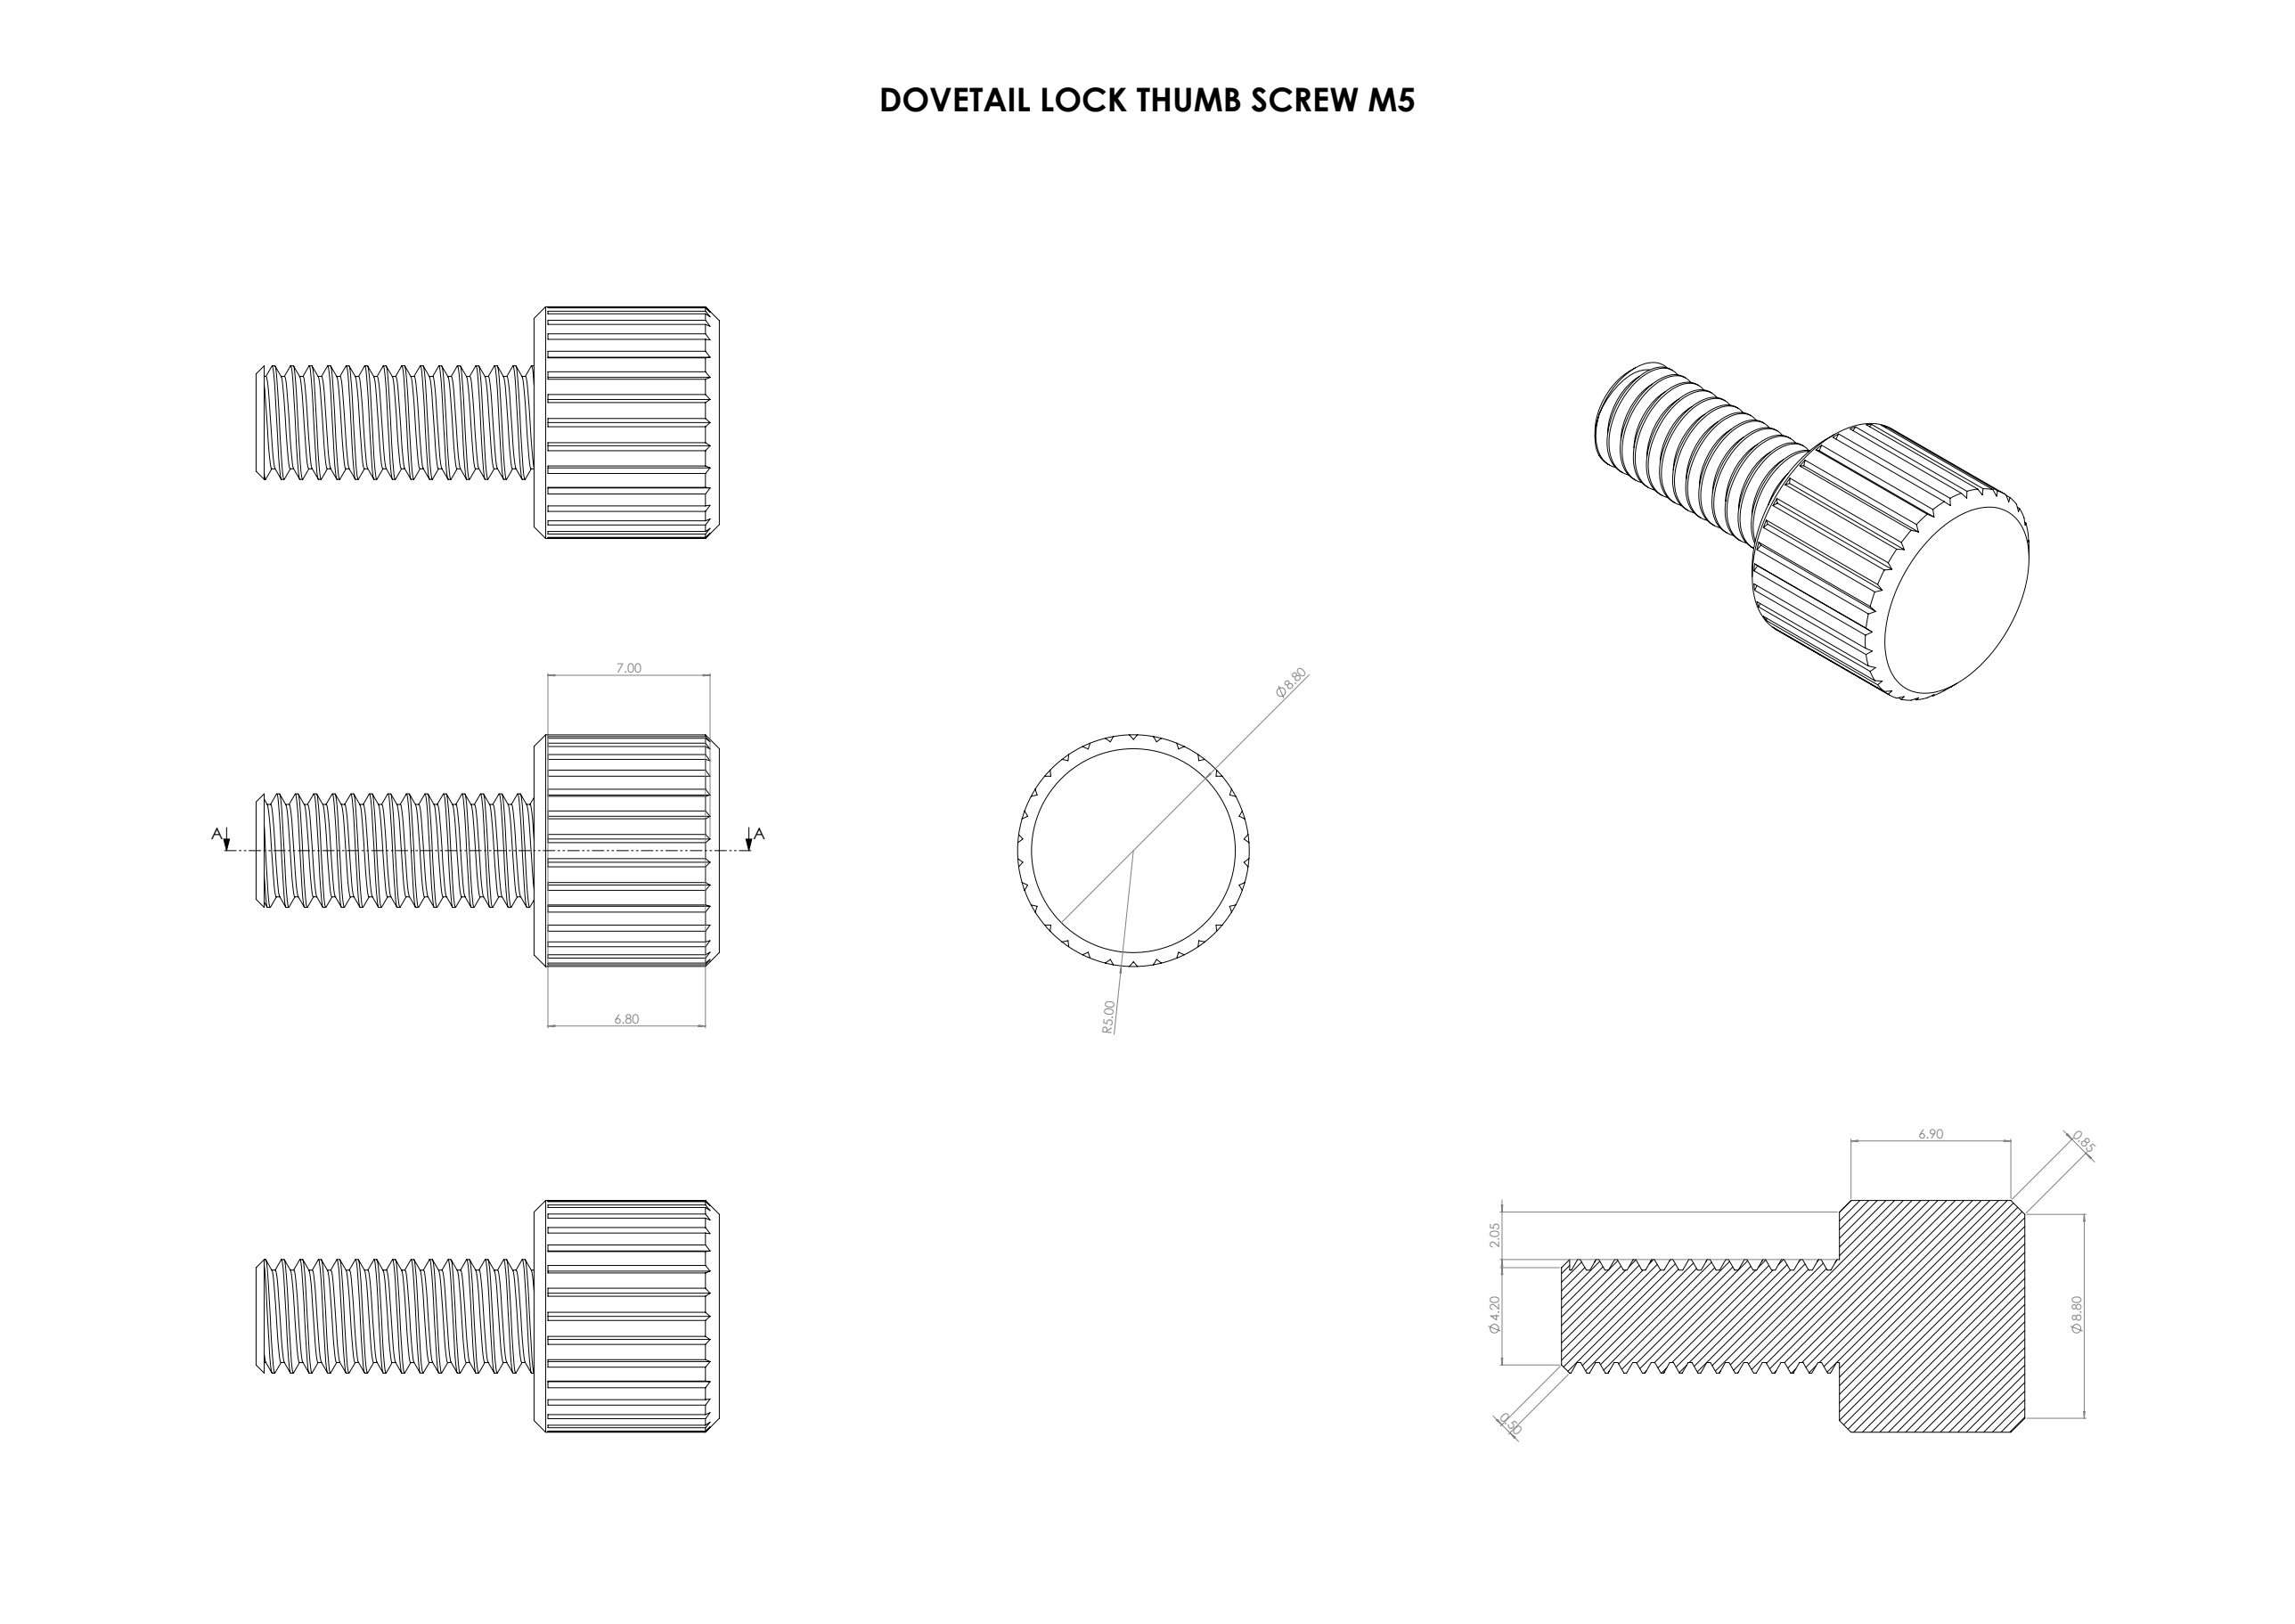
ISO-10303-21;
HEADER;
/* Generated by software containing ST-Developer
 * from STEP Tools, Inc. (www.steptools.com) 
 */

FILE_DESCRIPTION(
/* description */ (''),
/* implementation_level */ '2;1');

FILE_NAME(
/* name */ '12_Dovetail_Lock_Thumb_Screw_M5.step',
/* time_stamp */ '2026-10-21T02:03:06-07:00',
/* author */ (''),
/* organization */ (''),
/* preprocessor_version */ 'ST-DEVELOPER v20.2',
/* originating_system */ 'Autodesk Translation Framework v15.15.0.0',
/* authorisation */ '');

FILE_SCHEMA (('AUTOMOTIVE_DESIGN { 1 0 10303 214 3 1 1 }'));
ENDSEC;

DATA;
#10=MECHANICAL_DESIGN_GEOMETRIC_PRESENTATION_REPRESENTATION('',(#126),#38528);
#89=B_SPLINE_SURFACE_WITH_KNOTS('',3,3,((#36636,#36637,#36638,#36639,#36640,
#36641,#36642,#36643,#36644,#36645,#36646,#36647,#36648,#36649,#36650,#36651,
#36652,#36653,#36654,#36655,#36656,#36657,#36658,#36659,#36660,#36661,#36662,
#36663,#36664,#36665,#36666,#36667,#36668,#36669,#36670,#36671,#36672,#36673,
#36674,#36675,#36676,#36677,#36678,#36679,#36680,#36681,#36682,#36683,#36684,
#36685,#36686,#36687,#36688,#36689,#36690,#36691,#36692,#36693,#36694,#36695,
#36696,#36697,#36698,#36699,#36700,#36701,#36702,#36703,#36704,#36705,#36706,
#36707,#36708,#36709,#36710,#36711,#36712,#36713,#36714,#36715,#36716,#36717,
#36718,#36719,#36720,#36721,#36722,#36723,#36724,#36725,#36726,#36727,#36728,
#36729,#36730,#36731,#36732),(#36733,#36734,#36735,#36736,#36737,#36738,
#36739,#36740,#36741,#36742,#36743,#36744,#36745,#36746,#36747,#36748,#36749,
#36750,#36751,#36752,#36753,#36754,#36755,#36756,#36757,#36758,#36759,#36760,
#36761,#36762,#36763,#36764,#36765,#36766,#36767,#36768,#36769,#36770,#36771,
#36772,#36773,#36774,#36775,#36776,#36777,#36778,#36779,#36780,#36781,#36782,
#36783,#36784,#36785,#36786,#36787,#36788,#36789,#36790,#36791,#36792,#36793,
#36794,#36795,#36796,#36797,#36798,#36799,#36800,#36801,#36802,#36803,#36804,
#36805,#36806,#36807,#36808,#36809,#36810,#36811,#36812,#36813,#36814,#36815,
#36816,#36817,#36818,#36819,#36820,#36821,#36822,#36823,#36824,#36825,#36826,
#36827,#36828,#36829),(#36830,#36831,#36832,#36833,#36834,#36835,#36836,
#36837,#36838,#36839,#36840,#36841,#36842,#36843,#36844,#36845,#36846,#36847,
#36848,#36849,#36850,#36851,#36852,#36853,#36854,#36855,#36856,#36857,#36858,
#36859,#36860,#36861,#36862,#36863,#36864,#36865,#36866,#36867,#36868,#36869,
#36870,#36871,#36872,#36873,#36874,#36875,#36876,#36877,#36878,#36879,#36880,
#36881,#36882,#36883,#36884,#36885,#36886,#36887,#36888,#36889,#36890,#36891,
#36892,#36893,#36894,#36895,#36896,#36897,#36898,#36899,#36900,#36901,#36902,
#36903,#36904,#36905,#36906,#36907,#36908,#36909,#36910,#36911,#36912,#36913,
#36914,#36915,#36916,#36917,#36918,#36919,#36920,#36921,#36922,#36923,#36924,
#36925,#36926),(#36927,#36928,#36929,#36930,#36931,#36932,#36933,#36934,
#36935,#36936,#36937,#36938,#36939,#36940,#36941,#36942,#36943,#36944,#36945,
#36946,#36947,#36948,#36949,#36950,#36951,#36952,#36953,#36954,#36955,#36956,
#36957,#36958,#36959,#36960,#36961,#36962,#36963,#36964,#36965,#36966,#36967,
#36968,#36969,#36970,#36971,#36972,#36973,#36974,#36975,#36976,#36977,#36978,
#36979,#36980,#36981,#36982,#36983,#36984,#36985,#36986,#36987,#36988,#36989,
#36990,#36991,#36992,#36993,#36994,#36995,#36996,#36997,#36998,#36999,#37000,
#37001,#37002,#37003,#37004,#37005,#37006,#37007,#37008,#37009,#37010,#37011,
#37012,#37013,#37014,#37015,#37016,#37017,#37018,#37019,#37020,#37021,#37022,
#37023)),.UNSPECIFIED.,.F.,.F.,.F.,(4,4),(4,1,1,1,1,1,1,1,1,1,1,1,1,1,1,
1,1,1,1,1,1,1,1,1,1,1,1,1,1,1,1,1,1,1,1,1,1,1,1,1,1,1,1,1,1,1,1,1,1,1,1,
1,1,1,1,1,1,1,1,1,1,1,1,1,1,1,1,1,1,1,1,1,1,1,1,1,1,1,1,1,1,1,1,1,1,1,1,
1,1,1,1,1,1,1,4),(0.,0.0526254770366343),(8.30815772716261,9.30349343669038,
10.2988291462181,11.2941648557459,12.2895005652737,13.2848362748014,14.2801719843292,
15.275507693857,16.2708434033847,17.2661791129125,18.2615148224403,19.256850531968,
20.2521862414958,21.2475219510236,22.2428576605513,23.2381933700791,24.2335290796069,
25.2288647891346,26.2242004986624,27.2195362081902,28.2148719177179,29.2102076272457,
30.2055433367735,31.2008790463012,32.196214755829,33.1915504653568,34.1868861748845,
35.1822218844123,36.1775575939401,37.1728933034678,38.1682290129956,39.1635647225234,
40.1589004320511,41.1542361415789,42.1495718511067,43.1449075606344,44.1402432701622,
45.13557897969,46.1309146892177,47.1262503987455,48.1215861082733,49.116921817801,
50.1122575273288,51.1075932368566,52.1029289463843,53.0982646559121,54.0936003654399,
55.0889360749676,56.0842717844954,57.0796074940232,58.0749432035509,59.0702789130787,
60.0656146226065,61.0609503321342,62.056286041662,63.0516217511898,64.0469574607175,
65.0422931702453,66.0376288797731,67.0329645893008,68.0283002988286,69.0236360083564,
70.0189717178841,71.0143074274119,72.0096431369397,73.0049788464674,74.0003145559952,
74.995650265523,75.9909859750507,76.9863216845785,77.9816573941063,78.976993103634,
79.9723288131618,80.9676645226896,81.9630002322173,82.9583359417451,83.9536716512729,
84.9490073608006,85.9443430703284,86.9396787798562,87.9350144893839,88.9303501989117,
89.9256859084395,90.9210216179672,91.916357327495,92.9116930370228,93.9070287465505,
94.9023644560783,95.8977001656061,96.8930358751338,97.8883715846616,98.8837072941894,
99.8790430037171,100.874378713245,101.869714422773),.UNSPECIFIED.);
#90=B_SPLINE_SURFACE_WITH_KNOTS('',3,3,((#37321,#37322,#37323,#37324,#37325,
#37326,#37327,#37328,#37329,#37330,#37331,#37332,#37333,#37334,#37335,#37336,
#37337,#37338,#37339,#37340,#37341,#37342,#37343,#37344,#37345,#37346,#37347,
#37348,#37349,#37350,#37351,#37352,#37353,#37354,#37355,#37356,#37357,#37358,
#37359,#37360,#37361,#37362,#37363,#37364,#37365,#37366,#37367,#37368,#37369,
#37370,#37371,#37372,#37373,#37374,#37375,#37376,#37377,#37378,#37379,#37380,
#37381,#37382,#37383,#37384,#37385,#37386,#37387,#37388,#37389,#37390,#37391,
#37392,#37393,#37394,#37395,#37396,#37397,#37398,#37399,#37400,#37401,#37402,
#37403,#37404,#37405,#37406,#37407,#37408,#37409,#37410,#37411,#37412,#37413,
#37414,#37415,#37416,#37417),(#37418,#37419,#37420,#37421,#37422,#37423,
#37424,#37425,#37426,#37427,#37428,#37429,#37430,#37431,#37432,#37433,#37434,
#37435,#37436,#37437,#37438,#37439,#37440,#37441,#37442,#37443,#37444,#37445,
#37446,#37447,#37448,#37449,#37450,#37451,#37452,#37453,#37454,#37455,#37456,
#37457,#37458,#37459,#37460,#37461,#37462,#37463,#37464,#37465,#37466,#37467,
#37468,#37469,#37470,#37471,#37472,#37473,#37474,#37475,#37476,#37477,#37478,
#37479,#37480,#37481,#37482,#37483,#37484,#37485,#37486,#37487,#37488,#37489,
#37490,#37491,#37492,#37493,#37494,#37495,#37496,#37497,#37498,#37499,#37500,
#37501,#37502,#37503,#37504,#37505,#37506,#37507,#37508,#37509,#37510,#37511,
#37512,#37513,#37514),(#37515,#37516,#37517,#37518,#37519,#37520,#37521,
#37522,#37523,#37524,#37525,#37526,#37527,#37528,#37529,#37530,#37531,#37532,
#37533,#37534,#37535,#37536,#37537,#37538,#37539,#37540,#37541,#37542,#37543,
#37544,#37545,#37546,#37547,#37548,#37549,#37550,#37551,#37552,#37553,#37554,
#37555,#37556,#37557,#37558,#37559,#37560,#37561,#37562,#37563,#37564,#37565,
#37566,#37567,#37568,#37569,#37570,#37571,#37572,#37573,#37574,#37575,#37576,
#37577,#37578,#37579,#37580,#37581,#37582,#37583,#37584,#37585,#37586,#37587,
#37588,#37589,#37590,#37591,#37592,#37593,#37594,#37595,#37596,#37597,#37598,
#37599,#37600,#37601,#37602,#37603,#37604,#37605,#37606,#37607,#37608,#37609,
#37610,#37611),(#37612,#37613,#37614,#37615,#37616,#37617,#37618,#37619,
#37620,#37621,#37622,#37623,#37624,#37625,#37626,#37627,#37628,#37629,#37630,
#37631,#37632,#37633,#37634,#37635,#37636,#37637,#37638,#37639,#37640,#37641,
#37642,#37643,#37644,#37645,#37646,#37647,#37648,#37649,#37650,#37651,#37652,
#37653,#37654,#37655,#37656,#37657,#37658,#37659,#37660,#37661,#37662,#37663,
#37664,#37665,#37666,#37667,#37668,#37669,#37670,#37671,#37672,#37673,#37674,
#37675,#37676,#37677,#37678,#37679,#37680,#37681,#37682,#37683,#37684,#37685,
#37686,#37687,#37688,#37689,#37690,#37691,#37692,#37693,#37694,#37695,#37696,
#37697,#37698,#37699,#37700,#37701,#37702,#37703,#37704,#37705,#37706,#37707,
#37708)),.UNSPECIFIED.,.F.,.F.,.F.,(4,4),(4,1,1,1,1,1,1,1,1,1,1,1,1,1,1,
1,1,1,1,1,1,1,1,1,1,1,1,1,1,1,1,1,1,1,1,1,1,1,1,1,1,1,1,1,1,1,1,1,1,1,1,
1,1,1,1,1,1,1,1,1,1,1,1,1,1,1,1,1,1,1,1,1,1,1,1,1,1,1,1,1,1,1,1,1,1,1,1,
1,1,1,1,1,1,1,4),(0.,0.0526254770366343),(11.6163931973414,12.6117289068692,
13.6070646163969,14.6024003259247,15.5977360354525,16.5930717449802,17.588407454508,
18.5837431640358,19.5790788735635,20.5744145830913,21.5697502926191,22.5650860021468,
23.5604217116746,24.5557574212024,25.5510931307301,26.5464288402579,27.5417645497857,
28.5371002593134,29.5324359688412,30.527771678369,31.5231073878967,32.5184430974245,
33.5137788069523,34.50911451648,35.5044502260078,36.4997859355356,37.4951216450633,
38.4904573545911,39.4857930641189,40.4811287736466,41.4764644831744,42.4718001927022,
43.4671359022299,44.4624716117577,45.4578073212855,46.4531430308133,47.448478740341,
48.4438144498688,49.4391501593965,50.4344858689243,51.4298215784521,52.4251572879798,
53.4204929975076,54.4158287070354,55.4111644165631,56.4065001260909,57.4018358356187,
58.3971715451464,59.3925072546742,60.387842964202,61.3831786737297,62.3785143832575,
63.3738500927853,64.369185802313,65.3645215118408,66.3598572213686,67.3551929308963,
68.3505286404241,69.3458643499519,70.3412000594796,71.3365357690074,72.3318714785352,
73.3272071880629,74.3225428975907,75.3178786071185,76.3132143166462,77.308550026174,
78.3038857357018,79.2992214452295,80.2945571547573,81.2898928642851,82.2852285738128,
83.2805642833406,84.2758999928684,85.2712357023961,86.2665714119239,87.2619071214517,
88.2572428309794,89.2525785405072,90.247914250035,91.2432499595627,92.2385856690905,
93.2339213786183,94.229257088146,95.2245927976738,96.2199285072016,97.2152642167293,
98.2105999262571,99.2059356357849,100.201271345313,101.19660705484,102.191942764368,
103.187278473896,104.182614183424,105.177949892951),.UNSPECIFIED.);
#102=SHAPE_REPRESENTATION_RELATIONSHIP('SRR','None',#38587,#114);
#114=ADVANCED_BREP_SHAPE_REPRESENTATION('',(#138),#38527);
#126=STYLED_ITEM('',(#38713),#138);
#138=MANIFOLD_SOLID_BREP('Body1',#17083);
#396=CYLINDRICAL_SURFACE('',#18809,2.4505);
#397=CYLINDRICAL_SURFACE('',#18811,2.4505);
#398=CYLINDRICAL_SURFACE('',#18812,2.4505);
#399=CYLINDRICAL_SURFACE('',#18813,2.4505);
#400=CYLINDRICAL_SURFACE('',#18814,2.4505);
#401=CYLINDRICAL_SURFACE('',#18815,2.4505);
#402=CYLINDRICAL_SURFACE('',#18816,2.4505);
#403=CYLINDRICAL_SURFACE('',#18817,2.4505);
#404=CYLINDRICAL_SURFACE('',#18818,2.4505);
#405=CYLINDRICAL_SURFACE('',#18819,2.4505);
#406=CYLINDRICAL_SURFACE('',#18820,2.4505);
#407=CYLINDRICAL_SURFACE('',#18821,2.4505);
#408=CYLINDRICAL_SURFACE('',#18822,2.4505);
#409=CYLINDRICAL_SURFACE('',#18823,2.4505);
#410=CYLINDRICAL_SURFACE('',#18824,2.4505);
#411=CYLINDRICAL_SURFACE('',#18825,1.99475);
#412=CYLINDRICAL_SURFACE('',#18827,1.99475);
#413=CYLINDRICAL_SURFACE('',#18828,1.99475);
#414=CYLINDRICAL_SURFACE('',#18829,1.99475);
#415=CYLINDRICAL_SURFACE('',#18830,1.99475);
#416=CYLINDRICAL_SURFACE('',#18831,1.99475);
#417=CYLINDRICAL_SURFACE('',#18832,1.99475);
#418=CYLINDRICAL_SURFACE('',#18833,1.99475);
#419=CYLINDRICAL_SURFACE('',#18834,1.99475);
#420=CYLINDRICAL_SURFACE('',#18835,1.99475);
#421=CYLINDRICAL_SURFACE('',#18836,1.99475);
#422=CYLINDRICAL_SURFACE('',#18837,1.99475);
#423=CYLINDRICAL_SURFACE('',#18838,1.99475);
#424=CYLINDRICAL_SURFACE('',#18839,1.99475);
#425=CYLINDRICAL_SURFACE('',#18844,1.99475);
#426=CYLINDRICAL_SURFACE('',#18849,5.);
#427=CYLINDRICAL_SURFACE('',#19001,2.4505);
#781=B_SPLINE_CURVE_WITH_KNOTS('',3,(#35577,#35578,#35579,#35580,#35581,
#35582,#35583,#35584,#35585,#35586),.UNSPECIFIED.,.F.,.F.,(4,3,3,4),(-4.09157007060748,
-3.98134283811107,-2.9860071285833,-2.06659765062437),.UNSPECIFIED.);
#782=B_SPLINE_CURVE_WITH_KNOTS('',3,(#35589,#35590,#35591,#35592,#35593,
#35594,#35595),.UNSPECIFIED.,.F.,.F.,(4,3,4),(0.,0.995335709527768,1.1166202336066),
 .UNSPECIFIED.);
#783=B_SPLINE_CURVE_WITH_KNOTS('',3,(#35600,#35601,#35602,#35603,#35604,
#35605,#35606,#35607,#35608,#35609,#35610,#35611,#35612,#35613,#35614,#35615,
#35616,#35617,#35618,#35619,#35620,#35621),.UNSPECIFIED.,.F.,.F.,(4,3,3,
3,3,3,3,4),(-10.3747553777871,-9.95335709527767,-8.9580213857499,-7.96268567622213,
-6.96734996669437,-5.9720142571666,-4.97667854763883,-4.09157007060748),
 .UNSPECIFIED.);
#784=B_SPLINE_CURVE_WITH_KNOTS('',3,(#35622,#35623,#35624,#35625,#35626,
#35627,#35628,#35629,#35630,#35631,#35632,#35633,#35634,#35635,#35636,#35637,
#35638,#35639,#35640,#35641,#35642,#35643),.UNSPECIFIED.,.F.,.F.,(4,3,3,
3,3,3,3,4),(1.1166202336066,1.99067141905553,2.9860071285833,3.98134283811107,
4.97667854763883,5.9720142571666,6.96734996669436,7.39980554078619),
 .UNSPECIFIED.);
#785=B_SPLINE_CURVE_WITH_KNOTS('',3,(#35648,#35649,#35650,#35651,#35652,
#35653,#35654,#35655,#35656,#35657,#35658,#35659,#35660,#35661,#35662,#35663,
#35664,#35665,#35666,#35667,#35668,#35669),.UNSPECIFIED.,.F.,.F.,(4,3,3,
3,3,3,3,4),(-16.6579406849666,-15.9253713524443,-14.9300356429165,-13.9346999333887,
-12.939364223861,-11.9440285143332,-10.9486928048054,-10.3747553777871),
 .UNSPECIFIED.);
#786=B_SPLINE_CURVE_WITH_KNOTS('',3,(#35670,#35671,#35672,#35673,#35674,
#35675,#35676,#35677,#35678,#35679,#35680,#35681,#35682,#35683,#35684,#35685,
#35686,#35687,#35688,#35689,#35690,#35691),.UNSPECIFIED.,.F.,.F.,(4,3,3,
3,3,3,3,4),(7.39980554078619,7.96268567622213,8.9580213857499,9.95335709527766,
10.9486928048054,11.9440285143332,12.939364223861,13.6829908479658),
 .UNSPECIFIED.);
#787=B_SPLINE_CURVE_WITH_KNOTS('',3,(#35696,#35697,#35698,#35699,#35700,
#35701,#35702,#35703,#35704,#35705,#35706,#35707,#35708,#35709,#35710,#35711,
#35712,#35713,#35714,#35715,#35716,#35717,#35718,#35719,#35720),
 .UNSPECIFIED.,.F.,.F.,(4,3,3,3,3,3,3,3,4),(-22.9411259921462,-22.8927213191386,
-21.8973856096109,-20.9020499000831,-19.9067141905553,-18.9113784810276,
-17.9160427714998,-16.920707061972,-16.6579406849666),.UNSPECIFIED.);
#788=B_SPLINE_CURVE_WITH_KNOTS('',3,(#35721,#35722,#35723,#35724,#35725,
#35726,#35727,#35728,#35729,#35730,#35731,#35732,#35733,#35734,#35735,#35736,
#35737,#35738,#35739,#35740,#35741,#35742,#35743,#35744,#35745),
 .UNSPECIFIED.,.F.,.F.,(4,3,3,3,3,3,3,3,4),(13.6829908479658,13.9346999333887,
14.9300356429165,15.9253713524443,16.920707061972,17.9160427714998,18.9113784810276,
19.9067141905553,19.9661761551454),.UNSPECIFIED.);
#789=B_SPLINE_CURVE_WITH_KNOTS('',3,(#35750,#35751,#35752,#35753,#35754,
#35755,#35756,#35757,#35758,#35759,#35760,#35761,#35762,#35763,#35764,#35765,
#35766,#35767,#35768,#35769,#35770,#35771),.UNSPECIFIED.,.F.,.F.,(4,3,3,
3,3,3,3,4),(-29.2243112993258,-28.8647355763052,-27.8693998667775,-26.8740641572497,
-25.8787284477219,-24.8833927381942,-23.8880570286664,-22.9411259921462),
 .UNSPECIFIED.);
#790=B_SPLINE_CURVE_WITH_KNOTS('',3,(#35772,#35773,#35774,#35775,#35776,
#35777,#35778,#35779,#35780,#35781,#35782,#35783,#35784,#35785,#35786,#35787,
#35788,#35789,#35790,#35791,#35792,#35793),.UNSPECIFIED.,.F.,.F.,(4,3,3,
3,3,3,3,4),(19.9661761551454,20.9020499000831,21.8973856096109,22.8927213191386,
23.8880570286664,24.8833927381942,25.8787284477219,26.2493614623249),
 .UNSPECIFIED.);
#791=B_SPLINE_CURVE_WITH_KNOTS('',3,(#35798,#35799,#35800,#35801,#35802,
#35803,#35804,#35805,#35806,#35807,#35808,#35809,#35810,#35811,#35812,#35813,
#35814,#35815,#35816,#35817,#35818,#35819),.UNSPECIFIED.,.F.,.F.,(4,3,3,
3,3,3,3,4),(-35.5074966065054,-34.8367498334718,-33.8414141239441,-32.8460784144163,
-31.8507427048885,-30.8554069953608,-29.860071285833,-29.2243112993258),
 .UNSPECIFIED.);
#792=B_SPLINE_CURVE_WITH_KNOTS('',3,(#35820,#35821,#35822,#35823,#35824,
#35825,#35826,#35827,#35828,#35829,#35830,#35831,#35832,#35833,#35834,#35835,
#35836,#35837,#35838,#35839,#35840,#35841),.UNSPECIFIED.,.F.,.F.,(4,3,3,
3,3,3,3,4),(26.2493614623249,26.8740641572497,27.8693998667775,28.8647355763052,
29.860071285833,30.8554069953608,31.8507427048885,32.5325467695045),
 .UNSPECIFIED.);
#793=B_SPLINE_CURVE_WITH_KNOTS('',3,(#35846,#35847,#35848,#35849,#35850,
#35851,#35852,#35853,#35854,#35855,#35856,#35857,#35858,#35859,#35860,#35861,
#35862,#35863,#35864,#35865,#35866,#35867),.UNSPECIFIED.,.F.,.F.,(4,3,3,
3,3,3,3,4),(-41.790681913685,-40.8087640906384,-39.8134283811107,-38.8180926715829,
-37.8227569620551,-36.8274212525274,-35.8320855429996,-35.5074966065054),
 .UNSPECIFIED.);
#794=B_SPLINE_CURVE_WITH_KNOTS('',3,(#35868,#35869,#35870,#35871,#35872,
#35873,#35874,#35875,#35876,#35877,#35878,#35879,#35880,#35881,#35882,#35883,
#35884,#35885,#35886,#35887,#35888,#35889),.UNSPECIFIED.,.F.,.F.,(4,3,3,
3,3,3,3,4),(32.5325467695045,32.8460784144163,33.8414141239441,34.8367498334718,
35.8320855429996,36.8274212525274,37.8227569620551,38.8157320766841),
 .UNSPECIFIED.);
#795=B_SPLINE_CURVE_WITH_KNOTS('',3,(#35894,#35895,#35896,#35897,#35898,
#35899,#35900,#35901,#35902,#35903,#35904,#35905,#35906,#35907,#35908,#35909,
#35910,#35911,#35912,#35913,#35914,#35915,#35916,#35917,#35918),
 .UNSPECIFIED.,.F.,.F.,(4,3,3,3,3,3,3,3,4),(-48.0738672208646,-47.7761140573328,
-46.780778347805,-45.7854426382773,-44.7901069287495,-43.7947712192217,
-42.799435509694,-41.8040998001662,-41.790681913685),.UNSPECIFIED.);
#796=B_SPLINE_CURVE_WITH_KNOTS('',3,(#35919,#35920,#35921,#35922,#35923,
#35924,#35925,#35926,#35927,#35928,#35929,#35930,#35931,#35932,#35933,#35934,
#35935,#35936,#35937,#35938,#35939,#35940,#35941,#35942,#35943),
 .UNSPECIFIED.,.F.,.F.,(4,3,3,3,3,3,3,3,4),(38.8157320766841,38.8180926715829,
39.8134283811107,40.8087640906384,41.8040998001662,42.799435509694,43.7947712192217,
44.7901069287495,45.0989173838637),.UNSPECIFIED.);
#797=B_SPLINE_CURVE_WITH_KNOTS('',3,(#35948,#35949,#35950,#35951,#35952,
#35953,#35954,#35955,#35956,#35957,#35958,#35959,#35960,#35961,#35962,#35963,
#35964,#35965,#35966,#35967,#35968,#35969),.UNSPECIFIED.,.F.,.F.,(4,3,3,
3,3,3,3,4),(-54.3570525280442,-53.7481283144994,-52.7527926049716,-51.7574568954439,
-50.7621211859161,-49.7667854763883,-48.7714497668606,-48.0738672208646),
 .UNSPECIFIED.);
#798=B_SPLINE_CURVE_WITH_KNOTS('',3,(#35970,#35971,#35972,#35973,#35974,
#35975,#35976,#35977,#35978,#35979,#35980,#35981,#35982,#35983,#35984,#35985,
#35986,#35987,#35988,#35989,#35990,#35991),.UNSPECIFIED.,.F.,.F.,(4,3,3,
3,3,3,3,4),(45.0989173838637,45.7854426382773,46.780778347805,47.7761140573328,
48.7714497668606,49.7667854763883,50.7621211859161,51.3821026910433),
 .UNSPECIFIED.);
#799=B_SPLINE_CURVE_WITH_KNOTS('',3,(#35996,#35997,#35998,#35999,#36000,
#36001,#36002,#36003,#36004,#36005,#36006,#36007,#36008,#36009,#36010,#36011,
#36012,#36013,#36014,#36015,#36016,#36017),.UNSPECIFIED.,.F.,.F.,(4,3,3,
3,3,3,3,4),(-60.6402378352238,-59.720142571666,-58.7248068621382,-57.7294711526105,
-56.7341354430827,-55.7387997335549,-54.7434640240272,-54.3570525280442),
 .UNSPECIFIED.);
#800=B_SPLINE_CURVE_WITH_KNOTS('',3,(#36018,#36019,#36020,#36021,#36022,
#36023,#36024,#36025,#36026,#36027,#36028,#36029,#36030,#36031,#36032,#36033,
#36034,#36035,#36036,#36037,#36038,#36039),.UNSPECIFIED.,.F.,.F.,(4,3,3,
3,3,3,3,4),(51.3821026910433,51.7574568954439,52.7527926049716,53.7481283144994,
54.7434640240272,55.7387997335549,56.7341354430827,57.6652879982229),
 .UNSPECIFIED.);
#801=B_SPLINE_CURVE_WITH_KNOTS('',3,(#36044,#36045,#36046,#36047,#36048,
#36049,#36050,#36051,#36052,#36053,#36054,#36055,#36056,#36057,#36058,#36059,
#36060,#36061,#36062,#36063,#36064,#36065,#36066,#36067,#36068),
 .UNSPECIFIED.,.F.,.F.,(4,3,3,3,3,3,3,3,4),(-66.9234231424034,-66.6874925383604,
-65.6921568288326,-64.6968211193048,-63.7014854097771,-62.7061497002493,
-61.7108139907215,-60.7154782811938,-60.6402378352238),.UNSPECIFIED.);
#802=B_SPLINE_CURVE_WITH_KNOTS('',3,(#36069,#36070,#36071,#36072,#36073,
#36074,#36075,#36076,#36077,#36078,#36079,#36080,#36081,#36082,#36083,#36084,
#36085,#36086,#36087,#36088,#36089,#36090,#36091,#36092,#36093),
 .UNSPECIFIED.,.F.,.F.,(4,3,3,3,3,3,3,3,4),(57.6652879982229,57.7294711526105,
58.7248068621382,59.720142571666,60.7154782811938,61.7108139907215,62.7061497002493,
63.7014854097771,63.9484733054025),.UNSPECIFIED.);
#803=B_SPLINE_CURVE_WITH_KNOTS('',3,(#36098,#36099,#36100,#36101,#36102,
#36103,#36104,#36105,#36106,#36107,#36108,#36109,#36110,#36111,#36112,#36113,
#36114,#36115,#36116,#36117,#36118,#36119),.UNSPECIFIED.,.F.,.F.,(4,3,3,
3,3,3,3,4),(-73.206608449583,-72.659506795527,-71.6641710859992,-70.6688353764714,
-69.6734996669437,-68.6781639574159,-67.6828282478881,-66.9234231424034),
 .UNSPECIFIED.);
#804=B_SPLINE_CURVE_WITH_KNOTS('',3,(#36120,#36121,#36122,#36123,#36124,
#36125,#36126,#36127,#36128,#36129,#36130,#36131,#36132,#36133,#36134,#36135,
#36136,#36137,#36138,#36139,#36140,#36141),.UNSPECIFIED.,.F.,.F.,(4,3,3,
3,3,3,3,4),(63.9484733054025,64.6968211193048,65.6921568288326,66.6874925383604,
67.6828282478881,68.6781639574159,69.6734996669437,70.2316586125821),
 .UNSPECIFIED.);
#805=B_SPLINE_CURVE_WITH_KNOTS('',3,(#36146,#36147,#36148,#36149,#36150,
#36151,#36152,#36153,#36154,#36155,#36156,#36157,#36158,#36159,#36160,#36161,
#36162,#36163,#36164,#36165,#36166,#36167),.UNSPECIFIED.,.F.,.F.,(4,3,3,
3,3,3,3,4),(-79.4897937567626,-78.6315210526936,-77.6361853431658,-76.640849633638,
-75.6455139241102,-74.6501782145825,-73.6548425050547,-73.206608449583),
 .UNSPECIFIED.);
#806=B_SPLINE_CURVE_WITH_KNOTS('',3,(#36168,#36169,#36170,#36171,#36172,
#36173,#36174,#36175,#36176,#36177,#36178,#36179,#36180,#36181,#36182,#36183,
#36184,#36185,#36186,#36187,#36188,#36189),.UNSPECIFIED.,.F.,.F.,(4,3,3,
3,3,3,3,4),(70.2316586125821,70.6688353764714,71.6641710859992,72.659506795527,
73.6548425050547,74.6501782145825,75.6455139241103,76.5148439197617),
 .UNSPECIFIED.);
#807=B_SPLINE_CURVE_WITH_KNOTS('',3,(#36194,#36195,#36196,#36197,#36198,
#36199,#36200,#36201,#36202,#36203,#36204,#36205,#36206,#36207,#36208,#36209,
#36210,#36211,#36212,#36213,#36214,#36215,#36216,#36217,#36218),
 .UNSPECIFIED.,.F.,.F.,(4,3,3,3,3,3,3,3,4),(-85.7729790639422,-85.5988710193879,
-84.6035353098602,-83.6081996003324,-82.6128638908046,-81.6175281812769,
-80.6221924717491,-79.6268567622213,-79.4897937567626),.UNSPECIFIED.);
#808=B_SPLINE_CURVE_WITH_KNOTS('',3,(#36219,#36220,#36221,#36222,#36223,
#36224,#36225,#36226,#36227,#36228,#36229,#36230,#36231,#36232,#36233,#36234,
#36235,#36236,#36237,#36238,#36239,#36240,#36241,#36242,#36243),
 .UNSPECIFIED.,.F.,.F.,(4,3,3,3,3,3,3,3,4),(76.5148439197617,76.640849633638,
77.6361853431658,78.6315210526936,79.6268567622213,80.6221924717491,81.6175281812769,
82.6128638908046,82.7980292269413),.UNSPECIFIED.);
#809=B_SPLINE_CURVE_WITH_KNOTS('',3,(#36248,#36249,#36250,#36251,#36252,
#36253,#36254,#36255,#36256,#36257,#36258,#36259,#36260,#36261,#36262,#36263,
#36264,#36265,#36266,#36267,#36268,#36269),.UNSPECIFIED.,.F.,.F.,(4,3,3,
3,3,3,3,4),(-92.0561643711218,-91.5708852765545,-90.5755495670268,-89.580213857499,
-88.5848781479712,-87.5895424384435,-86.5942067289157,-85.7729790639422),
 .UNSPECIFIED.);
#810=B_SPLINE_CURVE_WITH_KNOTS('',3,(#36270,#36271,#36272,#36273,#36274,
#36275,#36276,#36277,#36278,#36279,#36280,#36281,#36282,#36283,#36284,#36285,
#36286,#36287,#36288,#36289,#36290,#36291),.UNSPECIFIED.,.F.,.F.,(4,3,3,
3,3,3,3,4),(82.7980292269413,83.6081996003324,84.6035353098601,85.5988710193879,
86.5942067289157,87.5895424384435,88.5848781479712,89.0812145341209),
 .UNSPECIFIED.);
#811=B_SPLINE_CURVE_WITH_KNOTS('',3,(#36297,#36298,#36299,#36300,#36301,
#36302,#36303,#36304,#36305),.UNSPECIFIED.,.F.,.F.,(4,1,1,1,1,1,4),(97.3893722612836,
98.2105999262571,99.2059356357849,100.201271345313,101.19660705484,102.191942764368,
103.111352242327),.UNSPECIFIED.);
#812=B_SPLINE_CURVE_WITH_KNOTS('',3,(#36308,#36309,#36310,#36311,#36312,
#36313,#36314,#36315),.UNSPECIFIED.,.F.,.F.,(4,1,1,1,1,4),(97.3893722612836,
97.8883715846616,98.8837072941894,99.8790430037171,100.874378713245,101.869714422773),
 .UNSPECIFIED.);
#813=B_SPLINE_CURVE_WITH_KNOTS('',3,(#36320,#36321,#36322,#36323,#36324,
#36325,#36326,#36327,#36328,#36329,#36330),.UNSPECIFIED.,.F.,.F.,(4,1,1,
1,1,1,1,1,4),(91.106186954104,91.2432499595627,92.2385856690905,93.2339213786183,
94.229257088146,95.2245927976738,96.2199285072016,97.2152642167293,97.3893722612836),
 .UNSPECIFIED.);
#814=B_SPLINE_CURVE_WITH_KNOTS('',3,(#36331,#36332,#36333,#36334,#36335,
#36336,#36337,#36338,#36339,#36340),.UNSPECIFIED.,.F.,.F.,(4,1,1,1,1,1,
1,4),(91.106186954104,91.916357327495,92.9116930370228,93.9070287465505,
94.9023644560783,95.8977001656061,96.8930358751338,97.3893722612836),
 .UNSPECIFIED.);
#815=B_SPLINE_CURVE_WITH_KNOTS('',3,(#36345,#36346,#36347,#36348,#36349,
#36350,#36351,#36352,#36353,#36354),.UNSPECIFIED.,.F.,.F.,(4,1,1,1,1,1,
1,4),(84.8230016469244,85.2712357023961,86.2665714119239,87.2619071214517,
88.2572428309794,89.2525785405072,90.247914250035,91.106186954104),
 .UNSPECIFIED.);
#816=B_SPLINE_CURVE_WITH_KNOTS('',3,(#36355,#36356,#36357,#36358,#36359,
#36360,#36361,#36362,#36363,#36364,#36365),.UNSPECIFIED.,.F.,.F.,(4,1,1,
1,1,1,1,1,4),(84.8230016469244,84.9490073608006,85.9443430703284,86.9396787798562,
87.9350144893839,88.9303501989117,89.9256859084395,90.9210216179672,91.106186954104),
 .UNSPECIFIED.);
#817=B_SPLINE_CURVE_WITH_KNOTS('',3,(#36370,#36371,#36372,#36373,#36374,
#36375,#36376,#36377,#36378,#36379),.UNSPECIFIED.,.F.,.F.,(4,1,1,1,1,1,
1,4),(78.5398163397448,79.2992214452295,80.2945571547573,81.2898928642851,
82.2852285738128,83.2805642833406,84.2758999928684,84.8230016469244),
 .UNSPECIFIED.);
#818=B_SPLINE_CURVE_WITH_KNOTS('',3,(#36380,#36381,#36382,#36383,#36384,
#36385,#36386,#36387,#36388,#36389),.UNSPECIFIED.,.F.,.F.,(4,1,1,1,1,1,
1,4),(78.5398163397448,78.976993103634,79.9723288131618,80.9676645226896,
81.9630002322173,82.9583359417451,83.9536716512729,84.8230016469244),
 .UNSPECIFIED.);
#819=B_SPLINE_CURVE_WITH_KNOTS('',3,(#36394,#36395,#36396,#36397,#36398,
#36399,#36400,#36401,#36402,#36403,#36404),.UNSPECIFIED.,.F.,.F.,(4,1,1,
1,1,1,1,1,4),(72.2566310325652,72.3318714785352,73.3272071880629,74.3225428975907,
75.3178786071185,76.3132143166462,77.308550026174,78.3038857357018,78.5398163397448),
 .UNSPECIFIED.);
#820=B_SPLINE_CURVE_WITH_KNOTS('',3,(#36405,#36406,#36407,#36408,#36409,
#36410,#36411,#36412,#36413,#36414),.UNSPECIFIED.,.F.,.F.,(4,1,1,1,1,1,
1,4),(72.2566310325652,73.0049788464674,74.0003145559952,74.995650265523,
75.9909859750507,76.9863216845785,77.9816573941063,78.5398163397448),
 .UNSPECIFIED.);
#821=B_SPLINE_CURVE_WITH_KNOTS('',3,(#36419,#36420,#36421,#36422,#36423,
#36424,#36425,#36426,#36427,#36428),.UNSPECIFIED.,.F.,.F.,(4,1,1,1,1,1,
1,4),(65.9734457253856,66.3598572213686,67.3551929308963,68.3505286404241,
69.3458643499519,70.3412000594796,71.3365357690074,72.2566310325652),
 .UNSPECIFIED.);
#822=B_SPLINE_CURVE_WITH_KNOTS('',3,(#36429,#36430,#36431,#36432,#36433,
#36434,#36435,#36436,#36437,#36438,#36439),.UNSPECIFIED.,.F.,.F.,(4,1,1,
1,1,1,1,1,4),(65.9734457253856,66.0376288797731,67.0329645893008,68.0283002988286,
69.0236360083564,70.0189717178841,71.0143074274119,72.0096431369397,72.2566310325652),
 .UNSPECIFIED.);
#823=B_SPLINE_CURVE_WITH_KNOTS('',3,(#36444,#36445,#36446,#36447,#36448,
#36449,#36450,#36451,#36452,#36453),.UNSPECIFIED.,.F.,.F.,(4,1,1,1,1,1,
1,4),(59.690260418206,60.387842964202,61.3831786737297,62.3785143832575,
63.3738500927853,64.369185802313,65.3645215118408,65.9734457253856),
 .UNSPECIFIED.);
#824=B_SPLINE_CURVE_WITH_KNOTS('',3,(#36454,#36455,#36456,#36457,#36458,
#36459,#36460,#36461,#36462,#36463),.UNSPECIFIED.,.F.,.F.,(4,1,1,1,1,1,
1,4),(59.690260418206,60.0656146226065,61.0609503321342,62.056286041662,
63.0516217511898,64.0469574607175,65.0422931702453,65.9734457253856),
 .UNSPECIFIED.);
#825=B_SPLINE_CURVE_WITH_KNOTS('',3,(#36468,#36469,#36470,#36471,#36472,
#36473,#36474,#36475,#36476,#36477,#36478),.UNSPECIFIED.,.F.,.F.,(4,1,1,
1,1,1,1,1,4),(53.4070751110264,53.4204929975076,54.4158287070354,55.4111644165631,
56.4065001260909,57.4018358356187,58.3971715451464,59.3925072546742,59.690260418206),
 .UNSPECIFIED.);
#826=B_SPLINE_CURVE_WITH_KNOTS('',3,(#36479,#36480,#36481,#36482,#36483,
#36484,#36485,#36486,#36487,#36488),.UNSPECIFIED.,.F.,.F.,(4,1,1,1,1,1,
1,4),(53.4070751110264,54.0936003654399,55.0889360749676,56.0842717844954,
57.0796074940232,58.0749432035509,59.0702789130787,59.690260418206),
 .UNSPECIFIED.);
#827=B_SPLINE_CURVE_WITH_KNOTS('',3,(#36493,#36494,#36495,#36496,#36497,
#36498,#36499,#36500,#36501,#36502),.UNSPECIFIED.,.F.,.F.,(4,1,1,1,1,1,
1,4),(47.1238898038469,47.448478740341,48.4438144498688,49.4391501593965,
50.4344858689243,51.4298215784521,52.4251572879798,53.4070751110264),
 .UNSPECIFIED.);
#828=B_SPLINE_CURVE_WITH_KNOTS('',3,(#36503,#36504,#36505,#36506,#36507,
#36508,#36509,#36510,#36511,#36512,#36513),.UNSPECIFIED.,.F.,.F.,(4,1,1,
1,1,1,1,1,4),(47.1238898038468,47.1262503987455,48.1215861082733,49.116921817801,
50.1122575273288,51.1075932368566,52.1029289463843,53.0982646559121,53.4070751110264),
 .UNSPECIFIED.);
#829=B_SPLINE_CURVE_WITH_KNOTS('',3,(#36518,#36519,#36520,#36521,#36522,
#36523,#36524,#36525,#36526,#36527),.UNSPECIFIED.,.F.,.F.,(4,1,1,1,1,1,
1,4),(40.8407044966673,41.4764644831744,42.4718001927022,43.4671359022299,
44.4624716117577,45.4578073212855,46.4531430308133,47.1238898038469),
 .UNSPECIFIED.);
#830=B_SPLINE_CURVE_WITH_KNOTS('',3,(#36528,#36529,#36530,#36531,#36532,
#36533,#36534,#36535,#36536,#36537),.UNSPECIFIED.,.F.,.F.,(4,1,1,1,1,1,
1,4),(40.8407044966672,41.1542361415789,42.1495718511067,43.1449075606344,
44.1402432701622,45.13557897969,46.1309146892177,47.1238898038468),
 .UNSPECIFIED.);
#831=B_SPLINE_CURVE_WITH_KNOTS('',3,(#36542,#36543,#36544,#36545,#36546,
#36547,#36548,#36549,#36550,#36551),.UNSPECIFIED.,.F.,.F.,(4,1,1,1,1,1,
1,4),(34.5575191894877,35.5044502260078,36.4997859355356,37.4951216450633,
38.4904573545911,39.4857930641189,40.4811287736466,40.8407044966673),
 .UNSPECIFIED.);
#832=B_SPLINE_CURVE_WITH_KNOTS('',3,(#36552,#36553,#36554,#36555,#36556,
#36557,#36558,#36559,#36560,#36561),.UNSPECIFIED.,.F.,.F.,(4,1,1,1,1,1,
1,4),(34.5575191894876,35.1822218844123,36.1775575939401,37.1728933034678,
38.1682290129956,39.1635647225234,40.1589004320511,40.8407044966672),
 .UNSPECIFIED.);
#833=B_SPLINE_CURVE_WITH_KNOTS('',3,(#36566,#36567,#36568,#36569,#36570,
#36571,#36572,#36573,#36574,#36575,#36576),.UNSPECIFIED.,.F.,.F.,(4,1,1,
1,1,1,1,1,4),(28.2743338823081,28.5371002593134,29.5324359688412,30.527771678369,
31.5231073878967,32.5184430974245,33.5137788069523,34.50911451648,34.5575191894877),
 .UNSPECIFIED.);
#834=B_SPLINE_CURVE_WITH_KNOTS('',3,(#36577,#36578,#36579,#36580,#36581,
#36582,#36583,#36584,#36585,#36586),.UNSPECIFIED.,.F.,.F.,(4,1,1,1,1,1,
1,4),(28.2743338823081,29.2102076272457,30.2055433367735,31.2008790463012,
32.196214755829,33.1915504653568,34.1868861748845,34.5575191894876),
 .UNSPECIFIED.);
#835=B_SPLINE_CURVE_WITH_KNOTS('',3,(#36591,#36592,#36593,#36594,#36595,
#36596,#36597,#36598,#36599,#36600),.UNSPECIFIED.,.F.,.F.,(4,1,1,1,1,1,
1,4),(21.9911485751285,22.5650860021468,23.5604217116746,24.5557574212024,
25.5510931307301,26.5464288402579,27.5417645497857,28.2743338823081),
 .UNSPECIFIED.);
#836=B_SPLINE_CURVE_WITH_KNOTS('',3,(#36601,#36602,#36603,#36604,#36605,
#36606,#36607,#36608,#36609,#36610,#36611),.UNSPECIFIED.,.F.,.F.,(4,1,1,
1,1,1,1,1,4),(21.9911485751285,22.2428576605513,23.2381933700791,24.2335290796069,
25.2288647891346,26.2242004986624,27.2195362081902,28.2148719177179,28.2743338823081),
 .UNSPECIFIED.);
#837=B_SPLINE_CURVE_WITH_KNOTS('',3,(#36616,#36617,#36618,#36619,#36620,
#36621,#36622,#36623,#36624,#36625),.UNSPECIFIED.,.F.,.F.,(4,1,1,1,1,1,
1,4),(15.7079632679489,16.5930717449802,17.588407454508,18.5837431640358,
19.5790788735635,20.5744145830913,21.5697502926191,21.9911485751285),
 .UNSPECIFIED.);
#838=B_SPLINE_CURVE_WITH_KNOTS('',3,(#36626,#36627,#36628,#36629,#36630,
#36631,#36632,#36633,#36634,#36635),.UNSPECIFIED.,.F.,.F.,(4,1,1,1,1,1,
1,4),(15.7079632679489,16.2708434033847,17.2661791129125,18.2615148224403,
19.256850531968,20.2521862414958,21.2475219510236,21.9911485751285),
 .UNSPECIFIED.);
#839=B_SPLINE_CURVE_WITH_KNOTS('',3,(#37025,#37026,#37027,#37028,#37029,
#37030,#37031,#37032,#37033,#37034,#37035,#37036,#37037,#37038,#37039,#37040,
#37041,#37042,#37043,#37044,#37045,#37046,#37047,#37048,#37049,#37050,#37051,
#37052,#37053,#37054,#37055,#37056,#37057,#37058,#37059,#37060,#37061,#37062,
#37063,#37064,#37065,#37066,#37067,#37068,#37069,#37070,#37071,#37072,#37073,
#37074,#37075,#37076,#37077,#37078,#37079,#37080,#37081,#37082,#37083,#37084,
#37085,#37086,#37087,#37088,#37089,#37090,#37091,#37092,#37093,#37094,#37095,
#37096,#37097,#37098,#37099,#37100,#37101,#37102,#37103,#37104,#37105,#37106,
#37107,#37108,#37109,#37110,#37111,#37112),.UNSPECIFIED.,.F.,.F.,(4,3,3,
3,3,3,3,3,3,3,3,3,3,3,3,3,3,3,3,3,3,3,3,3,3,3,3,3,3,4),(-0.461788964899778,
-0.4432234502138,-0.417585071690447,-0.404676823606039,-0.398380133623887,
-0.393259612278708,-0.367874849545492,-0.348272131144797,-0.338456418860554,
-0.332916476029383,-0.308151864898805,-0.283877174259086,-0.260161043087549,
-0.251332965374558,-0.246977223747103,-0.243306514944723,-0.219829616972232,
-0.211053102339927,-0.187088418858572,-0.163702366501251,-0.158787258719064,
-0.135433187942531,-0.112095172587591,-0.0891454130303583,-0.0803315821691377,
-0.0766175667602699,-0.0541537505784823,-0.0320531226257585,-0.0106595864360154,
0.),.UNSPECIFIED.);
#840=B_SPLINE_CURVE_WITH_KNOTS('',3,(#37113,#37114,#37115,#37116,#37117,
#37118,#37119,#37120,#37121,#37122),.UNSPECIFIED.,.F.,.F.,(4,3,3,4),(89.0812145341209,
89.580213857499,90.5755495670267,91.4949590449857),.UNSPECIFIED.);
#841=B_SPLINE_CURVE_WITH_KNOTS('',3,(#37124,#37125,#37126,#37127,#37128,
#37129,#37130,#37131,#37132,#37133,#37134,#37135,#37136,#37137,#37138,#37139,
#37140,#37141,#37142,#37143,#37144,#37145,#37146,#37147,#37148,#37149,#37150,
#37151,#37152,#37153,#37154,#37155,#37156,#37157,#37158,#37159,#37160,#37161,
#37162,#37163,#37164,#37165,#37166,#37167,#37168,#37169,#37170,#37171,#37172,
#37173,#37174,#37175,#37176,#37177,#37178,#37179,#37180,#37181,#37182,#37183,
#37184,#37185,#37186,#37187,#37188,#37189,#37190,#37191,#37192,#37193,#37194,
#37195,#37196,#37197,#37198,#37199,#37200,#37201,#37202,#37203,#37204,#37205,
#37206,#37207,#37208),.UNSPECIFIED.,.F.,.F.,(4,3,3,3,3,3,3,3,3,3,3,3,3,
3,3,3,3,3,3,3,3,3,3,3,3,3,3,3,4),(-0.463803050843711,-0.448429413206914,
-0.426704171981601,-0.414159993364273,-0.409718066359999,-0.387136470680841,
-0.368120384440548,-0.35895595361815,-0.354767190879561,-0.331504579574296,
-0.307380379870345,-0.289287230092382,-0.275717367758909,-0.271450226768227,
-0.267796738492813,-0.243369230116364,-0.235007780758492,-0.211413020390669,
-0.187330446081715,-0.181489281437917,-0.157060938111767,-0.132145865675509,
-0.107037279266715,-0.0963831544778031,-0.0910163492829886,-0.0652783368980751,
-0.0394980984327342,-0.0142604401573251,0.),.UNSPECIFIED.);
#842=B_SPLINE_CURVE_WITH_KNOTS('',3,(#37209,#37210,#37211,#37212,#37213,
#37214,#37215,#37216,#37217),.UNSPECIFIED.,.F.,.F.,(4,1,1,1,1,1,4),(10.374755377787,
11.2941648557459,12.2895005652737,13.2848362748014,14.2801719843292,15.275507693857,
15.7079632679489),.UNSPECIFIED.);
#843=B_SPLINE_CURVE_WITH_KNOTS('',3,(#37223,#37224,#37225,#37226,#37227,
#37228,#37229,#37230,#37231,#37232,#37233,#37234,#37235,#37236,#37237,#37238,
#37239,#37240,#37241,#37242,#37243,#37244,#37245,#37246,#37247,#37248,#37249,
#37250,#37251,#37252,#37253,#37254,#37255,#37256,#37257,#37258,#37259,#37260,
#37261,#37262,#37263,#37264,#37265,#37266,#37267,#37268,#37269,#37270,#37271,
#37272,#37273,#37274,#37275,#37276,#37277,#37278,#37279,#37280,#37281,#37282,
#37283,#37284,#37285,#37286,#37287,#37288,#37289,#37290,#37291,#37292,#37293,
#37294,#37295,#37296,#37297,#37298,#37299,#37300,#37301,#37302,#37303,#37304,
#37305,#37306,#37307,#37308,#37309,#37310),.UNSPECIFIED.,.F.,.F.,(4,3,3,
3,3,3,3,3,3,3,3,3,3,3,3,3,3,3,3,3,3,3,3,3,3,3,3,3,3,4),(-0.461788964899765,
-0.443223450213792,-0.417585071143145,-0.404676823092943,-0.398380110287486,
-0.393259604558869,-0.367874841639472,-0.348272124227028,-0.338456405730752,
-0.332916474245839,-0.308151862176156,-0.283877172217097,-0.260161025980822,
-0.251332920274659,-0.246977167765169,-0.243306502630573,-0.219829594194119,
-0.211053102339921,-0.187088411880509,-0.163702360395445,-0.158787259103022,
-0.135433184446935,-0.112095174888583,-0.0891454298609094,-0.0803315842997371,
-0.0766175679727495,-0.0541537625388748,-0.0320531510297545,-0.010659635642814,
0.),.UNSPECIFIED.);
#844=B_SPLINE_CURVE_WITH_KNOTS('',3,(#37313,#37314,#37315,#37316,#37317,
#37318,#37319,#37320),.UNSPECIFIED.,.F.,.F.,(4,1,1,1,1,4),(11.6163931973414,
12.6117289068692,13.6070646163969,14.6024003259247,15.5977360354525,15.7079632679489),
 .UNSPECIFIED.);
#845=B_SPLINE_CURVE_WITH_KNOTS('',3,(#37710,#37711,#37712,#37713,#37714,
#37715,#37716,#37717,#37718,#37719,#37720,#37721,#37722,#37723,#37724,#37725,
#37726,#37727,#37728,#37729,#37730,#37731,#37732,#37733,#37734,#37735,#37736,
#37737,#37738,#37739,#37740,#37741,#37742,#37743,#37744,#37745,#37746,#37747,
#37748,#37749,#37750,#37751,#37752,#37753,#37754,#37755,#37756,#37757,#37758,
#37759,#37760,#37761,#37762,#37763,#37764,#37765,#37766,#37767,#37768,#37769,
#37770,#37771,#37772,#37773,#37774,#37775,#37776,#37777,#37778,#37779,#37780,
#37781,#37782,#37783,#37784,#37785,#37786,#37787,#37788,#37789,#37790,#37791,
#37792,#37793,#37794),.UNSPECIFIED.,.F.,.F.,(4,3,3,3,3,3,3,3,3,3,3,3,3,
3,3,3,3,3,3,3,3,3,3,3,3,3,3,3,4),(-0.463803050843705,-0.448429413206907,
-0.42670415944794,-0.4141599708977,-0.409718048450771,-0.387136443589144,
-0.368120360735312,-0.358955917726794,-0.354767147726934,-0.331504528371831,
-0.307380341468495,-0.289287201290993,-0.275717346157866,-0.271450058108256,
-0.267796704376614,-0.243369196611869,-0.235007780758486,-0.211413015229316,
-0.187330434823406,-0.181489285380682,-0.157060936178603,-0.132145857977694,
-0.107037270590661,-0.0963831412843047,-0.0910163503959406,-0.0652783344338678,
-0.0394980989815758,-0.0142604566308707,0.),.UNSPECIFIED.);
#846=B_SPLINE_CURVE_WITH_KNOTS('',3,(#37795,#37796,#37797,#37798,#37799,
#37800,#37801),.UNSPECIFIED.,.F.,.F.,(4,3,4),(-93.5615566956101,-92.5662209860823,
-92.0561643711218),.UNSPECIFIED.);
#1048=CONICAL_SURFACE('',#19000,2.3,0.785398163397448);
#1049=CONICAL_SURFACE('',#19005,4.75,0.785398163397448);
#1050=CONICAL_SURFACE('',#19006,4.7,0.785398163397447);
#1364=(
BOUNDED_CURVE()
B_SPLINE_CURVE(2,(#37805,#37806,#37807),.UNSPECIFIED.,.F.,.F.)
B_SPLINE_CURVE_WITH_KNOTS((3,3),(0.,0.0331882448287731),.UNSPECIFIED.)
CURVE()
GEOMETRIC_REPRESENTATION_ITEM()
RATIONAL_B_SPLINE_CURVE((1.,1.00036538368932,1.))
REPRESENTATION_ITEM('')
);
#1365=(
BOUNDED_CURVE()
B_SPLINE_CURVE(2,(#37819,#37820,#37821),.UNSPECIFIED.,.F.,.F.)
B_SPLINE_CURVE_WITH_KNOTS((3,3),(0.,0.0331882448287731),.UNSPECIFIED.)
CURVE()
GEOMETRIC_REPRESENTATION_ITEM()
RATIONAL_B_SPLINE_CURVE((1.,1.00036538368669,1.))
REPRESENTATION_ITEM('')
);
#1366=(
BOUNDED_CURVE()
B_SPLINE_CURVE(2,(#38064,#38065,#38066),.UNSPECIFIED.,.F.,.F.)
B_SPLINE_CURVE_WITH_KNOTS((3,3),(0.,0.033188244828773),.UNSPECIFIED.)
CURVE()
GEOMETRIC_REPRESENTATION_ITEM()
RATIONAL_B_SPLINE_CURVE((1.,1.00036538369005,1.))
REPRESENTATION_ITEM('')
);
#1367=(
BOUNDED_CURVE()
B_SPLINE_CURVE(2,(#38073,#38074,#38075),.UNSPECIFIED.,.F.,.F.)
B_SPLINE_CURVE_WITH_KNOTS((3,3),(0.,0.0331882448287731),.UNSPECIFIED.)
CURVE()
GEOMETRIC_REPRESENTATION_ITEM()
RATIONAL_B_SPLINE_CURVE((1.,1.00036538368877,1.))
REPRESENTATION_ITEM('')
);
#1368=(
BOUNDED_CURVE()
B_SPLINE_CURVE(2,(#38078,#38079,#38080),.UNSPECIFIED.,.F.,.F.)
B_SPLINE_CURVE_WITH_KNOTS((3,3),(0.,0.0331882448287731),.UNSPECIFIED.)
CURVE()
GEOMETRIC_REPRESENTATION_ITEM()
RATIONAL_B_SPLINE_CURVE((1.,1.00036538368768,1.))
REPRESENTATION_ITEM('')
);
#1369=(
BOUNDED_CURVE()
B_SPLINE_CURVE(2,(#38087,#38088,#38089),.UNSPECIFIED.,.F.,.F.)
B_SPLINE_CURVE_WITH_KNOTS((3,3),(0.,0.0331882448287732),.UNSPECIFIED.)
CURVE()
GEOMETRIC_REPRESENTATION_ITEM()
RATIONAL_B_SPLINE_CURVE((1.,1.00036538368663,1.))
REPRESENTATION_ITEM('')
);
#1370=(
BOUNDED_CURVE()
B_SPLINE_CURVE(2,(#38092,#38093,#38094),.UNSPECIFIED.,.F.,.F.)
B_SPLINE_CURVE_WITH_KNOTS((3,3),(0.,0.033188244828773),.UNSPECIFIED.)
CURVE()
GEOMETRIC_REPRESENTATION_ITEM()
RATIONAL_B_SPLINE_CURVE((1.,1.0003653836895,1.))
REPRESENTATION_ITEM('')
);
#1371=(
BOUNDED_CURVE()
B_SPLINE_CURVE(2,(#38101,#38102,#38103),.UNSPECIFIED.,.F.,.F.)
B_SPLINE_CURVE_WITH_KNOTS((3,3),(0.,0.0331882448287732),.UNSPECIFIED.)
CURVE()
GEOMETRIC_REPRESENTATION_ITEM()
RATIONAL_B_SPLINE_CURVE((1.,1.0003653836875,1.))
REPRESENTATION_ITEM('')
);
#1372=(
BOUNDED_CURVE()
B_SPLINE_CURVE(2,(#38106,#38107,#38108),.UNSPECIFIED.,.F.,.F.)
B_SPLINE_CURVE_WITH_KNOTS((3,3),(0.,0.0331882448287729),.UNSPECIFIED.)
CURVE()
GEOMETRIC_REPRESENTATION_ITEM()
RATIONAL_B_SPLINE_CURVE((1.,1.00036538368829,1.))
REPRESENTATION_ITEM('')
);
#1373=(
BOUNDED_CURVE()
B_SPLINE_CURVE(2,(#38115,#38116,#38117),.UNSPECIFIED.,.F.,.F.)
B_SPLINE_CURVE_WITH_KNOTS((3,3),(0.,0.0331882448287728),.UNSPECIFIED.)
CURVE()
GEOMETRIC_REPRESENTATION_ITEM()
RATIONAL_B_SPLINE_CURVE((1.,1.00036538369157,1.))
REPRESENTATION_ITEM('')
);
#1374=(
BOUNDED_CURVE()
B_SPLINE_CURVE(2,(#38120,#38121,#38122),.UNSPECIFIED.,.F.,.F.)
B_SPLINE_CURVE_WITH_KNOTS((3,3),(0.,0.0331882448287729),.UNSPECIFIED.)
CURVE()
GEOMETRIC_REPRESENTATION_ITEM()
RATIONAL_B_SPLINE_CURVE((1.,1.00036538368829,1.))
REPRESENTATION_ITEM('')
);
#1375=(
BOUNDED_CURVE()
B_SPLINE_CURVE(2,(#38129,#38130,#38131),.UNSPECIFIED.,.F.,.F.)
B_SPLINE_CURVE_WITH_KNOTS((3,3),(0.,0.0331882448287729),.UNSPECIFIED.)
CURVE()
GEOMETRIC_REPRESENTATION_ITEM()
RATIONAL_B_SPLINE_CURVE((1.,1.00036538368924,1.))
REPRESENTATION_ITEM('')
);
#1376=(
BOUNDED_CURVE()
B_SPLINE_CURVE(2,(#38134,#38135,#38136),.UNSPECIFIED.,.F.,.F.)
B_SPLINE_CURVE_WITH_KNOTS((3,3),(0.,0.033188244828773),.UNSPECIFIED.)
CURVE()
GEOMETRIC_REPRESENTATION_ITEM()
RATIONAL_B_SPLINE_CURVE((1.,1.0003653836883,1.))
REPRESENTATION_ITEM('')
);
#1377=(
BOUNDED_CURVE()
B_SPLINE_CURVE(2,(#38143,#38144,#38145),.UNSPECIFIED.,.F.,.F.)
B_SPLINE_CURVE_WITH_KNOTS((3,3),(0.,0.033188244828773),.UNSPECIFIED.)
CURVE()
GEOMETRIC_REPRESENTATION_ITEM()
RATIONAL_B_SPLINE_CURVE((1.,1.00036538368856,1.))
REPRESENTATION_ITEM('')
);
#1378=(
BOUNDED_CURVE()
B_SPLINE_CURVE(2,(#38148,#38149,#38150),.UNSPECIFIED.,.F.,.F.)
B_SPLINE_CURVE_WITH_KNOTS((3,3),(0.,0.0331882448287729),.UNSPECIFIED.)
CURVE()
GEOMETRIC_REPRESENTATION_ITEM()
RATIONAL_B_SPLINE_CURVE((1.,1.000365383688,1.))
REPRESENTATION_ITEM('')
);
#1379=(
BOUNDED_CURVE()
B_SPLINE_CURVE(2,(#38157,#38158,#38159),.UNSPECIFIED.,.F.,.F.)
B_SPLINE_CURVE_WITH_KNOTS((3,3),(0.,0.0331882448287729),.UNSPECIFIED.)
CURVE()
GEOMETRIC_REPRESENTATION_ITEM()
RATIONAL_B_SPLINE_CURVE((1.,1.00036538369129,1.))
REPRESENTATION_ITEM('')
);
#1380=(
BOUNDED_CURVE()
B_SPLINE_CURVE(2,(#38162,#38163,#38164),.UNSPECIFIED.,.F.,.F.)
B_SPLINE_CURVE_WITH_KNOTS((3,3),(0.,0.033188244828773),.UNSPECIFIED.)
CURVE()
GEOMETRIC_REPRESENTATION_ITEM()
RATIONAL_B_SPLINE_CURVE((1.,1.00036538369007,1.))
REPRESENTATION_ITEM('')
);
#1381=(
BOUNDED_CURVE()
B_SPLINE_CURVE(2,(#38171,#38172,#38173),.UNSPECIFIED.,.F.,.F.)
B_SPLINE_CURVE_WITH_KNOTS((3,3),(0.,0.0331882448287728),.UNSPECIFIED.)
CURVE()
GEOMETRIC_REPRESENTATION_ITEM()
RATIONAL_B_SPLINE_CURVE((1.,1.00036538369054,1.))
REPRESENTATION_ITEM('')
);
#1382=(
BOUNDED_CURVE()
B_SPLINE_CURVE(2,(#38176,#38177,#38178),.UNSPECIFIED.,.F.,.F.)
B_SPLINE_CURVE_WITH_KNOTS((3,3),(0.,0.0331882448287728),.UNSPECIFIED.)
CURVE()
GEOMETRIC_REPRESENTATION_ITEM()
RATIONAL_B_SPLINE_CURVE((1.,1.00036538369027,1.))
REPRESENTATION_ITEM('')
);
#1383=(
BOUNDED_CURVE()
B_SPLINE_CURVE(2,(#38185,#38186,#38187),.UNSPECIFIED.,.F.,.F.)
B_SPLINE_CURVE_WITH_KNOTS((3,3),(0.,0.033188244828773),.UNSPECIFIED.)
CURVE()
GEOMETRIC_REPRESENTATION_ITEM()
RATIONAL_B_SPLINE_CURVE((1.,1.00036538369294,1.))
REPRESENTATION_ITEM('')
);
#1384=(
BOUNDED_CURVE()
B_SPLINE_CURVE(2,(#38190,#38191,#38192),.UNSPECIFIED.,.F.,.F.)
B_SPLINE_CURVE_WITH_KNOTS((3,3),(0.,0.0331882448287729),.UNSPECIFIED.)
CURVE()
GEOMETRIC_REPRESENTATION_ITEM()
RATIONAL_B_SPLINE_CURVE((1.,1.00036538369069,1.))
REPRESENTATION_ITEM('')
);
#1385=(
BOUNDED_CURVE()
B_SPLINE_CURVE(2,(#38199,#38200,#38201),.UNSPECIFIED.,.F.,.F.)
B_SPLINE_CURVE_WITH_KNOTS((3,3),(0.,0.0331882448287729),.UNSPECIFIED.)
CURVE()
GEOMETRIC_REPRESENTATION_ITEM()
RATIONAL_B_SPLINE_CURVE((1.,1.00036538369006,1.))
REPRESENTATION_ITEM('')
);
#1386=(
BOUNDED_CURVE()
B_SPLINE_CURVE(2,(#38204,#38205,#38206),.UNSPECIFIED.,.F.,.F.)
B_SPLINE_CURVE_WITH_KNOTS((3,3),(0.,0.0331882448287728),.UNSPECIFIED.)
CURVE()
GEOMETRIC_REPRESENTATION_ITEM()
RATIONAL_B_SPLINE_CURVE((1.,1.00036538369315,1.))
REPRESENTATION_ITEM('')
);
#1387=(
BOUNDED_CURVE()
B_SPLINE_CURVE(2,(#38213,#38214,#38215),.UNSPECIFIED.,.F.,.F.)
B_SPLINE_CURVE_WITH_KNOTS((3,3),(0.,0.0331882448287729),.UNSPECIFIED.)
CURVE()
GEOMETRIC_REPRESENTATION_ITEM()
RATIONAL_B_SPLINE_CURVE((1.,1.00036538368966,1.))
REPRESENTATION_ITEM('')
);
#1388=(
BOUNDED_CURVE()
B_SPLINE_CURVE(2,(#38218,#38219,#38220),.UNSPECIFIED.,.F.,.F.)
B_SPLINE_CURVE_WITH_KNOTS((3,3),(0.,0.0331882448287729),.UNSPECIFIED.)
CURVE()
GEOMETRIC_REPRESENTATION_ITEM()
RATIONAL_B_SPLINE_CURVE((1.,1.00036538369197,1.))
REPRESENTATION_ITEM('')
);
#1389=(
BOUNDED_CURVE()
B_SPLINE_CURVE(2,(#38227,#38228,#38229),.UNSPECIFIED.,.F.,.F.)
B_SPLINE_CURVE_WITH_KNOTS((3,3),(0.,0.0331882448287729),.UNSPECIFIED.)
CURVE()
GEOMETRIC_REPRESENTATION_ITEM()
RATIONAL_B_SPLINE_CURVE((1.,1.00036538368905,1.))
REPRESENTATION_ITEM('')
);
#1390=(
BOUNDED_CURVE()
B_SPLINE_CURVE(2,(#38232,#38233,#38234),.UNSPECIFIED.,.F.,.F.)
B_SPLINE_CURVE_WITH_KNOTS((3,3),(0.,0.033188244828773),.UNSPECIFIED.)
CURVE()
GEOMETRIC_REPRESENTATION_ITEM()
RATIONAL_B_SPLINE_CURVE((1.,1.0003653836867,1.))
REPRESENTATION_ITEM('')
);
#1391=(
BOUNDED_CURVE()
B_SPLINE_CURVE(2,(#38241,#38242,#38243),.UNSPECIFIED.,.F.,.F.)
B_SPLINE_CURVE_WITH_KNOTS((3,3),(0.,0.0331882448287729),.UNSPECIFIED.)
CURVE()
GEOMETRIC_REPRESENTATION_ITEM()
RATIONAL_B_SPLINE_CURVE((1.,1.00036538369137,1.))
REPRESENTATION_ITEM('')
);
#1392=(
BOUNDED_CURVE()
B_SPLINE_CURVE(2,(#38246,#38247,#38248),.UNSPECIFIED.,.F.,.F.)
B_SPLINE_CURVE_WITH_KNOTS((3,3),(0.,0.033188244828773),.UNSPECIFIED.)
CURVE()
GEOMETRIC_REPRESENTATION_ITEM()
RATIONAL_B_SPLINE_CURVE((1.,1.0003653836899,1.))
REPRESENTATION_ITEM('')
);
#1393=(
BOUNDED_CURVE()
B_SPLINE_CURVE(2,(#38255,#38256,#38257),.UNSPECIFIED.,.F.,.F.)
B_SPLINE_CURVE_WITH_KNOTS((3,3),(0.,0.033188244828773),.UNSPECIFIED.)
CURVE()
GEOMETRIC_REPRESENTATION_ITEM()
RATIONAL_B_SPLINE_CURVE((1.,1.00036538369,1.))
REPRESENTATION_ITEM('')
);
#1394=(
BOUNDED_CURVE()
B_SPLINE_CURVE(2,(#38260,#38261,#38262),.UNSPECIFIED.,.F.,.F.)
B_SPLINE_CURVE_WITH_KNOTS((3,3),(0.,0.0331882448287729),.UNSPECIFIED.)
CURVE()
GEOMETRIC_REPRESENTATION_ITEM()
RATIONAL_B_SPLINE_CURVE((1.,1.00036538369195,1.))
REPRESENTATION_ITEM('')
);
#1395=(
BOUNDED_CURVE()
B_SPLINE_CURVE(2,(#38269,#38270,#38271),.UNSPECIFIED.,.F.,.F.)
B_SPLINE_CURVE_WITH_KNOTS((3,3),(0.,0.033188244828773),.UNSPECIFIED.)
CURVE()
GEOMETRIC_REPRESENTATION_ITEM()
RATIONAL_B_SPLINE_CURVE((1.,1.00036538369028,1.))
REPRESENTATION_ITEM('')
);
#1396=(
BOUNDED_CURVE()
B_SPLINE_CURVE(2,(#38274,#38275,#38276),.UNSPECIFIED.,.F.,.F.)
B_SPLINE_CURVE_WITH_KNOTS((3,3),(0.,0.0331882448287728),.UNSPECIFIED.)
CURVE()
GEOMETRIC_REPRESENTATION_ITEM()
RATIONAL_B_SPLINE_CURVE((1.,1.00036538369196,1.))
REPRESENTATION_ITEM('')
);
#1397=(
BOUNDED_CURVE()
B_SPLINE_CURVE(2,(#38283,#38284,#38285),.UNSPECIFIED.,.F.,.F.)
B_SPLINE_CURVE_WITH_KNOTS((3,3),(0.,0.0331882448287729),.UNSPECIFIED.)
CURVE()
GEOMETRIC_REPRESENTATION_ITEM()
RATIONAL_B_SPLINE_CURVE((1.,1.00036538369028,1.))
REPRESENTATION_ITEM('')
);
#1398=(
BOUNDED_CURVE()
B_SPLINE_CURVE(2,(#38288,#38289,#38290),.UNSPECIFIED.,.F.,.F.)
B_SPLINE_CURVE_WITH_KNOTS((3,3),(0.,0.0331882448287729),.UNSPECIFIED.)
CURVE()
GEOMETRIC_REPRESENTATION_ITEM()
RATIONAL_B_SPLINE_CURVE((1.,1.00036538369004,1.))
REPRESENTATION_ITEM('')
);
#1399=(
BOUNDED_CURVE()
B_SPLINE_CURVE(2,(#38297,#38298,#38299),.UNSPECIFIED.,.F.,.F.)
B_SPLINE_CURVE_WITH_KNOTS((3,3),(0.,0.033188244828773),.UNSPECIFIED.)
CURVE()
GEOMETRIC_REPRESENTATION_ITEM()
RATIONAL_B_SPLINE_CURVE((1.,1.00036538368968,1.))
REPRESENTATION_ITEM('')
);
#1400=(
BOUNDED_CURVE()
B_SPLINE_CURVE(2,(#38302,#38303,#38304),.UNSPECIFIED.,.F.,.F.)
B_SPLINE_CURVE_WITH_KNOTS((3,3),(0.,0.0331882448287729),.UNSPECIFIED.)
CURVE()
GEOMETRIC_REPRESENTATION_ITEM()
RATIONAL_B_SPLINE_CURVE((1.,1.0003653836908,1.))
REPRESENTATION_ITEM('')
);
#1401=(
BOUNDED_CURVE()
B_SPLINE_CURVE(2,(#38311,#38312,#38313),.UNSPECIFIED.,.F.,.F.)
B_SPLINE_CURVE_WITH_KNOTS((3,3),(0.,0.0331882448287729),.UNSPECIFIED.)
CURVE()
GEOMETRIC_REPRESENTATION_ITEM()
RATIONAL_B_SPLINE_CURVE((1.,1.00036538369234,1.))
REPRESENTATION_ITEM('')
);
#1402=(
BOUNDED_CURVE()
B_SPLINE_CURVE(2,(#38316,#38317,#38318),.UNSPECIFIED.,.F.,.F.)
B_SPLINE_CURVE_WITH_KNOTS((3,3),(0.,0.033188244828773),.UNSPECIFIED.)
CURVE()
GEOMETRIC_REPRESENTATION_ITEM()
RATIONAL_B_SPLINE_CURVE((1.,1.00036538368982,1.))
REPRESENTATION_ITEM('')
);
#1403=(
BOUNDED_CURVE()
B_SPLINE_CURVE(2,(#38325,#38326,#38327),.UNSPECIFIED.,.F.,.F.)
B_SPLINE_CURVE_WITH_KNOTS((3,3),(0.,0.0331882448287727),.UNSPECIFIED.)
CURVE()
GEOMETRIC_REPRESENTATION_ITEM()
RATIONAL_B_SPLINE_CURVE((1.,1.00036538368872,1.))
REPRESENTATION_ITEM('')
);
#1404=(
BOUNDED_CURVE()
B_SPLINE_CURVE(2,(#38330,#38331,#38332),.UNSPECIFIED.,.F.,.F.)
B_SPLINE_CURVE_WITH_KNOTS((3,3),(0.,0.0331882448287729),.UNSPECIFIED.)
CURVE()
GEOMETRIC_REPRESENTATION_ITEM()
RATIONAL_B_SPLINE_CURVE((1.,1.00036538368741,1.))
REPRESENTATION_ITEM('')
);
#1405=(
BOUNDED_CURVE()
B_SPLINE_CURVE(2,(#38339,#38340,#38341),.UNSPECIFIED.,.F.,.F.)
B_SPLINE_CURVE_WITH_KNOTS((3,3),(0.,0.0331882448287729),.UNSPECIFIED.)
CURVE()
GEOMETRIC_REPRESENTATION_ITEM()
RATIONAL_B_SPLINE_CURVE((1.,1.00036538369134,1.))
REPRESENTATION_ITEM('')
);
#1406=(
BOUNDED_CURVE()
B_SPLINE_CURVE(2,(#38344,#38345,#38346),.UNSPECIFIED.,.F.,.F.)
B_SPLINE_CURVE_WITH_KNOTS((3,3),(0.,0.0331882448287729),.UNSPECIFIED.)
CURVE()
GEOMETRIC_REPRESENTATION_ITEM()
RATIONAL_B_SPLINE_CURVE((1.,1.00036538368855,1.))
REPRESENTATION_ITEM('')
);
#1407=(
BOUNDED_CURVE()
B_SPLINE_CURVE(2,(#38353,#38354,#38355),.UNSPECIFIED.,.F.,.F.)
B_SPLINE_CURVE_WITH_KNOTS((3,3),(0.,0.0331882448287729),.UNSPECIFIED.)
CURVE()
GEOMETRIC_REPRESENTATION_ITEM()
RATIONAL_B_SPLINE_CURVE((1.,1.00036538368991,1.))
REPRESENTATION_ITEM('')
);
#1408=(
BOUNDED_CURVE()
B_SPLINE_CURVE(2,(#38358,#38359,#38360),.UNSPECIFIED.,.F.,.F.)
B_SPLINE_CURVE_WITH_KNOTS((3,3),(0.,0.0331882448287729),.UNSPECIFIED.)
CURVE()
GEOMETRIC_REPRESENTATION_ITEM()
RATIONAL_B_SPLINE_CURVE((1.,1.00036538369097,1.))
REPRESENTATION_ITEM('')
);
#1409=(
BOUNDED_CURVE()
B_SPLINE_CURVE(2,(#38367,#38368,#38369),.UNSPECIFIED.,.F.,.F.)
B_SPLINE_CURVE_WITH_KNOTS((3,3),(0.,0.0331882448287729),.UNSPECIFIED.)
CURVE()
GEOMETRIC_REPRESENTATION_ITEM()
RATIONAL_B_SPLINE_CURVE((1.,1.00036538369135,1.))
REPRESENTATION_ITEM('')
);
#1410=(
BOUNDED_CURVE()
B_SPLINE_CURVE(2,(#38372,#38373,#38374),.UNSPECIFIED.,.F.,.F.)
B_SPLINE_CURVE_WITH_KNOTS((3,3),(0.,0.033188244828773),.UNSPECIFIED.)
CURVE()
GEOMETRIC_REPRESENTATION_ITEM()
RATIONAL_B_SPLINE_CURVE((1.,1.00036538369049,1.))
REPRESENTATION_ITEM('')
);
#1411=(
BOUNDED_CURVE()
B_SPLINE_CURVE(2,(#38381,#38382,#38383),.UNSPECIFIED.,.F.,.F.)
B_SPLINE_CURVE_WITH_KNOTS((3,3),(0.,0.033188244828773),.UNSPECIFIED.)
CURVE()
GEOMETRIC_REPRESENTATION_ITEM()
RATIONAL_B_SPLINE_CURVE((1.,1.00036538369154,1.))
REPRESENTATION_ITEM('')
);
#1412=(
BOUNDED_CURVE()
B_SPLINE_CURVE(2,(#38386,#38387,#38388),.UNSPECIFIED.,.F.,.F.)
B_SPLINE_CURVE_WITH_KNOTS((3,3),(0.,0.0331882448287728),.UNSPECIFIED.)
CURVE()
GEOMETRIC_REPRESENTATION_ITEM()
RATIONAL_B_SPLINE_CURVE((1.,1.00036538368967,1.))
REPRESENTATION_ITEM('')
);
#1413=(
BOUNDED_CURVE()
B_SPLINE_CURVE(2,(#38395,#38396,#38397),.UNSPECIFIED.,.F.,.F.)
B_SPLINE_CURVE_WITH_KNOTS((3,3),(0.,0.033188244828773),.UNSPECIFIED.)
CURVE()
GEOMETRIC_REPRESENTATION_ITEM()
RATIONAL_B_SPLINE_CURVE((1.,1.00036538369075,1.))
REPRESENTATION_ITEM('')
);
#1414=(
BOUNDED_CURVE()
B_SPLINE_CURVE(2,(#38400,#38401,#38402),.UNSPECIFIED.,.F.,.F.)
B_SPLINE_CURVE_WITH_KNOTS((3,3),(0.,0.0331882448287729),.UNSPECIFIED.)
CURVE()
GEOMETRIC_REPRESENTATION_ITEM()
RATIONAL_B_SPLINE_CURVE((1.,1.00036538369014,1.))
REPRESENTATION_ITEM('')
);
#1415=(
BOUNDED_CURVE()
B_SPLINE_CURVE(2,(#38409,#38410,#38411),.UNSPECIFIED.,.F.,.F.)
B_SPLINE_CURVE_WITH_KNOTS((3,3),(0.,0.0331882448287729),.UNSPECIFIED.)
CURVE()
GEOMETRIC_REPRESENTATION_ITEM()
RATIONAL_B_SPLINE_CURVE((1.,1.00036538368956,1.))
REPRESENTATION_ITEM('')
);
#1416=(
BOUNDED_CURVE()
B_SPLINE_CURVE(2,(#38414,#38415,#38416),.UNSPECIFIED.,.F.,.F.)
B_SPLINE_CURVE_WITH_KNOTS((3,3),(0.,0.0331882448287729),.UNSPECIFIED.)
CURVE()
GEOMETRIC_REPRESENTATION_ITEM()
RATIONAL_B_SPLINE_CURVE((1.,1.00036538369215,1.))
REPRESENTATION_ITEM('')
);
#1417=(
BOUNDED_CURVE()
B_SPLINE_CURVE(2,(#38423,#38424,#38425),.UNSPECIFIED.,.F.,.F.)
B_SPLINE_CURVE_WITH_KNOTS((3,3),(0.,0.0331882448287728),.UNSPECIFIED.)
CURVE()
GEOMETRIC_REPRESENTATION_ITEM()
RATIONAL_B_SPLINE_CURVE((1.,1.00036538368934,1.))
REPRESENTATION_ITEM('')
);
#1418=(
BOUNDED_CURVE()
B_SPLINE_CURVE(2,(#38428,#38429,#38430),.UNSPECIFIED.,.F.,.F.)
B_SPLINE_CURVE_WITH_KNOTS((3,3),(0.,0.0331882448287729),.UNSPECIFIED.)
CURVE()
GEOMETRIC_REPRESENTATION_ITEM()
RATIONAL_B_SPLINE_CURVE((1.,1.00036538368812,1.))
REPRESENTATION_ITEM('')
);
#1419=(
BOUNDED_CURVE()
B_SPLINE_CURVE(2,(#38437,#38438,#38439),.UNSPECIFIED.,.F.,.F.)
B_SPLINE_CURVE_WITH_KNOTS((3,3),(0.,0.033188244828773),.UNSPECIFIED.)
CURVE()
GEOMETRIC_REPRESENTATION_ITEM()
RATIONAL_B_SPLINE_CURVE((1.,1.00036538368966,1.))
REPRESENTATION_ITEM('')
);
#1420=(
BOUNDED_CURVE()
B_SPLINE_CURVE(2,(#38442,#38443,#38444),.UNSPECIFIED.,.F.,.F.)
B_SPLINE_CURVE_WITH_KNOTS((3,3),(0.,0.033188244828773),.UNSPECIFIED.)
CURVE()
GEOMETRIC_REPRESENTATION_ITEM()
RATIONAL_B_SPLINE_CURVE((1.,1.00036538368713,1.))
REPRESENTATION_ITEM('')
);
#1421=(
BOUNDED_CURVE()
B_SPLINE_CURVE(2,(#38451,#38452,#38453),.UNSPECIFIED.,.F.,.F.)
B_SPLINE_CURVE_WITH_KNOTS((3,3),(0.,0.0331882448287729),.UNSPECIFIED.)
CURVE()
GEOMETRIC_REPRESENTATION_ITEM()
RATIONAL_B_SPLINE_CURVE((1.,1.00036538369046,1.))
REPRESENTATION_ITEM('')
);
#1422=(
BOUNDED_CURVE()
B_SPLINE_CURVE(2,(#38456,#38457,#38458),.UNSPECIFIED.,.F.,.F.)
B_SPLINE_CURVE_WITH_KNOTS((3,3),(0.,0.033188244828773),.UNSPECIFIED.)
CURVE()
GEOMETRIC_REPRESENTATION_ITEM()
RATIONAL_B_SPLINE_CURVE((1.,1.00036538369035,1.))
REPRESENTATION_ITEM('')
);
#1423=(
BOUNDED_CURVE()
B_SPLINE_CURVE(2,(#38465,#38466,#38467),.UNSPECIFIED.,.F.,.F.)
B_SPLINE_CURVE_WITH_KNOTS((3,3),(0.,0.033188244828773),.UNSPECIFIED.)
CURVE()
GEOMETRIC_REPRESENTATION_ITEM()
RATIONAL_B_SPLINE_CURVE((1.,1.00036538369101,1.))
REPRESENTATION_ITEM('')
);
#1476=FACE_BOUND('',#4287,.T.);
#2209=CIRCLE('',#18810,2.4505);
#2210=CIRCLE('',#18826,1.99475);
#2211=CIRCLE('',#18841,2.4505);
#2212=CIRCLE('',#18842,2.4505);
#2213=CIRCLE('',#18843,1.99475);
#2214=CIRCLE('',#18847,5.);
#2215=CIRCLE('',#18850,5.);
#2216=CIRCLE('',#18851,5.);
#2217=CIRCLE('',#18852,5.);
#2218=CIRCLE('',#18853,5.);
#2219=CIRCLE('',#18854,5.);
#2220=CIRCLE('',#18855,5.);
#2221=CIRCLE('',#18856,5.);
#2222=CIRCLE('',#18857,5.);
#2223=CIRCLE('',#18858,5.);
#2224=CIRCLE('',#18859,5.);
#2225=CIRCLE('',#18860,5.);
#2226=CIRCLE('',#18861,5.);
#2227=CIRCLE('',#18862,5.);
#2228=CIRCLE('',#18863,5.);
#2229=CIRCLE('',#18864,5.);
#2230=CIRCLE('',#18865,5.);
#2231=CIRCLE('',#18866,5.);
#2232=CIRCLE('',#18867,5.);
#2233=CIRCLE('',#18868,5.);
#2234=CIRCLE('',#18869,5.);
#2235=CIRCLE('',#18870,5.);
#2236=CIRCLE('',#18871,5.);
#2237=CIRCLE('',#18872,5.);
#2238=CIRCLE('',#18873,5.);
#2239=CIRCLE('',#18874,5.);
#2240=CIRCLE('',#18875,5.);
#2241=CIRCLE('',#18876,5.);
#2242=CIRCLE('',#18877,5.);
#2243=CIRCLE('',#18878,5.);
#2244=CIRCLE('',#18879,5.);
#2245=CIRCLE('',#18880,5.);
#2246=CIRCLE('',#18881,5.);
#2247=CIRCLE('',#18882,5.);
#2248=CIRCLE('',#18883,5.);
#2249=CIRCLE('',#18884,5.);
#2250=CIRCLE('',#18885,5.);
#2251=CIRCLE('',#18886,5.);
#2252=CIRCLE('',#18887,5.);
#2253=CIRCLE('',#18888,5.);
#2254=CIRCLE('',#18889,5.);
#2255=CIRCLE('',#18890,5.);
#2256=CIRCLE('',#18891,5.);
#2257=CIRCLE('',#18892,5.);
#2258=CIRCLE('',#18893,5.);
#2259=CIRCLE('',#18894,5.);
#2260=CIRCLE('',#18895,5.);
#2261=CIRCLE('',#18896,5.);
#2262=CIRCLE('',#18897,5.);
#2263=CIRCLE('',#18898,5.);
#2264=CIRCLE('',#18899,5.);
#2265=CIRCLE('',#18900,5.);
#2266=CIRCLE('',#18901,5.);
#2267=CIRCLE('',#18902,5.);
#2268=CIRCLE('',#18903,5.);
#2269=CIRCLE('',#18904,5.);
#2270=CIRCLE('',#18905,5.);
#2271=CIRCLE('',#18906,5.);
#2272=CIRCLE('',#18907,5.);
#2273=CIRCLE('',#18908,5.);
#2274=CIRCLE('',#18909,5.);
#2275=CIRCLE('',#18910,5.);
#2276=CIRCLE('',#18999,2.1);
#2277=CIRCLE('',#19002,2.4505);
#2278=CIRCLE('',#19004,4.5);
#2279=CIRCLE('',#19007,4.4);
#3132=FACE_OUTER_BOUND('',#4159,.T.);
#3133=FACE_OUTER_BOUND('',#4160,.T.);
#3134=FACE_OUTER_BOUND('',#4161,.T.);
#3135=FACE_OUTER_BOUND('',#4162,.T.);
#3136=FACE_OUTER_BOUND('',#4163,.T.);
#3137=FACE_OUTER_BOUND('',#4164,.T.);
#3138=FACE_OUTER_BOUND('',#4165,.T.);
#3139=FACE_OUTER_BOUND('',#4166,.T.);
#3140=FACE_OUTER_BOUND('',#4167,.T.);
#3141=FACE_OUTER_BOUND('',#4168,.T.);
#3142=FACE_OUTER_BOUND('',#4169,.T.);
#3143=FACE_OUTER_BOUND('',#4170,.T.);
#3144=FACE_OUTER_BOUND('',#4171,.T.);
#3145=FACE_OUTER_BOUND('',#4172,.T.);
#3146=FACE_OUTER_BOUND('',#4173,.T.);
#3147=FACE_OUTER_BOUND('',#4174,.T.);
#3148=FACE_OUTER_BOUND('',#4175,.T.);
#3149=FACE_OUTER_BOUND('',#4176,.T.);
#3150=FACE_OUTER_BOUND('',#4177,.T.);
#3151=FACE_OUTER_BOUND('',#4178,.T.);
#3152=FACE_OUTER_BOUND('',#4179,.T.);
#3153=FACE_OUTER_BOUND('',#4180,.T.);
#3154=FACE_OUTER_BOUND('',#4181,.T.);
#3155=FACE_OUTER_BOUND('',#4182,.T.);
#3156=FACE_OUTER_BOUND('',#4183,.T.);
#3157=FACE_OUTER_BOUND('',#4184,.T.);
#3158=FACE_OUTER_BOUND('',#4185,.T.);
#3159=FACE_OUTER_BOUND('',#4186,.T.);
#3160=FACE_OUTER_BOUND('',#4187,.T.);
#3161=FACE_OUTER_BOUND('',#4188,.T.);
#3162=FACE_OUTER_BOUND('',#4189,.T.);
#3163=FACE_OUTER_BOUND('',#4190,.T.);
#3164=FACE_OUTER_BOUND('',#4191,.T.);
#3165=FACE_OUTER_BOUND('',#4192,.T.);
#3166=FACE_OUTER_BOUND('',#4193,.T.);
#3167=FACE_OUTER_BOUND('',#4194,.T.);
#3168=FACE_OUTER_BOUND('',#4195,.T.);
#3169=FACE_OUTER_BOUND('',#4196,.T.);
#3170=FACE_OUTER_BOUND('',#4197,.T.);
#3171=FACE_OUTER_BOUND('',#4198,.T.);
#3172=FACE_OUTER_BOUND('',#4199,.T.);
#3173=FACE_OUTER_BOUND('',#4200,.T.);
#3174=FACE_OUTER_BOUND('',#4201,.T.);
#3175=FACE_OUTER_BOUND('',#4202,.T.);
#3176=FACE_OUTER_BOUND('',#4203,.T.);
#3177=FACE_OUTER_BOUND('',#4204,.T.);
#3178=FACE_OUTER_BOUND('',#4205,.T.);
#3179=FACE_OUTER_BOUND('',#4206,.T.);
#3180=FACE_OUTER_BOUND('',#4207,.T.);
#3181=FACE_OUTER_BOUND('',#4208,.T.);
#3182=FACE_OUTER_BOUND('',#4209,.T.);
#3183=FACE_OUTER_BOUND('',#4210,.T.);
#3184=FACE_OUTER_BOUND('',#4211,.T.);
#3185=FACE_OUTER_BOUND('',#4212,.T.);
#3186=FACE_OUTER_BOUND('',#4213,.T.);
#3187=FACE_OUTER_BOUND('',#4214,.T.);
#3188=FACE_OUTER_BOUND('',#4215,.T.);
#3189=FACE_OUTER_BOUND('',#4216,.T.);
#3190=FACE_OUTER_BOUND('',#4217,.T.);
#3191=FACE_OUTER_BOUND('',#4218,.T.);
#3192=FACE_OUTER_BOUND('',#4219,.T.);
#3193=FACE_OUTER_BOUND('',#4220,.T.);
#3194=FACE_OUTER_BOUND('',#4221,.T.);
#3195=FACE_OUTER_BOUND('',#4222,.T.);
#3196=FACE_OUTER_BOUND('',#4223,.T.);
#3197=FACE_OUTER_BOUND('',#4224,.T.);
#3198=FACE_OUTER_BOUND('',#4225,.T.);
#3199=FACE_OUTER_BOUND('',#4226,.T.);
#3200=FACE_OUTER_BOUND('',#4227,.T.);
#3201=FACE_OUTER_BOUND('',#4228,.T.);
#3202=FACE_OUTER_BOUND('',#4229,.T.);
#3203=FACE_OUTER_BOUND('',#4230,.T.);
#3204=FACE_OUTER_BOUND('',#4231,.T.);
#3205=FACE_OUTER_BOUND('',#4232,.T.);
#3206=FACE_OUTER_BOUND('',#4233,.T.);
#3207=FACE_OUTER_BOUND('',#4234,.T.);
#3208=FACE_OUTER_BOUND('',#4235,.T.);
#3209=FACE_OUTER_BOUND('',#4236,.T.);
#3210=FACE_OUTER_BOUND('',#4237,.T.);
#3211=FACE_OUTER_BOUND('',#4238,.T.);
#3212=FACE_OUTER_BOUND('',#4239,.T.);
#3213=FACE_OUTER_BOUND('',#4240,.T.);
#3214=FACE_OUTER_BOUND('',#4241,.T.);
#3215=FACE_OUTER_BOUND('',#4242,.T.);
#3216=FACE_OUTER_BOUND('',#4243,.T.);
#3217=FACE_OUTER_BOUND('',#4244,.T.);
#3218=FACE_OUTER_BOUND('',#4245,.T.);
#3219=FACE_OUTER_BOUND('',#4246,.T.);
#3220=FACE_OUTER_BOUND('',#4247,.T.);
#3221=FACE_OUTER_BOUND('',#4248,.T.);
#3222=FACE_OUTER_BOUND('',#4249,.T.);
#3223=FACE_OUTER_BOUND('',#4250,.T.);
#3224=FACE_OUTER_BOUND('',#4251,.T.);
#3225=FACE_OUTER_BOUND('',#4252,.T.);
#3226=FACE_OUTER_BOUND('',#4253,.T.);
#3227=FACE_OUTER_BOUND('',#4254,.T.);
#3228=FACE_OUTER_BOUND('',#4255,.T.);
#3229=FACE_OUTER_BOUND('',#4256,.T.);
#3230=FACE_OUTER_BOUND('',#4257,.T.);
#3231=FACE_OUTER_BOUND('',#4258,.T.);
#3232=FACE_OUTER_BOUND('',#4259,.T.);
#3233=FACE_OUTER_BOUND('',#4260,.T.);
#3234=FACE_OUTER_BOUND('',#4261,.T.);
#3235=FACE_OUTER_BOUND('',#4262,.T.);
#3236=FACE_OUTER_BOUND('',#4263,.T.);
#3237=FACE_OUTER_BOUND('',#4264,.T.);
#3238=FACE_OUTER_BOUND('',#4265,.T.);
#3239=FACE_OUTER_BOUND('',#4266,.T.);
#3240=FACE_OUTER_BOUND('',#4267,.T.);
#3241=FACE_OUTER_BOUND('',#4268,.T.);
#3242=FACE_OUTER_BOUND('',#4269,.T.);
#3243=FACE_OUTER_BOUND('',#4270,.T.);
#3244=FACE_OUTER_BOUND('',#4271,.T.);
#3245=FACE_OUTER_BOUND('',#4272,.T.);
#3246=FACE_OUTER_BOUND('',#4273,.T.);
#3247=FACE_OUTER_BOUND('',#4274,.T.);
#3248=FACE_OUTER_BOUND('',#4275,.T.);
#3249=FACE_OUTER_BOUND('',#4276,.T.);
#3250=FACE_OUTER_BOUND('',#4277,.T.);
#3251=FACE_OUTER_BOUND('',#4278,.T.);
#3252=FACE_OUTER_BOUND('',#4279,.T.);
#3253=FACE_OUTER_BOUND('',#4280,.T.);
#3254=FACE_OUTER_BOUND('',#4281,.T.);
#3255=FACE_OUTER_BOUND('',#4282,.T.);
#3256=FACE_OUTER_BOUND('',#4283,.T.);
#3257=FACE_OUTER_BOUND('',#4284,.T.);
#3258=FACE_OUTER_BOUND('',#4285,.T.);
#3259=FACE_OUTER_BOUND('',#4286,.T.);
#3260=FACE_OUTER_BOUND('',#4288,.T.);
#3261=FACE_OUTER_BOUND('',#4289,.T.);
#3262=FACE_OUTER_BOUND('',#4290,.T.);
#4159=EDGE_LOOP('',(#14855,#14856,#14857,#14858));
#4160=EDGE_LOOP('',(#14859,#14860,#14861,#14862));
#4161=EDGE_LOOP('',(#14863,#14864,#14865,#14866));
#4162=EDGE_LOOP('',(#14867,#14868,#14869,#14870));
#4163=EDGE_LOOP('',(#14871,#14872,#14873,#14874));
#4164=EDGE_LOOP('',(#14875,#14876,#14877,#14878));
#4165=EDGE_LOOP('',(#14879,#14880,#14881,#14882));
#4166=EDGE_LOOP('',(#14883,#14884,#14885,#14886));
#4167=EDGE_LOOP('',(#14887,#14888,#14889,#14890));
#4168=EDGE_LOOP('',(#14891,#14892,#14893,#14894));
#4169=EDGE_LOOP('',(#14895,#14896,#14897,#14898));
#4170=EDGE_LOOP('',(#14899,#14900,#14901,#14902));
#4171=EDGE_LOOP('',(#14903,#14904,#14905,#14906));
#4172=EDGE_LOOP('',(#14907,#14908,#14909,#14910));
#4173=EDGE_LOOP('',(#14911,#14912,#14913,#14914));
#4174=EDGE_LOOP('',(#14915,#14916,#14917,#14918));
#4175=EDGE_LOOP('',(#14919,#14920,#14921,#14922));
#4176=EDGE_LOOP('',(#14923,#14924,#14925,#14926));
#4177=EDGE_LOOP('',(#14927,#14928,#14929,#14930));
#4178=EDGE_LOOP('',(#14931,#14932,#14933,#14934));
#4179=EDGE_LOOP('',(#14935,#14936,#14937,#14938));
#4180=EDGE_LOOP('',(#14939,#14940,#14941,#14942));
#4181=EDGE_LOOP('',(#14943,#14944,#14945,#14946));
#4182=EDGE_LOOP('',(#14947,#14948,#14949,#14950));
#4183=EDGE_LOOP('',(#14951,#14952,#14953,#14954));
#4184=EDGE_LOOP('',(#14955,#14956,#14957,#14958));
#4185=EDGE_LOOP('',(#14959,#14960,#14961,#14962));
#4186=EDGE_LOOP('',(#14963,#14964,#14965,#14966));
#4187=EDGE_LOOP('',(#14967,#14968,#14969,#14970));
#4188=EDGE_LOOP('',(#14971,#14972,#14973,#14974,#14975,#14976,#14977,#14978,
#14979,#14980,#14981,#14982,#14983,#14984,#14985,#14986,#14987,#14988,#14989,
#14990,#14991,#14992,#14993,#14994,#14995,#14996,#14997,#14998,#14999,#15000,
#15001,#15002,#15003));
#4189=EDGE_LOOP('',(#15004,#15005,#15006,#15007,#15008));
#4190=EDGE_LOOP('',(#15009,#15010,#15011,#15012));
#4191=EDGE_LOOP('',(#15013,#15014,#15015,#15016,#15017,#15018,#15019,#15020,
#15021,#15022,#15023,#15024,#15025,#15026,#15027,#15028,#15029,#15030,#15031,
#15032,#15033,#15034,#15035,#15036,#15037,#15038,#15039,#15040,#15041,#15042,
#15043,#15044,#15045));
#4192=EDGE_LOOP('',(#15046,#15047,#15048,#15049));
#4193=EDGE_LOOP('',(#15050,#15051,#15052));
#4194=EDGE_LOOP('',(#15053,#15054,#15055,#15056));
#4195=EDGE_LOOP('',(#15057,#15058,#15059,#15060,#15061,#15062,#15063,#15064,
#15065,#15066,#15067,#15068,#15069,#15070,#15071,#15072,#15073,#15074,#15075,
#15076,#15077,#15078,#15079,#15080,#15081,#15082,#15083,#15084,#15085,#15086,
#15087,#15088,#15089,#15090,#15091,#15092,#15093,#15094,#15095,#15096,#15097,
#15098,#15099,#15100,#15101,#15102,#15103,#15104,#15105,#15106,#15107,#15108,
#15109,#15110,#15111,#15112,#15113,#15114,#15115,#15116,#15117,#15118,#15119,
#15120,#15121,#15122,#15123,#15124,#15125,#15126,#15127,#15128,#15129,#15130,
#15131,#15132,#15133,#15134,#15135,#15136,#15137,#15138,#15139,#15140,#15141,
#15142,#15143,#15144,#15145,#15146,#15147,#15148,#15149,#15150,#15151,#15152,
#15153,#15154,#15155,#15156,#15157,#15158,#15159,#15160,#15161,#15162,#15163,
#15164,#15165,#15166,#15167,#15168,#15169,#15170,#15171,#15172,#15173,#15174,
#15175,#15176,#15177,#15178,#15179,#15180));
#4196=EDGE_LOOP('',(#15181,#15182,#15183,#15184));
#4197=EDGE_LOOP('',(#15185,#15186,#15187));
#4198=EDGE_LOOP('',(#15188,#15189,#15190,#15191));
#4199=EDGE_LOOP('',(#15192,#15193,#15194,#15195));
#4200=EDGE_LOOP('',(#15196,#15197,#15198));
#4201=EDGE_LOOP('',(#15199,#15200,#15201,#15202));
#4202=EDGE_LOOP('',(#15203,#15204,#15205,#15206));
#4203=EDGE_LOOP('',(#15207,#15208,#15209));
#4204=EDGE_LOOP('',(#15210,#15211,#15212,#15213));
#4205=EDGE_LOOP('',(#15214,#15215,#15216,#15217));
#4206=EDGE_LOOP('',(#15218,#15219,#15220));
#4207=EDGE_LOOP('',(#15221,#15222,#15223,#15224));
#4208=EDGE_LOOP('',(#15225,#15226,#15227,#15228));
#4209=EDGE_LOOP('',(#15229,#15230,#15231));
#4210=EDGE_LOOP('',(#15232,#15233,#15234,#15235));
#4211=EDGE_LOOP('',(#15236,#15237,#15238,#15239));
#4212=EDGE_LOOP('',(#15240,#15241,#15242));
#4213=EDGE_LOOP('',(#15243,#15244,#15245,#15246));
#4214=EDGE_LOOP('',(#15247,#15248,#15249,#15250));
#4215=EDGE_LOOP('',(#15251,#15252,#15253));
#4216=EDGE_LOOP('',(#15254,#15255,#15256,#15257));
#4217=EDGE_LOOP('',(#15258,#15259,#15260,#15261));
#4218=EDGE_LOOP('',(#15262,#15263,#15264));
#4219=EDGE_LOOP('',(#15265,#15266,#15267,#15268));
#4220=EDGE_LOOP('',(#15269,#15270,#15271,#15272));
#4221=EDGE_LOOP('',(#15273,#15274,#15275));
#4222=EDGE_LOOP('',(#15276,#15277,#15278,#15279));
#4223=EDGE_LOOP('',(#15280,#15281,#15282,#15283));
#4224=EDGE_LOOP('',(#15284,#15285,#15286));
#4225=EDGE_LOOP('',(#15287,#15288,#15289,#15290));
#4226=EDGE_LOOP('',(#15291,#15292,#15293,#15294));
#4227=EDGE_LOOP('',(#15295,#15296,#15297));
#4228=EDGE_LOOP('',(#15298,#15299,#15300,#15301));
#4229=EDGE_LOOP('',(#15302,#15303,#15304,#15305));
#4230=EDGE_LOOP('',(#15306,#15307,#15308));
#4231=EDGE_LOOP('',(#15309,#15310,#15311,#15312));
#4232=EDGE_LOOP('',(#15313,#15314,#15315,#15316));
#4233=EDGE_LOOP('',(#15317,#15318,#15319));
#4234=EDGE_LOOP('',(#15320,#15321,#15322,#15323));
#4235=EDGE_LOOP('',(#15324,#15325,#15326,#15327));
#4236=EDGE_LOOP('',(#15328,#15329,#15330,#15331));
#4237=EDGE_LOOP('',(#15332,#15333,#15334,#15335));
#4238=EDGE_LOOP('',(#15336,#15337,#15338,#15339));
#4239=EDGE_LOOP('',(#15340,#15341,#15342));
#4240=EDGE_LOOP('',(#15343,#15344,#15345,#15346));
#4241=EDGE_LOOP('',(#15347,#15348,#15349,#15350));
#4242=EDGE_LOOP('',(#15351,#15352,#15353));
#4243=EDGE_LOOP('',(#15354,#15355,#15356,#15357));
#4244=EDGE_LOOP('',(#15358,#15359,#15360,#15361));
#4245=EDGE_LOOP('',(#15362,#15363,#15364));
#4246=EDGE_LOOP('',(#15365,#15366,#15367,#15368));
#4247=EDGE_LOOP('',(#15369,#15370,#15371,#15372));
#4248=EDGE_LOOP('',(#15373,#15374,#15375));
#4249=EDGE_LOOP('',(#15376,#15377,#15378,#15379));
#4250=EDGE_LOOP('',(#15380,#15381,#15382,#15383));
#4251=EDGE_LOOP('',(#15384,#15385,#15386));
#4252=EDGE_LOOP('',(#15387,#15388,#15389,#15390));
#4253=EDGE_LOOP('',(#15391,#15392,#15393,#15394));
#4254=EDGE_LOOP('',(#15395,#15396,#15397));
#4255=EDGE_LOOP('',(#15398,#15399,#15400,#15401));
#4256=EDGE_LOOP('',(#15402,#15403,#15404,#15405));
#4257=EDGE_LOOP('',(#15406,#15407,#15408));
#4258=EDGE_LOOP('',(#15409,#15410,#15411,#15412));
#4259=EDGE_LOOP('',(#15413,#15414,#15415,#15416));
#4260=EDGE_LOOP('',(#15417,#15418,#15419));
#4261=EDGE_LOOP('',(#15420,#15421,#15422,#15423));
#4262=EDGE_LOOP('',(#15424,#15425,#15426,#15427));
#4263=EDGE_LOOP('',(#15428,#15429,#15430));
#4264=EDGE_LOOP('',(#15431,#15432,#15433,#15434));
#4265=EDGE_LOOP('',(#15435,#15436,#15437,#15438));
#4266=EDGE_LOOP('',(#15439,#15440,#15441));
#4267=EDGE_LOOP('',(#15442,#15443,#15444,#15445));
#4268=EDGE_LOOP('',(#15446,#15447,#15448,#15449));
#4269=EDGE_LOOP('',(#15450,#15451,#15452));
#4270=EDGE_LOOP('',(#15453,#15454,#15455,#15456));
#4271=EDGE_LOOP('',(#15457,#15458,#15459,#15460));
#4272=EDGE_LOOP('',(#15461,#15462,#15463));
#4273=EDGE_LOOP('',(#15464,#15465,#15466,#15467));
#4274=EDGE_LOOP('',(#15468,#15469,#15470,#15471));
#4275=EDGE_LOOP('',(#15472,#15473,#15474));
#4276=EDGE_LOOP('',(#15475,#15476,#15477,#15478));
#4277=EDGE_LOOP('',(#15479,#15480,#15481,#15482));
#4278=EDGE_LOOP('',(#15483,#15484,#15485));
#4279=EDGE_LOOP('',(#15486,#15487,#15488,#15489));
#4280=EDGE_LOOP('',(#15490,#15491,#15492,#15493));
#4281=EDGE_LOOP('',(#15494,#15495,#15496));
#4282=EDGE_LOOP('',(#15497,#15498,#15499,#15500));
#4283=EDGE_LOOP('',(#15501));
#4284=EDGE_LOOP('',(#15502,#15503,#15504,#15505,#15506,#15507));
#4285=EDGE_LOOP('',(#15508,#15509,#15510,#15511));
#4286=EDGE_LOOP('',(#15512));
#4287=EDGE_LOOP('',(#15513,#15514,#15515,#15516));
#4288=EDGE_LOOP('',(#15517,#15518,#15519,#15520));
#4289=EDGE_LOOP('',(#15521,#15522,#15523,#15524,#15525,#15526,#15527,#15528,
#15529,#15530,#15531,#15532,#15533,#15534,#15535,#15536,#15537,#15538,#15539,
#15540,#15541,#15542,#15543,#15544,#15545,#15546,#15547,#15548,#15549,#15550,
#15551,#15552,#15553,#15554,#15555,#15556,#15557,#15558,#15559,#15560,#15561,
#15562,#15563,#15564,#15565,#15566,#15567,#15568,#15569,#15570,#15571,#15572,
#15573,#15574,#15575,#15576,#15577,#15578,#15579,#15580,#15581,#15582,#15583,
#15584,#15585,#15586,#15587,#15588,#15589,#15590,#15591,#15592,#15593,#15594,
#15595,#15596,#15597,#15598,#15599,#15600,#15601,#15602,#15603,#15604,#15605,
#15606,#15607,#15608,#15609,#15610,#15611,#15612,#15613));
#4290=EDGE_LOOP('',(#15614));
#5083=LINE('',#35575,#6058);
#5084=LINE('',#35599,#6059);
#5085=LINE('',#35647,#6060);
#5086=LINE('',#35695,#6061);
#5087=LINE('',#35749,#6062);
#5088=LINE('',#35797,#6063);
#5089=LINE('',#35845,#6064);
#5090=LINE('',#35893,#6065);
#5091=LINE('',#35947,#6066);
#5092=LINE('',#35995,#6067);
#5093=LINE('',#36043,#6068);
#5094=LINE('',#36097,#6069);
#5095=LINE('',#36145,#6070);
#5096=LINE('',#36193,#6071);
#5097=LINE('',#36247,#6072);
#5098=LINE('',#36295,#6073);
#5099=LINE('',#36319,#6074);
#5100=LINE('',#36344,#6075);
#5101=LINE('',#36369,#6076);
#5102=LINE('',#36393,#6077);
#5103=LINE('',#36418,#6078);
#5104=LINE('',#36443,#6079);
#5105=LINE('',#36467,#6080);
#5106=LINE('',#36492,#6081);
#5107=LINE('',#36517,#6082);
#5108=LINE('',#36541,#6083);
#5109=LINE('',#36565,#6084);
#5110=LINE('',#36590,#6085);
#5111=LINE('',#36615,#6086);
#5112=LINE('',#37809,#6087);
#5113=LINE('',#37811,#6088);
#5114=LINE('',#37812,#6089);
#5115=LINE('',#37816,#6090);
#5116=LINE('',#37822,#6091);
#5117=LINE('',#37827,#6092);
#5118=LINE('',#37831,#6093);
#5119=LINE('',#37835,#6094);
#5120=LINE('',#37839,#6095);
#5121=LINE('',#37843,#6096);
#5122=LINE('',#37847,#6097);
#5123=LINE('',#37851,#6098);
#5124=LINE('',#37855,#6099);
#5125=LINE('',#37859,#6100);
#5126=LINE('',#37863,#6101);
#5127=LINE('',#37867,#6102);
#5128=LINE('',#37871,#6103);
#5129=LINE('',#37875,#6104);
#5130=LINE('',#37879,#6105);
#5131=LINE('',#37883,#6106);
#5132=LINE('',#37887,#6107);
#5133=LINE('',#37891,#6108);
#5134=LINE('',#37895,#6109);
#5135=LINE('',#37899,#6110);
#5136=LINE('',#37903,#6111);
#5137=LINE('',#37907,#6112);
#5138=LINE('',#37911,#6113);
#5139=LINE('',#37915,#6114);
#5140=LINE('',#37919,#6115);
#5141=LINE('',#37923,#6116);
#5142=LINE('',#37927,#6117);
#5143=LINE('',#37931,#6118);
#5144=LINE('',#37935,#6119);
#5145=LINE('',#37940,#6120);
#5146=LINE('',#37944,#6121);
#5147=LINE('',#37948,#6122);
#5148=LINE('',#37952,#6123);
#5149=LINE('',#37956,#6124);
#5150=LINE('',#37960,#6125);
#5151=LINE('',#37964,#6126);
#5152=LINE('',#37968,#6127);
#5153=LINE('',#37972,#6128);
#5154=LINE('',#37976,#6129);
#5155=LINE('',#37980,#6130);
#5156=LINE('',#37984,#6131);
#5157=LINE('',#37988,#6132);
#5158=LINE('',#37992,#6133);
#5159=LINE('',#37996,#6134);
#5160=LINE('',#38000,#6135);
#5161=LINE('',#38004,#6136);
#5162=LINE('',#38008,#6137);
#5163=LINE('',#38012,#6138);
#5164=LINE('',#38016,#6139);
#5165=LINE('',#38020,#6140);
#5166=LINE('',#38024,#6141);
#5167=LINE('',#38028,#6142);
#5168=LINE('',#38032,#6143);
#5169=LINE('',#38036,#6144);
#5170=LINE('',#38040,#6145);
#5171=LINE('',#38044,#6146);
#5172=LINE('',#38048,#6147);
#5173=LINE('',#38052,#6148);
#5174=LINE('',#38056,#6149);
#5175=LINE('',#38060,#6150);
#5176=LINE('',#38068,#6151);
#5177=LINE('',#38069,#6152);
#5178=LINE('',#38071,#6153);
#5179=LINE('',#38082,#6154);
#5180=LINE('',#38083,#6155);
#5181=LINE('',#38085,#6156);
#5182=LINE('',#38096,#6157);
#5183=LINE('',#38097,#6158);
#5184=LINE('',#38099,#6159);
#5185=LINE('',#38110,#6160);
#5186=LINE('',#38111,#6161);
#5187=LINE('',#38113,#6162);
#5188=LINE('',#38124,#6163);
#5189=LINE('',#38125,#6164);
#5190=LINE('',#38127,#6165);
#5191=LINE('',#38138,#6166);
#5192=LINE('',#38139,#6167);
#5193=LINE('',#38141,#6168);
#5194=LINE('',#38152,#6169);
#5195=LINE('',#38153,#6170);
#5196=LINE('',#38155,#6171);
#5197=LINE('',#38166,#6172);
#5198=LINE('',#38167,#6173);
#5199=LINE('',#38169,#6174);
#5200=LINE('',#38180,#6175);
#5201=LINE('',#38181,#6176);
#5202=LINE('',#38183,#6177);
#5203=LINE('',#38194,#6178);
#5204=LINE('',#38195,#6179);
#5205=LINE('',#38197,#6180);
#5206=LINE('',#38208,#6181);
#5207=LINE('',#38209,#6182);
#5208=LINE('',#38211,#6183);
#5209=LINE('',#38222,#6184);
#5210=LINE('',#38223,#6185);
#5211=LINE('',#38225,#6186);
#5212=LINE('',#38236,#6187);
#5213=LINE('',#38237,#6188);
#5214=LINE('',#38239,#6189);
#5215=LINE('',#38250,#6190);
#5216=LINE('',#38251,#6191);
#5217=LINE('',#38253,#6192);
#5218=LINE('',#38264,#6193);
#5219=LINE('',#38265,#6194);
#5220=LINE('',#38267,#6195);
#5221=LINE('',#38278,#6196);
#5222=LINE('',#38279,#6197);
#5223=LINE('',#38281,#6198);
#5224=LINE('',#38292,#6199);
#5225=LINE('',#38293,#6200);
#5226=LINE('',#38295,#6201);
#5227=LINE('',#38306,#6202);
#5228=LINE('',#38307,#6203);
#5229=LINE('',#38309,#6204);
#5230=LINE('',#38320,#6205);
#5231=LINE('',#38321,#6206);
#5232=LINE('',#38323,#6207);
#5233=LINE('',#38334,#6208);
#5234=LINE('',#38335,#6209);
#5235=LINE('',#38337,#6210);
#5236=LINE('',#38348,#6211);
#5237=LINE('',#38349,#6212);
#5238=LINE('',#38351,#6213);
#5239=LINE('',#38362,#6214);
#5240=LINE('',#38363,#6215);
#5241=LINE('',#38365,#6216);
#5242=LINE('',#38376,#6217);
#5243=LINE('',#38377,#6218);
#5244=LINE('',#38379,#6219);
#5245=LINE('',#38390,#6220);
#5246=LINE('',#38391,#6221);
#5247=LINE('',#38393,#6222);
#5248=LINE('',#38404,#6223);
#5249=LINE('',#38405,#6224);
#5250=LINE('',#38407,#6225);
#5251=LINE('',#38418,#6226);
#5252=LINE('',#38419,#6227);
#5253=LINE('',#38421,#6228);
#5254=LINE('',#38432,#6229);
#5255=LINE('',#38433,#6230);
#5256=LINE('',#38435,#6231);
#5257=LINE('',#38446,#6232);
#5258=LINE('',#38447,#6233);
#5259=LINE('',#38449,#6234);
#5260=LINE('',#38460,#6235);
#5261=LINE('',#38461,#6236);
#5262=LINE('',#38463,#6237);
#5263=LINE('',#38472,#6238);
#5264=LINE('',#38479,#6239);
#5265=LINE('',#38483,#6240);
#6058=VECTOR('',#23003,2.5);
#6059=VECTOR('',#23008,2.5);
#6060=VECTOR('',#23011,2.5);
#6061=VECTOR('',#23014,2.5);
#6062=VECTOR('',#23017,2.5);
#6063=VECTOR('',#23020,2.5);
#6064=VECTOR('',#23023,2.5);
#6065=VECTOR('',#23026,2.5);
#6066=VECTOR('',#23029,2.5);
#6067=VECTOR('',#23032,2.5);
#6068=VECTOR('',#23035,2.5);
#6069=VECTOR('',#23038,2.5);
#6070=VECTOR('',#23041,2.5);
#6071=VECTOR('',#23044,2.5);
#6072=VECTOR('',#23047,2.5);
#6073=VECTOR('',#23050,1.99475);
#6074=VECTOR('',#23055,1.99475);
#6075=VECTOR('',#23058,1.99475);
#6076=VECTOR('',#23061,1.99475);
#6077=VECTOR('',#23064,1.99475);
#6078=VECTOR('',#23067,1.99475);
#6079=VECTOR('',#23070,1.99475);
#6080=VECTOR('',#23073,1.99475);
#6081=VECTOR('',#23076,1.99475);
#6082=VECTOR('',#23079,1.99475);
#6083=VECTOR('',#23082,1.99475);
#6084=VECTOR('',#23085,1.99475);
#6085=VECTOR('',#23088,1.99475);
#6086=VECTOR('',#23091,1.99475);
#6087=VECTOR('',#23104,10.);
#6088=VECTOR('',#23105,10.);
#6089=VECTOR('',#23106,10.);
#6090=VECTOR('',#23111,10.);
#6091=VECTOR('',#23114,10.);
#6092=VECTOR('',#23119,10.);
#6093=VECTOR('',#23122,10.);
#6094=VECTOR('',#23125,10.);
#6095=VECTOR('',#23128,10.);
#6096=VECTOR('',#23131,10.);
#6097=VECTOR('',#23134,10.);
#6098=VECTOR('',#23137,10.);
#6099=VECTOR('',#23140,10.);
#6100=VECTOR('',#23143,10.);
#6101=VECTOR('',#23146,10.);
#6102=VECTOR('',#23149,10.);
#6103=VECTOR('',#23152,10.);
#6104=VECTOR('',#23155,10.);
#6105=VECTOR('',#23158,10.);
#6106=VECTOR('',#23161,10.);
#6107=VECTOR('',#23164,10.);
#6108=VECTOR('',#23167,10.);
#6109=VECTOR('',#23170,10.);
#6110=VECTOR('',#23173,10.);
#6111=VECTOR('',#23176,10.);
#6112=VECTOR('',#23179,10.);
#6113=VECTOR('',#23182,10.);
#6114=VECTOR('',#23185,10.);
#6115=VECTOR('',#23188,10.);
#6116=VECTOR('',#23191,10.);
#6117=VECTOR('',#23194,10.);
#6118=VECTOR('',#23197,10.);
#6119=VECTOR('',#23200,5.);
#6120=VECTOR('',#23205,10.);
#6121=VECTOR('',#23208,10.);
#6122=VECTOR('',#23211,10.);
#6123=VECTOR('',#23214,10.);
#6124=VECTOR('',#23217,10.);
#6125=VECTOR('',#23220,10.);
#6126=VECTOR('',#23223,10.);
#6127=VECTOR('',#23226,10.);
#6128=VECTOR('',#23229,10.);
#6129=VECTOR('',#23232,10.);
#6130=VECTOR('',#23235,10.);
#6131=VECTOR('',#23238,10.);
#6132=VECTOR('',#23241,10.);
#6133=VECTOR('',#23244,10.);
#6134=VECTOR('',#23247,10.);
#6135=VECTOR('',#23250,10.);
#6136=VECTOR('',#23253,10.);
#6137=VECTOR('',#23256,10.);
#6138=VECTOR('',#23259,10.);
#6139=VECTOR('',#23262,10.);
#6140=VECTOR('',#23265,10.);
#6141=VECTOR('',#23268,10.);
#6142=VECTOR('',#23271,10.);
#6143=VECTOR('',#23274,10.);
#6144=VECTOR('',#23277,10.);
#6145=VECTOR('',#23280,10.);
#6146=VECTOR('',#23283,10.);
#6147=VECTOR('',#23286,10.);
#6148=VECTOR('',#23289,10.);
#6149=VECTOR('',#23292,10.);
#6150=VECTOR('',#23295,10.);
#6151=VECTOR('',#23300,10.);
#6152=VECTOR('',#23301,10.);
#6153=VECTOR('',#23304,10.);
#6154=VECTOR('',#23309,10.);
#6155=VECTOR('',#23310,10.);
#6156=VECTOR('',#23313,10.);
#6157=VECTOR('',#23318,10.);
#6158=VECTOR('',#23319,10.);
#6159=VECTOR('',#23322,10.);
#6160=VECTOR('',#23327,10.);
#6161=VECTOR('',#23328,10.);
#6162=VECTOR('',#23331,10.);
#6163=VECTOR('',#23336,10.);
#6164=VECTOR('',#23337,10.);
#6165=VECTOR('',#23340,10.);
#6166=VECTOR('',#23345,10.);
#6167=VECTOR('',#23346,10.);
#6168=VECTOR('',#23349,10.);
#6169=VECTOR('',#23354,10.);
#6170=VECTOR('',#23355,10.);
#6171=VECTOR('',#23358,10.);
#6172=VECTOR('',#23363,10.);
#6173=VECTOR('',#23364,10.);
#6174=VECTOR('',#23367,10.);
#6175=VECTOR('',#23372,10.);
#6176=VECTOR('',#23373,10.);
#6177=VECTOR('',#23376,10.);
#6178=VECTOR('',#23381,10.);
#6179=VECTOR('',#23382,10.);
#6180=VECTOR('',#23385,10.);
#6181=VECTOR('',#23390,10.);
#6182=VECTOR('',#23391,10.);
#6183=VECTOR('',#23394,10.);
#6184=VECTOR('',#23399,10.);
#6185=VECTOR('',#23400,10.);
#6186=VECTOR('',#23403,10.);
#6187=VECTOR('',#23408,10.);
#6188=VECTOR('',#23409,10.);
#6189=VECTOR('',#23412,10.);
#6190=VECTOR('',#23417,10.);
#6191=VECTOR('',#23418,10.);
#6192=VECTOR('',#23421,10.);
#6193=VECTOR('',#23426,10.);
#6194=VECTOR('',#23427,10.);
#6195=VECTOR('',#23430,10.);
#6196=VECTOR('',#23435,10.);
#6197=VECTOR('',#23436,10.);
#6198=VECTOR('',#23439,10.);
#6199=VECTOR('',#23444,10.);
#6200=VECTOR('',#23445,10.);
#6201=VECTOR('',#23448,10.);
#6202=VECTOR('',#23453,10.);
#6203=VECTOR('',#23454,10.);
#6204=VECTOR('',#23457,10.);
#6205=VECTOR('',#23462,10.);
#6206=VECTOR('',#23463,10.);
#6207=VECTOR('',#23466,10.);
#6208=VECTOR('',#23471,10.);
#6209=VECTOR('',#23472,10.);
#6210=VECTOR('',#23475,10.);
#6211=VECTOR('',#23480,10.);
#6212=VECTOR('',#23481,10.);
#6213=VECTOR('',#23484,10.);
#6214=VECTOR('',#23489,10.);
#6215=VECTOR('',#23490,10.);
#6216=VECTOR('',#23493,10.);
#6217=VECTOR('',#23498,10.);
#6218=VECTOR('',#23499,10.);
#6219=VECTOR('',#23502,10.);
#6220=VECTOR('',#23507,10.);
#6221=VECTOR('',#23508,10.);
#6222=VECTOR('',#23511,10.);
#6223=VECTOR('',#23516,10.);
#6224=VECTOR('',#23517,10.);
#6225=VECTOR('',#23520,10.);
#6226=VECTOR('',#23525,10.);
#6227=VECTOR('',#23526,10.);
#6228=VECTOR('',#23529,10.);
#6229=VECTOR('',#23534,10.);
#6230=VECTOR('',#23535,10.);
#6231=VECTOR('',#23538,10.);
#6232=VECTOR('',#23543,10.);
#6233=VECTOR('',#23544,10.);
#6234=VECTOR('',#23547,10.);
#6235=VECTOR('',#23552,10.);
#6236=VECTOR('',#23553,10.);
#6237=VECTOR('',#23556,10.);
#6238=VECTOR('',#23565,2.3);
#6239=VECTOR('',#23576,4.75);
#6240=VECTOR('',#23581,4.7);
#7629=VERTEX_POINT('',#35573);
#7630=VERTEX_POINT('',#35574);
#7631=VERTEX_POINT('',#35576);
#7632=VERTEX_POINT('',#35587);
#7633=VERTEX_POINT('',#35597);
#7634=VERTEX_POINT('',#35598);
#7635=VERTEX_POINT('',#35645);
#7636=VERTEX_POINT('',#35646);
#7637=VERTEX_POINT('',#35693);
#7638=VERTEX_POINT('',#35694);
#7639=VERTEX_POINT('',#35747);
#7640=VERTEX_POINT('',#35748);
#7641=VERTEX_POINT('',#35795);
#7642=VERTEX_POINT('',#35796);
#7643=VERTEX_POINT('',#35843);
#7644=VERTEX_POINT('',#35844);
#7645=VERTEX_POINT('',#35891);
#7646=VERTEX_POINT('',#35892);
#7647=VERTEX_POINT('',#35945);
#7648=VERTEX_POINT('',#35946);
#7649=VERTEX_POINT('',#35993);
#7650=VERTEX_POINT('',#35994);
#7651=VERTEX_POINT('',#36041);
#7652=VERTEX_POINT('',#36042);
#7653=VERTEX_POINT('',#36095);
#7654=VERTEX_POINT('',#36096);
#7655=VERTEX_POINT('',#36143);
#7656=VERTEX_POINT('',#36144);
#7657=VERTEX_POINT('',#36191);
#7658=VERTEX_POINT('',#36192);
#7659=VERTEX_POINT('',#36245);
#7660=VERTEX_POINT('',#36246);
#7661=VERTEX_POINT('',#36293);
#7662=VERTEX_POINT('',#36294);
#7663=VERTEX_POINT('',#36296);
#7664=VERTEX_POINT('',#36306);
#7665=VERTEX_POINT('',#36317);
#7666=VERTEX_POINT('',#36318);
#7667=VERTEX_POINT('',#36342);
#7668=VERTEX_POINT('',#36343);
#7669=VERTEX_POINT('',#36367);
#7670=VERTEX_POINT('',#36368);
#7671=VERTEX_POINT('',#36391);
#7672=VERTEX_POINT('',#36392);
#7673=VERTEX_POINT('',#36416);
#7674=VERTEX_POINT('',#36417);
#7675=VERTEX_POINT('',#36441);
#7676=VERTEX_POINT('',#36442);
#7677=VERTEX_POINT('',#36465);
#7678=VERTEX_POINT('',#36466);
#7679=VERTEX_POINT('',#36490);
#7680=VERTEX_POINT('',#36491);
#7681=VERTEX_POINT('',#36515);
#7682=VERTEX_POINT('',#36516);
#7683=VERTEX_POINT('',#36539);
#7684=VERTEX_POINT('',#36540);
#7685=VERTEX_POINT('',#36563);
#7686=VERTEX_POINT('',#36564);
#7687=VERTEX_POINT('',#36588);
#7688=VERTEX_POINT('',#36589);
#7689=VERTEX_POINT('',#36613);
#7690=VERTEX_POINT('',#36614);
#7691=VERTEX_POINT('',#37024);
#7692=VERTEX_POINT('',#37123);
#7693=VERTEX_POINT('',#37219);
#7694=VERTEX_POINT('',#37222);
#7695=VERTEX_POINT('',#37709);
#7696=VERTEX_POINT('',#37803);
#7697=VERTEX_POINT('',#37804);
#7698=VERTEX_POINT('',#37808);
#7699=VERTEX_POINT('',#37810);
#7700=VERTEX_POINT('',#37814);
#7701=VERTEX_POINT('',#37818);
#7702=VERTEX_POINT('',#37824);
#7703=VERTEX_POINT('',#37826);
#7704=VERTEX_POINT('',#37828);
#7705=VERTEX_POINT('',#37830);
#7706=VERTEX_POINT('',#37832);
#7707=VERTEX_POINT('',#37834);
#7708=VERTEX_POINT('',#37836);
#7709=VERTEX_POINT('',#37838);
#7710=VERTEX_POINT('',#37840);
#7711=VERTEX_POINT('',#37842);
#7712=VERTEX_POINT('',#37844);
#7713=VERTEX_POINT('',#37846);
#7714=VERTEX_POINT('',#37848);
#7715=VERTEX_POINT('',#37850);
#7716=VERTEX_POINT('',#37852);
#7717=VERTEX_POINT('',#37854);
#7718=VERTEX_POINT('',#37856);
#7719=VERTEX_POINT('',#37858);
#7720=VERTEX_POINT('',#37860);
#7721=VERTEX_POINT('',#37862);
#7722=VERTEX_POINT('',#37864);
#7723=VERTEX_POINT('',#37866);
#7724=VERTEX_POINT('',#37868);
#7725=VERTEX_POINT('',#37870);
#7726=VERTEX_POINT('',#37872);
#7727=VERTEX_POINT('',#37874);
#7728=VERTEX_POINT('',#37876);
#7729=VERTEX_POINT('',#37878);
#7730=VERTEX_POINT('',#37880);
#7731=VERTEX_POINT('',#37882);
#7732=VERTEX_POINT('',#37884);
#7733=VERTEX_POINT('',#37886);
#7734=VERTEX_POINT('',#37888);
#7735=VERTEX_POINT('',#37890);
#7736=VERTEX_POINT('',#37892);
#7737=VERTEX_POINT('',#37894);
#7738=VERTEX_POINT('',#37896);
#7739=VERTEX_POINT('',#37898);
#7740=VERTEX_POINT('',#37900);
#7741=VERTEX_POINT('',#37902);
#7742=VERTEX_POINT('',#37904);
#7743=VERTEX_POINT('',#37906);
#7744=VERTEX_POINT('',#37908);
#7745=VERTEX_POINT('',#37910);
#7746=VERTEX_POINT('',#37912);
#7747=VERTEX_POINT('',#37914);
#7748=VERTEX_POINT('',#37916);
#7749=VERTEX_POINT('',#37918);
#7750=VERTEX_POINT('',#37920);
#7751=VERTEX_POINT('',#37922);
#7752=VERTEX_POINT('',#37924);
#7753=VERTEX_POINT('',#37926);
#7754=VERTEX_POINT('',#37928);
#7755=VERTEX_POINT('',#37930);
#7756=VERTEX_POINT('',#37932);
#7757=VERTEX_POINT('',#37934);
#7758=VERTEX_POINT('',#37937);
#7759=VERTEX_POINT('',#37939);
#7760=VERTEX_POINT('',#37941);
#7761=VERTEX_POINT('',#37943);
#7762=VERTEX_POINT('',#37945);
#7763=VERTEX_POINT('',#37947);
#7764=VERTEX_POINT('',#37949);
#7765=VERTEX_POINT('',#37951);
#7766=VERTEX_POINT('',#37953);
#7767=VERTEX_POINT('',#37955);
#7768=VERTEX_POINT('',#37957);
#7769=VERTEX_POINT('',#37959);
#7770=VERTEX_POINT('',#37961);
#7771=VERTEX_POINT('',#37963);
#7772=VERTEX_POINT('',#37965);
#7773=VERTEX_POINT('',#37967);
#7774=VERTEX_POINT('',#37969);
#7775=VERTEX_POINT('',#37971);
#7776=VERTEX_POINT('',#37973);
#7777=VERTEX_POINT('',#37975);
#7778=VERTEX_POINT('',#37977);
#7779=VERTEX_POINT('',#37979);
#7780=VERTEX_POINT('',#37981);
#7781=VERTEX_POINT('',#37983);
#7782=VERTEX_POINT('',#37985);
#7783=VERTEX_POINT('',#37987);
#7784=VERTEX_POINT('',#37989);
#7785=VERTEX_POINT('',#37991);
#7786=VERTEX_POINT('',#37993);
#7787=VERTEX_POINT('',#37995);
#7788=VERTEX_POINT('',#37997);
#7789=VERTEX_POINT('',#37999);
#7790=VERTEX_POINT('',#38001);
#7791=VERTEX_POINT('',#38003);
#7792=VERTEX_POINT('',#38005);
#7793=VERTEX_POINT('',#38007);
#7794=VERTEX_POINT('',#38009);
#7795=VERTEX_POINT('',#38011);
#7796=VERTEX_POINT('',#38013);
#7797=VERTEX_POINT('',#38015);
#7798=VERTEX_POINT('',#38017);
#7799=VERTEX_POINT('',#38019);
#7800=VERTEX_POINT('',#38021);
#7801=VERTEX_POINT('',#38023);
#7802=VERTEX_POINT('',#38025);
#7803=VERTEX_POINT('',#38027);
#7804=VERTEX_POINT('',#38029);
#7805=VERTEX_POINT('',#38031);
#7806=VERTEX_POINT('',#38033);
#7807=VERTEX_POINT('',#38035);
#7808=VERTEX_POINT('',#38037);
#7809=VERTEX_POINT('',#38039);
#7810=VERTEX_POINT('',#38041);
#7811=VERTEX_POINT('',#38043);
#7812=VERTEX_POINT('',#38045);
#7813=VERTEX_POINT('',#38047);
#7814=VERTEX_POINT('',#38049);
#7815=VERTEX_POINT('',#38051);
#7816=VERTEX_POINT('',#38053);
#7817=VERTEX_POINT('',#38055);
#7818=VERTEX_POINT('',#38057);
#7819=VERTEX_POINT('',#38059);
#7820=VERTEX_POINT('',#38063);
#7821=VERTEX_POINT('',#38067);
#7822=VERTEX_POINT('',#38077);
#7823=VERTEX_POINT('',#38081);
#7824=VERTEX_POINT('',#38091);
#7825=VERTEX_POINT('',#38095);
#7826=VERTEX_POINT('',#38105);
#7827=VERTEX_POINT('',#38109);
#7828=VERTEX_POINT('',#38119);
#7829=VERTEX_POINT('',#38123);
#7830=VERTEX_POINT('',#38133);
#7831=VERTEX_POINT('',#38137);
#7832=VERTEX_POINT('',#38147);
#7833=VERTEX_POINT('',#38151);
#7834=VERTEX_POINT('',#38161);
#7835=VERTEX_POINT('',#38165);
#7836=VERTEX_POINT('',#38175);
#7837=VERTEX_POINT('',#38179);
#7838=VERTEX_POINT('',#38189);
#7839=VERTEX_POINT('',#38193);
#7840=VERTEX_POINT('',#38203);
#7841=VERTEX_POINT('',#38207);
#7842=VERTEX_POINT('',#38217);
#7843=VERTEX_POINT('',#38221);
#7844=VERTEX_POINT('',#38231);
#7845=VERTEX_POINT('',#38235);
#7846=VERTEX_POINT('',#38245);
#7847=VERTEX_POINT('',#38249);
#7848=VERTEX_POINT('',#38259);
#7849=VERTEX_POINT('',#38263);
#7850=VERTEX_POINT('',#38273);
#7851=VERTEX_POINT('',#38277);
#7852=VERTEX_POINT('',#38287);
#7853=VERTEX_POINT('',#38291);
#7854=VERTEX_POINT('',#38301);
#7855=VERTEX_POINT('',#38305);
#7856=VERTEX_POINT('',#38315);
#7857=VERTEX_POINT('',#38319);
#7858=VERTEX_POINT('',#38329);
#7859=VERTEX_POINT('',#38333);
#7860=VERTEX_POINT('',#38343);
#7861=VERTEX_POINT('',#38347);
#7862=VERTEX_POINT('',#38357);
#7863=VERTEX_POINT('',#38361);
#7864=VERTEX_POINT('',#38371);
#7865=VERTEX_POINT('',#38375);
#7866=VERTEX_POINT('',#38385);
#7867=VERTEX_POINT('',#38389);
#7868=VERTEX_POINT('',#38399);
#7869=VERTEX_POINT('',#38403);
#7870=VERTEX_POINT('',#38413);
#7871=VERTEX_POINT('',#38417);
#7872=VERTEX_POINT('',#38427);
#7873=VERTEX_POINT('',#38431);
#7874=VERTEX_POINT('',#38441);
#7875=VERTEX_POINT('',#38445);
#7876=VERTEX_POINT('',#38455);
#7877=VERTEX_POINT('',#38459);
#7878=VERTEX_POINT('',#38469);
#7879=VERTEX_POINT('',#38476);
#7880=VERTEX_POINT('',#38481);
#10079=EDGE_CURVE('',#7629,#7630,#5083,.T.);
#10080=EDGE_CURVE('',#7629,#7631,#781,.T.);
#10081=EDGE_CURVE('',#7631,#7632,#2209,.T.);
#10082=EDGE_CURVE('',#7632,#7630,#782,.T.);
#10083=EDGE_CURVE('',#7633,#7634,#5084,.T.);
#10084=EDGE_CURVE('',#7633,#7629,#783,.T.);
#10085=EDGE_CURVE('',#7630,#7634,#784,.T.);
#10086=EDGE_CURVE('',#7635,#7636,#5085,.T.);
#10087=EDGE_CURVE('',#7635,#7633,#785,.T.);
#10088=EDGE_CURVE('',#7634,#7636,#786,.T.);
#10089=EDGE_CURVE('',#7637,#7638,#5086,.T.);
#10090=EDGE_CURVE('',#7637,#7635,#787,.T.);
#10091=EDGE_CURVE('',#7636,#7638,#788,.T.);
#10092=EDGE_CURVE('',#7639,#7640,#5087,.T.);
#10093=EDGE_CURVE('',#7639,#7637,#789,.T.);
#10094=EDGE_CURVE('',#7638,#7640,#790,.T.);
#10095=EDGE_CURVE('',#7641,#7642,#5088,.T.);
#10096=EDGE_CURVE('',#7641,#7639,#791,.T.);
#10097=EDGE_CURVE('',#7640,#7642,#792,.T.);
#10098=EDGE_CURVE('',#7643,#7644,#5089,.T.);
#10099=EDGE_CURVE('',#7643,#7641,#793,.T.);
#10100=EDGE_CURVE('',#7642,#7644,#794,.T.);
#10101=EDGE_CURVE('',#7645,#7646,#5090,.T.);
#10102=EDGE_CURVE('',#7645,#7643,#795,.T.);
#10103=EDGE_CURVE('',#7644,#7646,#796,.T.);
#10104=EDGE_CURVE('',#7647,#7648,#5091,.T.);
#10105=EDGE_CURVE('',#7647,#7645,#797,.T.);
#10106=EDGE_CURVE('',#7646,#7648,#798,.T.);
#10107=EDGE_CURVE('',#7649,#7650,#5092,.T.);
#10108=EDGE_CURVE('',#7649,#7647,#799,.T.);
#10109=EDGE_CURVE('',#7648,#7650,#800,.T.);
#10110=EDGE_CURVE('',#7651,#7652,#5093,.T.);
#10111=EDGE_CURVE('',#7651,#7649,#801,.T.);
#10112=EDGE_CURVE('',#7650,#7652,#802,.T.);
#10113=EDGE_CURVE('',#7653,#7654,#5094,.T.);
#10114=EDGE_CURVE('',#7653,#7651,#803,.T.);
#10115=EDGE_CURVE('',#7652,#7654,#804,.T.);
#10116=EDGE_CURVE('',#7655,#7656,#5095,.T.);
#10117=EDGE_CURVE('',#7655,#7653,#805,.T.);
#10118=EDGE_CURVE('',#7654,#7656,#806,.T.);
#10119=EDGE_CURVE('',#7657,#7658,#5096,.T.);
#10120=EDGE_CURVE('',#7657,#7655,#807,.T.);
#10121=EDGE_CURVE('',#7656,#7658,#808,.T.);
#10122=EDGE_CURVE('',#7659,#7660,#5097,.T.);
#10123=EDGE_CURVE('',#7659,#7657,#809,.T.);
#10124=EDGE_CURVE('',#7658,#7660,#810,.T.);
#10125=EDGE_CURVE('',#7661,#7662,#5098,.T.);
#10126=EDGE_CURVE('',#7661,#7663,#811,.T.);
#10127=EDGE_CURVE('',#7664,#7663,#2210,.T.);
#10128=EDGE_CURVE('',#7662,#7664,#812,.T.);
#10129=EDGE_CURVE('',#7665,#7666,#5099,.T.);
#10130=EDGE_CURVE('',#7665,#7661,#813,.T.);
#10131=EDGE_CURVE('',#7666,#7662,#814,.T.);
#10132=EDGE_CURVE('',#7667,#7668,#5100,.T.);
#10133=EDGE_CURVE('',#7667,#7665,#815,.T.);
#10134=EDGE_CURVE('',#7668,#7666,#816,.T.);
#10135=EDGE_CURVE('',#7669,#7670,#5101,.T.);
#10136=EDGE_CURVE('',#7669,#7667,#817,.T.);
#10137=EDGE_CURVE('',#7670,#7668,#818,.T.);
#10138=EDGE_CURVE('',#7671,#7672,#5102,.T.);
#10139=EDGE_CURVE('',#7671,#7669,#819,.T.);
#10140=EDGE_CURVE('',#7672,#7670,#820,.T.);
#10141=EDGE_CURVE('',#7673,#7674,#5103,.T.);
#10142=EDGE_CURVE('',#7673,#7671,#821,.T.);
#10143=EDGE_CURVE('',#7674,#7672,#822,.T.);
#10144=EDGE_CURVE('',#7675,#7676,#5104,.T.);
#10145=EDGE_CURVE('',#7675,#7673,#823,.T.);
#10146=EDGE_CURVE('',#7676,#7674,#824,.T.);
#10147=EDGE_CURVE('',#7677,#7678,#5105,.T.);
#10148=EDGE_CURVE('',#7677,#7675,#825,.T.);
#10149=EDGE_CURVE('',#7678,#7676,#826,.T.);
#10150=EDGE_CURVE('',#7679,#7680,#5106,.T.);
#10151=EDGE_CURVE('',#7679,#7677,#827,.T.);
#10152=EDGE_CURVE('',#7680,#7678,#828,.T.);
#10153=EDGE_CURVE('',#7681,#7682,#5107,.T.);
#10154=EDGE_CURVE('',#7681,#7679,#829,.T.);
#10155=EDGE_CURVE('',#7682,#7680,#830,.T.);
#10156=EDGE_CURVE('',#7683,#7684,#5108,.T.);
#10157=EDGE_CURVE('',#7683,#7681,#831,.T.);
#10158=EDGE_CURVE('',#7684,#7682,#832,.T.);
#10159=EDGE_CURVE('',#7685,#7686,#5109,.T.);
#10160=EDGE_CURVE('',#7685,#7683,#833,.T.);
#10161=EDGE_CURVE('',#7686,#7684,#834,.T.);
#10162=EDGE_CURVE('',#7687,#7688,#5110,.T.);
#10163=EDGE_CURVE('',#7687,#7685,#835,.T.);
#10164=EDGE_CURVE('',#7688,#7686,#836,.T.);
#10165=EDGE_CURVE('',#7689,#7690,#5111,.T.);
#10166=EDGE_CURVE('',#7689,#7687,#837,.T.);
#10167=EDGE_CURVE('',#7690,#7688,#838,.T.);
#10168=EDGE_CURVE('',#7691,#7664,#839,.T.);
#10169=EDGE_CURVE('',#7660,#7691,#840,.T.);
#10170=EDGE_CURVE('',#7692,#7632,#841,.T.);
#10171=EDGE_CURVE('',#7692,#7690,#842,.T.);
#10172=EDGE_CURVE('',#7632,#7693,#2211,.T.);
#10173=EDGE_CURVE('',#7693,#7631,#2212,.T.);
#10174=EDGE_CURVE('',#7631,#7694,#843,.T.);
#10175=EDGE_CURVE('',#7694,#7692,#2213,.T.);
#10176=EDGE_CURVE('',#7694,#7689,#844,.T.);
#10177=EDGE_CURVE('',#7663,#7695,#845,.T.);
#10178=EDGE_CURVE('',#7695,#7659,#846,.T.);
#10179=EDGE_CURVE('',#7696,#7697,#1364,.T.);
#10180=EDGE_CURVE('',#7698,#7696,#5112,.T.);
#10181=EDGE_CURVE('',#7699,#7698,#5113,.T.);
#10182=EDGE_CURVE('',#7697,#7699,#5114,.T.);
#10183=EDGE_CURVE('',#7699,#7700,#2214,.T.);
#10184=EDGE_CURVE('',#7698,#7700,#5115,.T.);
#10185=EDGE_CURVE('',#7701,#7696,#1365,.T.);
#10186=EDGE_CURVE('',#7700,#7701,#5116,.T.);
#10187=EDGE_CURVE('',#7702,#7701,#2215,.T.);
#10188=EDGE_CURVE('',#7702,#7703,#5117,.T.);
#10189=EDGE_CURVE('',#7703,#7704,#2216,.T.);
#10190=EDGE_CURVE('',#7704,#7705,#5118,.T.);
#10191=EDGE_CURVE('',#7706,#7705,#2217,.T.);
#10192=EDGE_CURVE('',#7706,#7707,#5119,.T.);
#10193=EDGE_CURVE('',#7707,#7708,#2218,.T.);
#10194=EDGE_CURVE('',#7708,#7709,#5120,.T.);
#10195=EDGE_CURVE('',#7710,#7709,#2219,.T.);
#10196=EDGE_CURVE('',#7710,#7711,#5121,.T.);
#10197=EDGE_CURVE('',#7711,#7712,#2220,.T.);
#10198=EDGE_CURVE('',#7712,#7713,#5122,.T.);
#10199=EDGE_CURVE('',#7714,#7713,#2221,.T.);
#10200=EDGE_CURVE('',#7714,#7715,#5123,.T.);
#10201=EDGE_CURVE('',#7715,#7716,#2222,.T.);
#10202=EDGE_CURVE('',#7716,#7717,#5124,.T.);
#10203=EDGE_CURVE('',#7718,#7717,#2223,.T.);
#10204=EDGE_CURVE('',#7718,#7719,#5125,.T.);
#10205=EDGE_CURVE('',#7719,#7720,#2224,.T.);
#10206=EDGE_CURVE('',#7720,#7721,#5126,.T.);
#10207=EDGE_CURVE('',#7722,#7721,#2225,.T.);
#10208=EDGE_CURVE('',#7722,#7723,#5127,.T.);
#10209=EDGE_CURVE('',#7723,#7724,#2226,.T.);
#10210=EDGE_CURVE('',#7724,#7725,#5128,.T.);
#10211=EDGE_CURVE('',#7726,#7725,#2227,.T.);
#10212=EDGE_CURVE('',#7726,#7727,#5129,.T.);
#10213=EDGE_CURVE('',#7727,#7728,#2228,.T.);
#10214=EDGE_CURVE('',#7728,#7729,#5130,.T.);
#10215=EDGE_CURVE('',#7730,#7729,#2229,.T.);
#10216=EDGE_CURVE('',#7730,#7731,#5131,.T.);
#10217=EDGE_CURVE('',#7731,#7732,#2230,.T.);
#10218=EDGE_CURVE('',#7732,#7733,#5132,.T.);
#10219=EDGE_CURVE('',#7734,#7733,#2231,.T.);
#10220=EDGE_CURVE('',#7734,#7735,#5133,.T.);
#10221=EDGE_CURVE('',#7735,#7736,#2232,.T.);
#10222=EDGE_CURVE('',#7736,#7737,#5134,.T.);
#10223=EDGE_CURVE('',#7738,#7737,#2233,.T.);
#10224=EDGE_CURVE('',#7738,#7739,#5135,.T.);
#10225=EDGE_CURVE('',#7739,#7740,#2234,.T.);
#10226=EDGE_CURVE('',#7740,#7741,#5136,.T.);
#10227=EDGE_CURVE('',#7742,#7741,#2235,.T.);
#10228=EDGE_CURVE('',#7742,#7743,#5137,.T.);
#10229=EDGE_CURVE('',#7743,#7744,#2236,.T.);
#10230=EDGE_CURVE('',#7744,#7745,#5138,.T.);
#10231=EDGE_CURVE('',#7746,#7745,#2237,.T.);
#10232=EDGE_CURVE('',#7746,#7747,#5139,.T.);
#10233=EDGE_CURVE('',#7747,#7748,#2238,.T.);
#10234=EDGE_CURVE('',#7748,#7749,#5140,.T.);
#10235=EDGE_CURVE('',#7750,#7749,#2239,.T.);
#10236=EDGE_CURVE('',#7750,#7751,#5141,.T.);
#10237=EDGE_CURVE('',#7751,#7752,#2240,.T.);
#10238=EDGE_CURVE('',#7752,#7753,#5142,.T.);
#10239=EDGE_CURVE('',#7754,#7753,#2241,.T.);
#10240=EDGE_CURVE('',#7754,#7755,#5143,.T.);
#10241=EDGE_CURVE('',#7755,#7756,#2242,.T.);
#10242=EDGE_CURVE('',#7756,#7757,#5144,.T.);
#10243=EDGE_CURVE('',#7757,#7757,#2243,.T.);
#10244=EDGE_CURVE('',#7756,#7758,#2244,.T.);
#10245=EDGE_CURVE('',#7758,#7759,#5145,.T.);
#10246=EDGE_CURVE('',#7760,#7759,#2245,.T.);
#10247=EDGE_CURVE('',#7760,#7761,#5146,.T.);
#10248=EDGE_CURVE('',#7761,#7762,#2246,.T.);
#10249=EDGE_CURVE('',#7762,#7763,#5147,.T.);
#10250=EDGE_CURVE('',#7764,#7763,#2247,.T.);
#10251=EDGE_CURVE('',#7764,#7765,#5148,.T.);
#10252=EDGE_CURVE('',#7765,#7766,#2248,.T.);
#10253=EDGE_CURVE('',#7766,#7767,#5149,.T.);
#10254=EDGE_CURVE('',#7768,#7767,#2249,.T.);
#10255=EDGE_CURVE('',#7768,#7769,#5150,.T.);
#10256=EDGE_CURVE('',#7769,#7770,#2250,.T.);
#10257=EDGE_CURVE('',#7770,#7771,#5151,.T.);
#10258=EDGE_CURVE('',#7772,#7771,#2251,.T.);
#10259=EDGE_CURVE('',#7772,#7773,#5152,.T.);
#10260=EDGE_CURVE('',#7773,#7774,#2252,.T.);
#10261=EDGE_CURVE('',#7774,#7775,#5153,.T.);
#10262=EDGE_CURVE('',#7776,#7775,#2253,.T.);
#10263=EDGE_CURVE('',#7776,#7777,#5154,.T.);
#10264=EDGE_CURVE('',#7777,#7778,#2254,.T.);
#10265=EDGE_CURVE('',#7778,#7779,#5155,.T.);
#10266=EDGE_CURVE('',#7780,#7779,#2255,.T.);
#10267=EDGE_CURVE('',#7780,#7781,#5156,.T.);
#10268=EDGE_CURVE('',#7781,#7782,#2256,.T.);
#10269=EDGE_CURVE('',#7782,#7783,#5157,.T.);
#10270=EDGE_CURVE('',#7784,#7783,#2257,.T.);
#10271=EDGE_CURVE('',#7784,#7785,#5158,.T.);
#10272=EDGE_CURVE('',#7785,#7786,#2258,.T.);
#10273=EDGE_CURVE('',#7786,#7787,#5159,.T.);
#10274=EDGE_CURVE('',#7788,#7787,#2259,.T.);
#10275=EDGE_CURVE('',#7788,#7789,#5160,.T.);
#10276=EDGE_CURVE('',#7789,#7790,#2260,.T.);
#10277=EDGE_CURVE('',#7790,#7791,#5161,.T.);
#10278=EDGE_CURVE('',#7792,#7791,#2261,.T.);
#10279=EDGE_CURVE('',#7792,#7793,#5162,.T.);
#10280=EDGE_CURVE('',#7793,#7794,#2262,.T.);
#10281=EDGE_CURVE('',#7794,#7795,#5163,.T.);
#10282=EDGE_CURVE('',#7796,#7795,#2263,.T.);
#10283=EDGE_CURVE('',#7796,#7797,#5164,.T.);
#10284=EDGE_CURVE('',#7797,#7798,#2264,.T.);
#10285=EDGE_CURVE('',#7798,#7799,#5165,.T.);
#10286=EDGE_CURVE('',#7800,#7799,#2265,.T.);
#10287=EDGE_CURVE('',#7800,#7801,#5166,.T.);
#10288=EDGE_CURVE('',#7801,#7802,#2266,.T.);
#10289=EDGE_CURVE('',#7802,#7803,#5167,.T.);
#10290=EDGE_CURVE('',#7804,#7803,#2267,.T.);
#10291=EDGE_CURVE('',#7804,#7805,#5168,.T.);
#10292=EDGE_CURVE('',#7805,#7806,#2268,.T.);
#10293=EDGE_CURVE('',#7806,#7807,#5169,.T.);
#10294=EDGE_CURVE('',#7808,#7807,#2269,.T.);
#10295=EDGE_CURVE('',#7808,#7809,#5170,.T.);
#10296=EDGE_CURVE('',#7809,#7810,#2270,.T.);
#10297=EDGE_CURVE('',#7810,#7811,#5171,.T.);
#10298=EDGE_CURVE('',#7812,#7811,#2271,.T.);
#10299=EDGE_CURVE('',#7812,#7813,#5172,.T.);
#10300=EDGE_CURVE('',#7813,#7814,#2272,.T.);
#10301=EDGE_CURVE('',#7814,#7815,#5173,.T.);
#10302=EDGE_CURVE('',#7816,#7815,#2273,.T.);
#10303=EDGE_CURVE('',#7816,#7817,#5174,.T.);
#10304=EDGE_CURVE('',#7817,#7818,#2274,.T.);
#10305=EDGE_CURVE('',#7818,#7819,#5175,.T.);
#10306=EDGE_CURVE('',#7697,#7819,#2275,.T.);
#10307=EDGE_CURVE('',#7820,#7702,#1366,.T.);
#10308=EDGE_CURVE('',#7821,#7820,#5176,.T.);
#10309=EDGE_CURVE('',#7703,#7821,#5177,.T.);
#10310=EDGE_CURVE('',#7821,#7704,#5178,.T.);
#10311=EDGE_CURVE('',#7705,#7820,#1367,.T.);
#10312=EDGE_CURVE('',#7822,#7706,#1368,.T.);
#10313=EDGE_CURVE('',#7823,#7822,#5179,.T.);
#10314=EDGE_CURVE('',#7707,#7823,#5180,.T.);
#10315=EDGE_CURVE('',#7823,#7708,#5181,.T.);
#10316=EDGE_CURVE('',#7709,#7822,#1369,.T.);
#10317=EDGE_CURVE('',#7824,#7710,#1370,.T.);
#10318=EDGE_CURVE('',#7825,#7824,#5182,.T.);
#10319=EDGE_CURVE('',#7711,#7825,#5183,.T.);
#10320=EDGE_CURVE('',#7825,#7712,#5184,.T.);
#10321=EDGE_CURVE('',#7713,#7824,#1371,.T.);
#10322=EDGE_CURVE('',#7826,#7714,#1372,.T.);
#10323=EDGE_CURVE('',#7827,#7826,#5185,.T.);
#10324=EDGE_CURVE('',#7715,#7827,#5186,.T.);
#10325=EDGE_CURVE('',#7827,#7716,#5187,.T.);
#10326=EDGE_CURVE('',#7717,#7826,#1373,.T.);
#10327=EDGE_CURVE('',#7828,#7718,#1374,.T.);
#10328=EDGE_CURVE('',#7829,#7828,#5188,.T.);
#10329=EDGE_CURVE('',#7719,#7829,#5189,.T.);
#10330=EDGE_CURVE('',#7829,#7720,#5190,.T.);
#10331=EDGE_CURVE('',#7721,#7828,#1375,.T.);
#10332=EDGE_CURVE('',#7830,#7722,#1376,.T.);
#10333=EDGE_CURVE('',#7831,#7830,#5191,.T.);
#10334=EDGE_CURVE('',#7723,#7831,#5192,.T.);
#10335=EDGE_CURVE('',#7831,#7724,#5193,.T.);
#10336=EDGE_CURVE('',#7725,#7830,#1377,.T.);
#10337=EDGE_CURVE('',#7832,#7726,#1378,.T.);
#10338=EDGE_CURVE('',#7833,#7832,#5194,.T.);
#10339=EDGE_CURVE('',#7727,#7833,#5195,.T.);
#10340=EDGE_CURVE('',#7833,#7728,#5196,.T.);
#10341=EDGE_CURVE('',#7729,#7832,#1379,.T.);
#10342=EDGE_CURVE('',#7834,#7730,#1380,.T.);
#10343=EDGE_CURVE('',#7835,#7834,#5197,.T.);
#10344=EDGE_CURVE('',#7731,#7835,#5198,.T.);
#10345=EDGE_CURVE('',#7835,#7732,#5199,.T.);
#10346=EDGE_CURVE('',#7733,#7834,#1381,.T.);
#10347=EDGE_CURVE('',#7836,#7734,#1382,.T.);
#10348=EDGE_CURVE('',#7837,#7836,#5200,.T.);
#10349=EDGE_CURVE('',#7735,#7837,#5201,.T.);
#10350=EDGE_CURVE('',#7837,#7736,#5202,.T.);
#10351=EDGE_CURVE('',#7737,#7836,#1383,.T.);
#10352=EDGE_CURVE('',#7838,#7738,#1384,.T.);
#10353=EDGE_CURVE('',#7839,#7838,#5203,.T.);
#10354=EDGE_CURVE('',#7739,#7839,#5204,.T.);
#10355=EDGE_CURVE('',#7839,#7740,#5205,.T.);
#10356=EDGE_CURVE('',#7741,#7838,#1385,.T.);
#10357=EDGE_CURVE('',#7840,#7742,#1386,.T.);
#10358=EDGE_CURVE('',#7841,#7840,#5206,.T.);
#10359=EDGE_CURVE('',#7743,#7841,#5207,.T.);
#10360=EDGE_CURVE('',#7841,#7744,#5208,.T.);
#10361=EDGE_CURVE('',#7745,#7840,#1387,.T.);
#10362=EDGE_CURVE('',#7842,#7746,#1388,.T.);
#10363=EDGE_CURVE('',#7843,#7842,#5209,.T.);
#10364=EDGE_CURVE('',#7747,#7843,#5210,.T.);
#10365=EDGE_CURVE('',#7843,#7748,#5211,.T.);
#10366=EDGE_CURVE('',#7749,#7842,#1389,.T.);
#10367=EDGE_CURVE('',#7844,#7750,#1390,.T.);
#10368=EDGE_CURVE('',#7845,#7844,#5212,.T.);
#10369=EDGE_CURVE('',#7751,#7845,#5213,.T.);
#10370=EDGE_CURVE('',#7845,#7752,#5214,.T.);
#10371=EDGE_CURVE('',#7753,#7844,#1391,.T.);
#10372=EDGE_CURVE('',#7846,#7754,#1392,.T.);
#10373=EDGE_CURVE('',#7847,#7846,#5215,.T.);
#10374=EDGE_CURVE('',#7755,#7847,#5216,.T.);
#10375=EDGE_CURVE('',#7847,#7758,#5217,.T.);
#10376=EDGE_CURVE('',#7759,#7846,#1393,.T.);
#10377=EDGE_CURVE('',#7848,#7760,#1394,.T.);
#10378=EDGE_CURVE('',#7849,#7848,#5218,.T.);
#10379=EDGE_CURVE('',#7761,#7849,#5219,.T.);
#10380=EDGE_CURVE('',#7849,#7762,#5220,.T.);
#10381=EDGE_CURVE('',#7763,#7848,#1395,.T.);
#10382=EDGE_CURVE('',#7850,#7764,#1396,.T.);
#10383=EDGE_CURVE('',#7851,#7850,#5221,.T.);
#10384=EDGE_CURVE('',#7765,#7851,#5222,.T.);
#10385=EDGE_CURVE('',#7851,#7766,#5223,.T.);
#10386=EDGE_CURVE('',#7767,#7850,#1397,.T.);
#10387=EDGE_CURVE('',#7852,#7768,#1398,.T.);
#10388=EDGE_CURVE('',#7853,#7852,#5224,.T.);
#10389=EDGE_CURVE('',#7769,#7853,#5225,.T.);
#10390=EDGE_CURVE('',#7853,#7770,#5226,.T.);
#10391=EDGE_CURVE('',#7771,#7852,#1399,.T.);
#10392=EDGE_CURVE('',#7854,#7772,#1400,.T.);
#10393=EDGE_CURVE('',#7855,#7854,#5227,.T.);
#10394=EDGE_CURVE('',#7773,#7855,#5228,.T.);
#10395=EDGE_CURVE('',#7855,#7774,#5229,.T.);
#10396=EDGE_CURVE('',#7775,#7854,#1401,.T.);
#10397=EDGE_CURVE('',#7856,#7776,#1402,.T.);
#10398=EDGE_CURVE('',#7857,#7856,#5230,.T.);
#10399=EDGE_CURVE('',#7777,#7857,#5231,.T.);
#10400=EDGE_CURVE('',#7857,#7778,#5232,.T.);
#10401=EDGE_CURVE('',#7779,#7856,#1403,.T.);
#10402=EDGE_CURVE('',#7858,#7780,#1404,.T.);
#10403=EDGE_CURVE('',#7859,#7858,#5233,.T.);
#10404=EDGE_CURVE('',#7781,#7859,#5234,.T.);
#10405=EDGE_CURVE('',#7859,#7782,#5235,.T.);
#10406=EDGE_CURVE('',#7783,#7858,#1405,.T.);
#10407=EDGE_CURVE('',#7860,#7784,#1406,.T.);
#10408=EDGE_CURVE('',#7861,#7860,#5236,.T.);
#10409=EDGE_CURVE('',#7785,#7861,#5237,.T.);
#10410=EDGE_CURVE('',#7861,#7786,#5238,.T.);
#10411=EDGE_CURVE('',#7787,#7860,#1407,.T.);
#10412=EDGE_CURVE('',#7862,#7788,#1408,.T.);
#10413=EDGE_CURVE('',#7863,#7862,#5239,.T.);
#10414=EDGE_CURVE('',#7789,#7863,#5240,.T.);
#10415=EDGE_CURVE('',#7863,#7790,#5241,.T.);
#10416=EDGE_CURVE('',#7791,#7862,#1409,.T.);
#10417=EDGE_CURVE('',#7864,#7792,#1410,.T.);
#10418=EDGE_CURVE('',#7865,#7864,#5242,.T.);
#10419=EDGE_CURVE('',#7793,#7865,#5243,.T.);
#10420=EDGE_CURVE('',#7865,#7794,#5244,.T.);
#10421=EDGE_CURVE('',#7795,#7864,#1411,.T.);
#10422=EDGE_CURVE('',#7866,#7796,#1412,.T.);
#10423=EDGE_CURVE('',#7867,#7866,#5245,.T.);
#10424=EDGE_CURVE('',#7797,#7867,#5246,.T.);
#10425=EDGE_CURVE('',#7867,#7798,#5247,.T.);
#10426=EDGE_CURVE('',#7799,#7866,#1413,.T.);
#10427=EDGE_CURVE('',#7868,#7800,#1414,.T.);
#10428=EDGE_CURVE('',#7869,#7868,#5248,.T.);
#10429=EDGE_CURVE('',#7801,#7869,#5249,.T.);
#10430=EDGE_CURVE('',#7869,#7802,#5250,.T.);
#10431=EDGE_CURVE('',#7803,#7868,#1415,.T.);
#10432=EDGE_CURVE('',#7870,#7804,#1416,.T.);
#10433=EDGE_CURVE('',#7871,#7870,#5251,.T.);
#10434=EDGE_CURVE('',#7805,#7871,#5252,.T.);
#10435=EDGE_CURVE('',#7871,#7806,#5253,.T.);
#10436=EDGE_CURVE('',#7807,#7870,#1417,.T.);
#10437=EDGE_CURVE('',#7872,#7808,#1418,.T.);
#10438=EDGE_CURVE('',#7873,#7872,#5254,.T.);
#10439=EDGE_CURVE('',#7809,#7873,#5255,.T.);
#10440=EDGE_CURVE('',#7873,#7810,#5256,.T.);
#10441=EDGE_CURVE('',#7811,#7872,#1419,.T.);
#10442=EDGE_CURVE('',#7874,#7812,#1420,.T.);
#10443=EDGE_CURVE('',#7875,#7874,#5257,.T.);
#10444=EDGE_CURVE('',#7813,#7875,#5258,.T.);
#10445=EDGE_CURVE('',#7875,#7814,#5259,.T.);
#10446=EDGE_CURVE('',#7815,#7874,#1421,.T.);
#10447=EDGE_CURVE('',#7876,#7816,#1422,.T.);
#10448=EDGE_CURVE('',#7877,#7876,#5260,.T.);
#10449=EDGE_CURVE('',#7817,#7877,#5261,.T.);
#10450=EDGE_CURVE('',#7877,#7818,#5262,.T.);
#10451=EDGE_CURVE('',#7819,#7876,#1423,.T.);
#10452=EDGE_CURVE('',#7878,#7878,#2276,.T.);
#10453=EDGE_CURVE('',#7693,#7878,#5263,.T.);
#10454=EDGE_CURVE('',#7695,#7691,#2277,.T.);
#10455=EDGE_CURVE('',#7879,#7879,#2278,.T.);
#10456=EDGE_CURVE('',#7757,#7879,#5264,.T.);
#10457=EDGE_CURVE('',#7880,#7880,#2279,.T.);
#10458=EDGE_CURVE('',#7880,#7846,#5265,.T.);
#14855=ORIENTED_EDGE('',*,*,#10079,.F.);
#14856=ORIENTED_EDGE('',*,*,#10080,.T.);
#14857=ORIENTED_EDGE('',*,*,#10081,.T.);
#14858=ORIENTED_EDGE('',*,*,#10082,.T.);
#14859=ORIENTED_EDGE('',*,*,#10083,.F.);
#14860=ORIENTED_EDGE('',*,*,#10084,.T.);
#14861=ORIENTED_EDGE('',*,*,#10079,.T.);
#14862=ORIENTED_EDGE('',*,*,#10085,.T.);
#14863=ORIENTED_EDGE('',*,*,#10086,.F.);
#14864=ORIENTED_EDGE('',*,*,#10087,.T.);
#14865=ORIENTED_EDGE('',*,*,#10083,.T.);
#14866=ORIENTED_EDGE('',*,*,#10088,.T.);
#14867=ORIENTED_EDGE('',*,*,#10089,.F.);
#14868=ORIENTED_EDGE('',*,*,#10090,.T.);
#14869=ORIENTED_EDGE('',*,*,#10086,.T.);
#14870=ORIENTED_EDGE('',*,*,#10091,.T.);
#14871=ORIENTED_EDGE('',*,*,#10092,.F.);
#14872=ORIENTED_EDGE('',*,*,#10093,.T.);
#14873=ORIENTED_EDGE('',*,*,#10089,.T.);
#14874=ORIENTED_EDGE('',*,*,#10094,.T.);
#14875=ORIENTED_EDGE('',*,*,#10095,.F.);
#14876=ORIENTED_EDGE('',*,*,#10096,.T.);
#14877=ORIENTED_EDGE('',*,*,#10092,.T.);
#14878=ORIENTED_EDGE('',*,*,#10097,.T.);
#14879=ORIENTED_EDGE('',*,*,#10098,.F.);
#14880=ORIENTED_EDGE('',*,*,#10099,.T.);
#14881=ORIENTED_EDGE('',*,*,#10095,.T.);
#14882=ORIENTED_EDGE('',*,*,#10100,.T.);
#14883=ORIENTED_EDGE('',*,*,#10101,.F.);
#14884=ORIENTED_EDGE('',*,*,#10102,.T.);
#14885=ORIENTED_EDGE('',*,*,#10098,.T.);
#14886=ORIENTED_EDGE('',*,*,#10103,.T.);
#14887=ORIENTED_EDGE('',*,*,#10104,.F.);
#14888=ORIENTED_EDGE('',*,*,#10105,.T.);
#14889=ORIENTED_EDGE('',*,*,#10101,.T.);
#14890=ORIENTED_EDGE('',*,*,#10106,.T.);
#14891=ORIENTED_EDGE('',*,*,#10107,.F.);
#14892=ORIENTED_EDGE('',*,*,#10108,.T.);
#14893=ORIENTED_EDGE('',*,*,#10104,.T.);
#14894=ORIENTED_EDGE('',*,*,#10109,.T.);
#14895=ORIENTED_EDGE('',*,*,#10110,.F.);
#14896=ORIENTED_EDGE('',*,*,#10111,.T.);
#14897=ORIENTED_EDGE('',*,*,#10107,.T.);
#14898=ORIENTED_EDGE('',*,*,#10112,.T.);
#14899=ORIENTED_EDGE('',*,*,#10113,.F.);
#14900=ORIENTED_EDGE('',*,*,#10114,.T.);
#14901=ORIENTED_EDGE('',*,*,#10110,.T.);
#14902=ORIENTED_EDGE('',*,*,#10115,.T.);
#14903=ORIENTED_EDGE('',*,*,#10116,.F.);
#14904=ORIENTED_EDGE('',*,*,#10117,.T.);
#14905=ORIENTED_EDGE('',*,*,#10113,.T.);
#14906=ORIENTED_EDGE('',*,*,#10118,.T.);
#14907=ORIENTED_EDGE('',*,*,#10119,.F.);
#14908=ORIENTED_EDGE('',*,*,#10120,.T.);
#14909=ORIENTED_EDGE('',*,*,#10116,.T.);
#14910=ORIENTED_EDGE('',*,*,#10121,.T.);
#14911=ORIENTED_EDGE('',*,*,#10122,.F.);
#14912=ORIENTED_EDGE('',*,*,#10123,.T.);
#14913=ORIENTED_EDGE('',*,*,#10119,.T.);
#14914=ORIENTED_EDGE('',*,*,#10124,.T.);
#14915=ORIENTED_EDGE('',*,*,#10125,.F.);
#14916=ORIENTED_EDGE('',*,*,#10126,.T.);
#14917=ORIENTED_EDGE('',*,*,#10127,.F.);
#14918=ORIENTED_EDGE('',*,*,#10128,.F.);
#14919=ORIENTED_EDGE('',*,*,#10129,.F.);
#14920=ORIENTED_EDGE('',*,*,#10130,.T.);
#14921=ORIENTED_EDGE('',*,*,#10125,.T.);
#14922=ORIENTED_EDGE('',*,*,#10131,.F.);
#14923=ORIENTED_EDGE('',*,*,#10132,.F.);
#14924=ORIENTED_EDGE('',*,*,#10133,.T.);
#14925=ORIENTED_EDGE('',*,*,#10129,.T.);
#14926=ORIENTED_EDGE('',*,*,#10134,.F.);
#14927=ORIENTED_EDGE('',*,*,#10135,.F.);
#14928=ORIENTED_EDGE('',*,*,#10136,.T.);
#14929=ORIENTED_EDGE('',*,*,#10132,.T.);
#14930=ORIENTED_EDGE('',*,*,#10137,.F.);
#14931=ORIENTED_EDGE('',*,*,#10138,.F.);
#14932=ORIENTED_EDGE('',*,*,#10139,.T.);
#14933=ORIENTED_EDGE('',*,*,#10135,.T.);
#14934=ORIENTED_EDGE('',*,*,#10140,.F.);
#14935=ORIENTED_EDGE('',*,*,#10141,.F.);
#14936=ORIENTED_EDGE('',*,*,#10142,.T.);
#14937=ORIENTED_EDGE('',*,*,#10138,.T.);
#14938=ORIENTED_EDGE('',*,*,#10143,.F.);
#14939=ORIENTED_EDGE('',*,*,#10144,.F.);
#14940=ORIENTED_EDGE('',*,*,#10145,.T.);
#14941=ORIENTED_EDGE('',*,*,#10141,.T.);
#14942=ORIENTED_EDGE('',*,*,#10146,.F.);
#14943=ORIENTED_EDGE('',*,*,#10147,.F.);
#14944=ORIENTED_EDGE('',*,*,#10148,.T.);
#14945=ORIENTED_EDGE('',*,*,#10144,.T.);
#14946=ORIENTED_EDGE('',*,*,#10149,.F.);
#14947=ORIENTED_EDGE('',*,*,#10150,.F.);
#14948=ORIENTED_EDGE('',*,*,#10151,.T.);
#14949=ORIENTED_EDGE('',*,*,#10147,.T.);
#14950=ORIENTED_EDGE('',*,*,#10152,.F.);
#14951=ORIENTED_EDGE('',*,*,#10153,.F.);
#14952=ORIENTED_EDGE('',*,*,#10154,.T.);
#14953=ORIENTED_EDGE('',*,*,#10150,.T.);
#14954=ORIENTED_EDGE('',*,*,#10155,.F.);
#14955=ORIENTED_EDGE('',*,*,#10156,.F.);
#14956=ORIENTED_EDGE('',*,*,#10157,.T.);
#14957=ORIENTED_EDGE('',*,*,#10153,.T.);
#14958=ORIENTED_EDGE('',*,*,#10158,.F.);
#14959=ORIENTED_EDGE('',*,*,#10159,.F.);
#14960=ORIENTED_EDGE('',*,*,#10160,.T.);
#14961=ORIENTED_EDGE('',*,*,#10156,.T.);
#14962=ORIENTED_EDGE('',*,*,#10161,.F.);
#14963=ORIENTED_EDGE('',*,*,#10162,.F.);
#14964=ORIENTED_EDGE('',*,*,#10163,.T.);
#14965=ORIENTED_EDGE('',*,*,#10159,.T.);
#14966=ORIENTED_EDGE('',*,*,#10164,.F.);
#14967=ORIENTED_EDGE('',*,*,#10165,.F.);
#14968=ORIENTED_EDGE('',*,*,#10166,.T.);
#14969=ORIENTED_EDGE('',*,*,#10162,.T.);
#14970=ORIENTED_EDGE('',*,*,#10167,.F.);
#14971=ORIENTED_EDGE('',*,*,#10168,.F.);
#14972=ORIENTED_EDGE('',*,*,#10169,.F.);
#14973=ORIENTED_EDGE('',*,*,#10124,.F.);
#14974=ORIENTED_EDGE('',*,*,#10121,.F.);
#14975=ORIENTED_EDGE('',*,*,#10118,.F.);
#14976=ORIENTED_EDGE('',*,*,#10115,.F.);
#14977=ORIENTED_EDGE('',*,*,#10112,.F.);
#14978=ORIENTED_EDGE('',*,*,#10109,.F.);
#14979=ORIENTED_EDGE('',*,*,#10106,.F.);
#14980=ORIENTED_EDGE('',*,*,#10103,.F.);
#14981=ORIENTED_EDGE('',*,*,#10100,.F.);
#14982=ORIENTED_EDGE('',*,*,#10097,.F.);
#14983=ORIENTED_EDGE('',*,*,#10094,.F.);
#14984=ORIENTED_EDGE('',*,*,#10091,.F.);
#14985=ORIENTED_EDGE('',*,*,#10088,.F.);
#14986=ORIENTED_EDGE('',*,*,#10085,.F.);
#14987=ORIENTED_EDGE('',*,*,#10082,.F.);
#14988=ORIENTED_EDGE('',*,*,#10170,.F.);
#14989=ORIENTED_EDGE('',*,*,#10171,.T.);
#14990=ORIENTED_EDGE('',*,*,#10167,.T.);
#14991=ORIENTED_EDGE('',*,*,#10164,.T.);
#14992=ORIENTED_EDGE('',*,*,#10161,.T.);
#14993=ORIENTED_EDGE('',*,*,#10158,.T.);
#14994=ORIENTED_EDGE('',*,*,#10155,.T.);
#14995=ORIENTED_EDGE('',*,*,#10152,.T.);
#14996=ORIENTED_EDGE('',*,*,#10149,.T.);
#14997=ORIENTED_EDGE('',*,*,#10146,.T.);
#14998=ORIENTED_EDGE('',*,*,#10143,.T.);
#14999=ORIENTED_EDGE('',*,*,#10140,.T.);
#15000=ORIENTED_EDGE('',*,*,#10137,.T.);
#15001=ORIENTED_EDGE('',*,*,#10134,.T.);
#15002=ORIENTED_EDGE('',*,*,#10131,.T.);
#15003=ORIENTED_EDGE('',*,*,#10128,.T.);
#15004=ORIENTED_EDGE('',*,*,#10172,.T.);
#15005=ORIENTED_EDGE('',*,*,#10173,.T.);
#15006=ORIENTED_EDGE('',*,*,#10174,.T.);
#15007=ORIENTED_EDGE('',*,*,#10175,.T.);
#15008=ORIENTED_EDGE('',*,*,#10170,.T.);
#15009=ORIENTED_EDGE('',*,*,#10165,.T.);
#15010=ORIENTED_EDGE('',*,*,#10171,.F.);
#15011=ORIENTED_EDGE('',*,*,#10175,.F.);
#15012=ORIENTED_EDGE('',*,*,#10176,.T.);
#15013=ORIENTED_EDGE('',*,*,#10177,.F.);
#15014=ORIENTED_EDGE('',*,*,#10126,.F.);
#15015=ORIENTED_EDGE('',*,*,#10130,.F.);
#15016=ORIENTED_EDGE('',*,*,#10133,.F.);
#15017=ORIENTED_EDGE('',*,*,#10136,.F.);
#15018=ORIENTED_EDGE('',*,*,#10139,.F.);
#15019=ORIENTED_EDGE('',*,*,#10142,.F.);
#15020=ORIENTED_EDGE('',*,*,#10145,.F.);
#15021=ORIENTED_EDGE('',*,*,#10148,.F.);
#15022=ORIENTED_EDGE('',*,*,#10151,.F.);
#15023=ORIENTED_EDGE('',*,*,#10154,.F.);
#15024=ORIENTED_EDGE('',*,*,#10157,.F.);
#15025=ORIENTED_EDGE('',*,*,#10160,.F.);
#15026=ORIENTED_EDGE('',*,*,#10163,.F.);
#15027=ORIENTED_EDGE('',*,*,#10166,.F.);
#15028=ORIENTED_EDGE('',*,*,#10176,.F.);
#15029=ORIENTED_EDGE('',*,*,#10174,.F.);
#15030=ORIENTED_EDGE('',*,*,#10080,.F.);
#15031=ORIENTED_EDGE('',*,*,#10084,.F.);
#15032=ORIENTED_EDGE('',*,*,#10087,.F.);
#15033=ORIENTED_EDGE('',*,*,#10090,.F.);
#15034=ORIENTED_EDGE('',*,*,#10093,.F.);
#15035=ORIENTED_EDGE('',*,*,#10096,.F.);
#15036=ORIENTED_EDGE('',*,*,#10099,.F.);
#15037=ORIENTED_EDGE('',*,*,#10102,.F.);
#15038=ORIENTED_EDGE('',*,*,#10105,.F.);
#15039=ORIENTED_EDGE('',*,*,#10108,.F.);
#15040=ORIENTED_EDGE('',*,*,#10111,.F.);
#15041=ORIENTED_EDGE('',*,*,#10114,.F.);
#15042=ORIENTED_EDGE('',*,*,#10117,.F.);
#15043=ORIENTED_EDGE('',*,*,#10120,.F.);
#15044=ORIENTED_EDGE('',*,*,#10123,.F.);
#15045=ORIENTED_EDGE('',*,*,#10178,.F.);
#15046=ORIENTED_EDGE('',*,*,#10179,.F.);
#15047=ORIENTED_EDGE('',*,*,#10180,.F.);
#15048=ORIENTED_EDGE('',*,*,#10181,.F.);
#15049=ORIENTED_EDGE('',*,*,#10182,.F.);
#15050=ORIENTED_EDGE('',*,*,#10183,.F.);
#15051=ORIENTED_EDGE('',*,*,#10181,.T.);
#15052=ORIENTED_EDGE('',*,*,#10184,.T.);
#15053=ORIENTED_EDGE('',*,*,#10185,.F.);
#15054=ORIENTED_EDGE('',*,*,#10186,.F.);
#15055=ORIENTED_EDGE('',*,*,#10184,.F.);
#15056=ORIENTED_EDGE('',*,*,#10180,.T.);
#15057=ORIENTED_EDGE('',*,*,#10182,.T.);
#15058=ORIENTED_EDGE('',*,*,#10183,.T.);
#15059=ORIENTED_EDGE('',*,*,#10186,.T.);
#15060=ORIENTED_EDGE('',*,*,#10187,.F.);
#15061=ORIENTED_EDGE('',*,*,#10188,.T.);
#15062=ORIENTED_EDGE('',*,*,#10189,.T.);
#15063=ORIENTED_EDGE('',*,*,#10190,.T.);
#15064=ORIENTED_EDGE('',*,*,#10191,.F.);
#15065=ORIENTED_EDGE('',*,*,#10192,.T.);
#15066=ORIENTED_EDGE('',*,*,#10193,.T.);
#15067=ORIENTED_EDGE('',*,*,#10194,.T.);
#15068=ORIENTED_EDGE('',*,*,#10195,.F.);
#15069=ORIENTED_EDGE('',*,*,#10196,.T.);
#15070=ORIENTED_EDGE('',*,*,#10197,.T.);
#15071=ORIENTED_EDGE('',*,*,#10198,.T.);
#15072=ORIENTED_EDGE('',*,*,#10199,.F.);
#15073=ORIENTED_EDGE('',*,*,#10200,.T.);
#15074=ORIENTED_EDGE('',*,*,#10201,.T.);
#15075=ORIENTED_EDGE('',*,*,#10202,.T.);
#15076=ORIENTED_EDGE('',*,*,#10203,.F.);
#15077=ORIENTED_EDGE('',*,*,#10204,.T.);
#15078=ORIENTED_EDGE('',*,*,#10205,.T.);
#15079=ORIENTED_EDGE('',*,*,#10206,.T.);
#15080=ORIENTED_EDGE('',*,*,#10207,.F.);
#15081=ORIENTED_EDGE('',*,*,#10208,.T.);
#15082=ORIENTED_EDGE('',*,*,#10209,.T.);
#15083=ORIENTED_EDGE('',*,*,#10210,.T.);
#15084=ORIENTED_EDGE('',*,*,#10211,.F.);
#15085=ORIENTED_EDGE('',*,*,#10212,.T.);
#15086=ORIENTED_EDGE('',*,*,#10213,.T.);
#15087=ORIENTED_EDGE('',*,*,#10214,.T.);
#15088=ORIENTED_EDGE('',*,*,#10215,.F.);
#15089=ORIENTED_EDGE('',*,*,#10216,.T.);
#15090=ORIENTED_EDGE('',*,*,#10217,.T.);
#15091=ORIENTED_EDGE('',*,*,#10218,.T.);
#15092=ORIENTED_EDGE('',*,*,#10219,.F.);
#15093=ORIENTED_EDGE('',*,*,#10220,.T.);
#15094=ORIENTED_EDGE('',*,*,#10221,.T.);
#15095=ORIENTED_EDGE('',*,*,#10222,.T.);
#15096=ORIENTED_EDGE('',*,*,#10223,.F.);
#15097=ORIENTED_EDGE('',*,*,#10224,.T.);
#15098=ORIENTED_EDGE('',*,*,#10225,.T.);
#15099=ORIENTED_EDGE('',*,*,#10226,.T.);
#15100=ORIENTED_EDGE('',*,*,#10227,.F.);
#15101=ORIENTED_EDGE('',*,*,#10228,.T.);
#15102=ORIENTED_EDGE('',*,*,#10229,.T.);
#15103=ORIENTED_EDGE('',*,*,#10230,.T.);
#15104=ORIENTED_EDGE('',*,*,#10231,.F.);
#15105=ORIENTED_EDGE('',*,*,#10232,.T.);
#15106=ORIENTED_EDGE('',*,*,#10233,.T.);
#15107=ORIENTED_EDGE('',*,*,#10234,.T.);
#15108=ORIENTED_EDGE('',*,*,#10235,.F.);
#15109=ORIENTED_EDGE('',*,*,#10236,.T.);
#15110=ORIENTED_EDGE('',*,*,#10237,.T.);
#15111=ORIENTED_EDGE('',*,*,#10238,.T.);
#15112=ORIENTED_EDGE('',*,*,#10239,.F.);
#15113=ORIENTED_EDGE('',*,*,#10240,.T.);
#15114=ORIENTED_EDGE('',*,*,#10241,.T.);
#15115=ORIENTED_EDGE('',*,*,#10242,.T.);
#15116=ORIENTED_EDGE('',*,*,#10243,.T.);
#15117=ORIENTED_EDGE('',*,*,#10242,.F.);
#15118=ORIENTED_EDGE('',*,*,#10244,.T.);
#15119=ORIENTED_EDGE('',*,*,#10245,.T.);
#15120=ORIENTED_EDGE('',*,*,#10246,.F.);
#15121=ORIENTED_EDGE('',*,*,#10247,.T.);
#15122=ORIENTED_EDGE('',*,*,#10248,.T.);
#15123=ORIENTED_EDGE('',*,*,#10249,.T.);
#15124=ORIENTED_EDGE('',*,*,#10250,.F.);
#15125=ORIENTED_EDGE('',*,*,#10251,.T.);
#15126=ORIENTED_EDGE('',*,*,#10252,.T.);
#15127=ORIENTED_EDGE('',*,*,#10253,.T.);
#15128=ORIENTED_EDGE('',*,*,#10254,.F.);
#15129=ORIENTED_EDGE('',*,*,#10255,.T.);
#15130=ORIENTED_EDGE('',*,*,#10256,.T.);
#15131=ORIENTED_EDGE('',*,*,#10257,.T.);
#15132=ORIENTED_EDGE('',*,*,#10258,.F.);
#15133=ORIENTED_EDGE('',*,*,#10259,.T.);
#15134=ORIENTED_EDGE('',*,*,#10260,.T.);
#15135=ORIENTED_EDGE('',*,*,#10261,.T.);
#15136=ORIENTED_EDGE('',*,*,#10262,.F.);
#15137=ORIENTED_EDGE('',*,*,#10263,.T.);
#15138=ORIENTED_EDGE('',*,*,#10264,.T.);
#15139=ORIENTED_EDGE('',*,*,#10265,.T.);
#15140=ORIENTED_EDGE('',*,*,#10266,.F.);
#15141=ORIENTED_EDGE('',*,*,#10267,.T.);
#15142=ORIENTED_EDGE('',*,*,#10268,.T.);
#15143=ORIENTED_EDGE('',*,*,#10269,.T.);
#15144=ORIENTED_EDGE('',*,*,#10270,.F.);
#15145=ORIENTED_EDGE('',*,*,#10271,.T.);
#15146=ORIENTED_EDGE('',*,*,#10272,.T.);
#15147=ORIENTED_EDGE('',*,*,#10273,.T.);
#15148=ORIENTED_EDGE('',*,*,#10274,.F.);
#15149=ORIENTED_EDGE('',*,*,#10275,.T.);
#15150=ORIENTED_EDGE('',*,*,#10276,.T.);
#15151=ORIENTED_EDGE('',*,*,#10277,.T.);
#15152=ORIENTED_EDGE('',*,*,#10278,.F.);
#15153=ORIENTED_EDGE('',*,*,#10279,.T.);
#15154=ORIENTED_EDGE('',*,*,#10280,.T.);
#15155=ORIENTED_EDGE('',*,*,#10281,.T.);
#15156=ORIENTED_EDGE('',*,*,#10282,.F.);
#15157=ORIENTED_EDGE('',*,*,#10283,.T.);
#15158=ORIENTED_EDGE('',*,*,#10284,.T.);
#15159=ORIENTED_EDGE('',*,*,#10285,.T.);
#15160=ORIENTED_EDGE('',*,*,#10286,.F.);
#15161=ORIENTED_EDGE('',*,*,#10287,.T.);
#15162=ORIENTED_EDGE('',*,*,#10288,.T.);
#15163=ORIENTED_EDGE('',*,*,#10289,.T.);
#15164=ORIENTED_EDGE('',*,*,#10290,.F.);
#15165=ORIENTED_EDGE('',*,*,#10291,.T.);
#15166=ORIENTED_EDGE('',*,*,#10292,.T.);
#15167=ORIENTED_EDGE('',*,*,#10293,.T.);
#15168=ORIENTED_EDGE('',*,*,#10294,.F.);
#15169=ORIENTED_EDGE('',*,*,#10295,.T.);
#15170=ORIENTED_EDGE('',*,*,#10296,.T.);
#15171=ORIENTED_EDGE('',*,*,#10297,.T.);
#15172=ORIENTED_EDGE('',*,*,#10298,.F.);
#15173=ORIENTED_EDGE('',*,*,#10299,.T.);
#15174=ORIENTED_EDGE('',*,*,#10300,.T.);
#15175=ORIENTED_EDGE('',*,*,#10301,.T.);
#15176=ORIENTED_EDGE('',*,*,#10302,.F.);
#15177=ORIENTED_EDGE('',*,*,#10303,.T.);
#15178=ORIENTED_EDGE('',*,*,#10304,.T.);
#15179=ORIENTED_EDGE('',*,*,#10305,.T.);
#15180=ORIENTED_EDGE('',*,*,#10306,.F.);
#15181=ORIENTED_EDGE('',*,*,#10307,.F.);
#15182=ORIENTED_EDGE('',*,*,#10308,.F.);
#15183=ORIENTED_EDGE('',*,*,#10309,.F.);
#15184=ORIENTED_EDGE('',*,*,#10188,.F.);
#15185=ORIENTED_EDGE('',*,*,#10189,.F.);
#15186=ORIENTED_EDGE('',*,*,#10309,.T.);
#15187=ORIENTED_EDGE('',*,*,#10310,.T.);
#15188=ORIENTED_EDGE('',*,*,#10311,.F.);
#15189=ORIENTED_EDGE('',*,*,#10190,.F.);
#15190=ORIENTED_EDGE('',*,*,#10310,.F.);
#15191=ORIENTED_EDGE('',*,*,#10308,.T.);
#15192=ORIENTED_EDGE('',*,*,#10312,.F.);
#15193=ORIENTED_EDGE('',*,*,#10313,.F.);
#15194=ORIENTED_EDGE('',*,*,#10314,.F.);
#15195=ORIENTED_EDGE('',*,*,#10192,.F.);
#15196=ORIENTED_EDGE('',*,*,#10193,.F.);
#15197=ORIENTED_EDGE('',*,*,#10314,.T.);
#15198=ORIENTED_EDGE('',*,*,#10315,.T.);
#15199=ORIENTED_EDGE('',*,*,#10316,.F.);
#15200=ORIENTED_EDGE('',*,*,#10194,.F.);
#15201=ORIENTED_EDGE('',*,*,#10315,.F.);
#15202=ORIENTED_EDGE('',*,*,#10313,.T.);
#15203=ORIENTED_EDGE('',*,*,#10317,.F.);
#15204=ORIENTED_EDGE('',*,*,#10318,.F.);
#15205=ORIENTED_EDGE('',*,*,#10319,.F.);
#15206=ORIENTED_EDGE('',*,*,#10196,.F.);
#15207=ORIENTED_EDGE('',*,*,#10197,.F.);
#15208=ORIENTED_EDGE('',*,*,#10319,.T.);
#15209=ORIENTED_EDGE('',*,*,#10320,.T.);
#15210=ORIENTED_EDGE('',*,*,#10321,.F.);
#15211=ORIENTED_EDGE('',*,*,#10198,.F.);
#15212=ORIENTED_EDGE('',*,*,#10320,.F.);
#15213=ORIENTED_EDGE('',*,*,#10318,.T.);
#15214=ORIENTED_EDGE('',*,*,#10322,.F.);
#15215=ORIENTED_EDGE('',*,*,#10323,.F.);
#15216=ORIENTED_EDGE('',*,*,#10324,.F.);
#15217=ORIENTED_EDGE('',*,*,#10200,.F.);
#15218=ORIENTED_EDGE('',*,*,#10201,.F.);
#15219=ORIENTED_EDGE('',*,*,#10324,.T.);
#15220=ORIENTED_EDGE('',*,*,#10325,.T.);
#15221=ORIENTED_EDGE('',*,*,#10326,.F.);
#15222=ORIENTED_EDGE('',*,*,#10202,.F.);
#15223=ORIENTED_EDGE('',*,*,#10325,.F.);
#15224=ORIENTED_EDGE('',*,*,#10323,.T.);
#15225=ORIENTED_EDGE('',*,*,#10327,.F.);
#15226=ORIENTED_EDGE('',*,*,#10328,.F.);
#15227=ORIENTED_EDGE('',*,*,#10329,.F.);
#15228=ORIENTED_EDGE('',*,*,#10204,.F.);
#15229=ORIENTED_EDGE('',*,*,#10205,.F.);
#15230=ORIENTED_EDGE('',*,*,#10329,.T.);
#15231=ORIENTED_EDGE('',*,*,#10330,.T.);
#15232=ORIENTED_EDGE('',*,*,#10331,.F.);
#15233=ORIENTED_EDGE('',*,*,#10206,.F.);
#15234=ORIENTED_EDGE('',*,*,#10330,.F.);
#15235=ORIENTED_EDGE('',*,*,#10328,.T.);
#15236=ORIENTED_EDGE('',*,*,#10332,.F.);
#15237=ORIENTED_EDGE('',*,*,#10333,.F.);
#15238=ORIENTED_EDGE('',*,*,#10334,.F.);
#15239=ORIENTED_EDGE('',*,*,#10208,.F.);
#15240=ORIENTED_EDGE('',*,*,#10209,.F.);
#15241=ORIENTED_EDGE('',*,*,#10334,.T.);
#15242=ORIENTED_EDGE('',*,*,#10335,.T.);
#15243=ORIENTED_EDGE('',*,*,#10336,.F.);
#15244=ORIENTED_EDGE('',*,*,#10210,.F.);
#15245=ORIENTED_EDGE('',*,*,#10335,.F.);
#15246=ORIENTED_EDGE('',*,*,#10333,.T.);
#15247=ORIENTED_EDGE('',*,*,#10337,.F.);
#15248=ORIENTED_EDGE('',*,*,#10338,.F.);
#15249=ORIENTED_EDGE('',*,*,#10339,.F.);
#15250=ORIENTED_EDGE('',*,*,#10212,.F.);
#15251=ORIENTED_EDGE('',*,*,#10213,.F.);
#15252=ORIENTED_EDGE('',*,*,#10339,.T.);
#15253=ORIENTED_EDGE('',*,*,#10340,.T.);
#15254=ORIENTED_EDGE('',*,*,#10341,.F.);
#15255=ORIENTED_EDGE('',*,*,#10214,.F.);
#15256=ORIENTED_EDGE('',*,*,#10340,.F.);
#15257=ORIENTED_EDGE('',*,*,#10338,.T.);
#15258=ORIENTED_EDGE('',*,*,#10342,.F.);
#15259=ORIENTED_EDGE('',*,*,#10343,.F.);
#15260=ORIENTED_EDGE('',*,*,#10344,.F.);
#15261=ORIENTED_EDGE('',*,*,#10216,.F.);
#15262=ORIENTED_EDGE('',*,*,#10217,.F.);
#15263=ORIENTED_EDGE('',*,*,#10344,.T.);
#15264=ORIENTED_EDGE('',*,*,#10345,.T.);
#15265=ORIENTED_EDGE('',*,*,#10346,.F.);
#15266=ORIENTED_EDGE('',*,*,#10218,.F.);
#15267=ORIENTED_EDGE('',*,*,#10345,.F.);
#15268=ORIENTED_EDGE('',*,*,#10343,.T.);
#15269=ORIENTED_EDGE('',*,*,#10347,.F.);
#15270=ORIENTED_EDGE('',*,*,#10348,.F.);
#15271=ORIENTED_EDGE('',*,*,#10349,.F.);
#15272=ORIENTED_EDGE('',*,*,#10220,.F.);
#15273=ORIENTED_EDGE('',*,*,#10221,.F.);
#15274=ORIENTED_EDGE('',*,*,#10349,.T.);
#15275=ORIENTED_EDGE('',*,*,#10350,.T.);
#15276=ORIENTED_EDGE('',*,*,#10351,.F.);
#15277=ORIENTED_EDGE('',*,*,#10222,.F.);
#15278=ORIENTED_EDGE('',*,*,#10350,.F.);
#15279=ORIENTED_EDGE('',*,*,#10348,.T.);
#15280=ORIENTED_EDGE('',*,*,#10352,.F.);
#15281=ORIENTED_EDGE('',*,*,#10353,.F.);
#15282=ORIENTED_EDGE('',*,*,#10354,.F.);
#15283=ORIENTED_EDGE('',*,*,#10224,.F.);
#15284=ORIENTED_EDGE('',*,*,#10225,.F.);
#15285=ORIENTED_EDGE('',*,*,#10354,.T.);
#15286=ORIENTED_EDGE('',*,*,#10355,.T.);
#15287=ORIENTED_EDGE('',*,*,#10356,.F.);
#15288=ORIENTED_EDGE('',*,*,#10226,.F.);
#15289=ORIENTED_EDGE('',*,*,#10355,.F.);
#15290=ORIENTED_EDGE('',*,*,#10353,.T.);
#15291=ORIENTED_EDGE('',*,*,#10357,.F.);
#15292=ORIENTED_EDGE('',*,*,#10358,.F.);
#15293=ORIENTED_EDGE('',*,*,#10359,.F.);
#15294=ORIENTED_EDGE('',*,*,#10228,.F.);
#15295=ORIENTED_EDGE('',*,*,#10229,.F.);
#15296=ORIENTED_EDGE('',*,*,#10359,.T.);
#15297=ORIENTED_EDGE('',*,*,#10360,.T.);
#15298=ORIENTED_EDGE('',*,*,#10361,.F.);
#15299=ORIENTED_EDGE('',*,*,#10230,.F.);
#15300=ORIENTED_EDGE('',*,*,#10360,.F.);
#15301=ORIENTED_EDGE('',*,*,#10358,.T.);
#15302=ORIENTED_EDGE('',*,*,#10362,.F.);
#15303=ORIENTED_EDGE('',*,*,#10363,.F.);
#15304=ORIENTED_EDGE('',*,*,#10364,.F.);
#15305=ORIENTED_EDGE('',*,*,#10232,.F.);
#15306=ORIENTED_EDGE('',*,*,#10233,.F.);
#15307=ORIENTED_EDGE('',*,*,#10364,.T.);
#15308=ORIENTED_EDGE('',*,*,#10365,.T.);
#15309=ORIENTED_EDGE('',*,*,#10366,.F.);
#15310=ORIENTED_EDGE('',*,*,#10234,.F.);
#15311=ORIENTED_EDGE('',*,*,#10365,.F.);
#15312=ORIENTED_EDGE('',*,*,#10363,.T.);
#15313=ORIENTED_EDGE('',*,*,#10367,.F.);
#15314=ORIENTED_EDGE('',*,*,#10368,.F.);
#15315=ORIENTED_EDGE('',*,*,#10369,.F.);
#15316=ORIENTED_EDGE('',*,*,#10236,.F.);
#15317=ORIENTED_EDGE('',*,*,#10237,.F.);
#15318=ORIENTED_EDGE('',*,*,#10369,.T.);
#15319=ORIENTED_EDGE('',*,*,#10370,.T.);
#15320=ORIENTED_EDGE('',*,*,#10371,.F.);
#15321=ORIENTED_EDGE('',*,*,#10238,.F.);
#15322=ORIENTED_EDGE('',*,*,#10370,.F.);
#15323=ORIENTED_EDGE('',*,*,#10368,.T.);
#15324=ORIENTED_EDGE('',*,*,#10372,.F.);
#15325=ORIENTED_EDGE('',*,*,#10373,.F.);
#15326=ORIENTED_EDGE('',*,*,#10374,.F.);
#15327=ORIENTED_EDGE('',*,*,#10240,.F.);
#15328=ORIENTED_EDGE('',*,*,#10241,.F.);
#15329=ORIENTED_EDGE('',*,*,#10374,.T.);
#15330=ORIENTED_EDGE('',*,*,#10375,.T.);
#15331=ORIENTED_EDGE('',*,*,#10244,.F.);
#15332=ORIENTED_EDGE('',*,*,#10376,.F.);
#15333=ORIENTED_EDGE('',*,*,#10245,.F.);
#15334=ORIENTED_EDGE('',*,*,#10375,.F.);
#15335=ORIENTED_EDGE('',*,*,#10373,.T.);
#15336=ORIENTED_EDGE('',*,*,#10377,.F.);
#15337=ORIENTED_EDGE('',*,*,#10378,.F.);
#15338=ORIENTED_EDGE('',*,*,#10379,.F.);
#15339=ORIENTED_EDGE('',*,*,#10247,.F.);
#15340=ORIENTED_EDGE('',*,*,#10248,.F.);
#15341=ORIENTED_EDGE('',*,*,#10379,.T.);
#15342=ORIENTED_EDGE('',*,*,#10380,.T.);
#15343=ORIENTED_EDGE('',*,*,#10381,.F.);
#15344=ORIENTED_EDGE('',*,*,#10249,.F.);
#15345=ORIENTED_EDGE('',*,*,#10380,.F.);
#15346=ORIENTED_EDGE('',*,*,#10378,.T.);
#15347=ORIENTED_EDGE('',*,*,#10382,.F.);
#15348=ORIENTED_EDGE('',*,*,#10383,.F.);
#15349=ORIENTED_EDGE('',*,*,#10384,.F.);
#15350=ORIENTED_EDGE('',*,*,#10251,.F.);
#15351=ORIENTED_EDGE('',*,*,#10252,.F.);
#15352=ORIENTED_EDGE('',*,*,#10384,.T.);
#15353=ORIENTED_EDGE('',*,*,#10385,.T.);
#15354=ORIENTED_EDGE('',*,*,#10386,.F.);
#15355=ORIENTED_EDGE('',*,*,#10253,.F.);
#15356=ORIENTED_EDGE('',*,*,#10385,.F.);
#15357=ORIENTED_EDGE('',*,*,#10383,.T.);
#15358=ORIENTED_EDGE('',*,*,#10387,.F.);
#15359=ORIENTED_EDGE('',*,*,#10388,.F.);
#15360=ORIENTED_EDGE('',*,*,#10389,.F.);
#15361=ORIENTED_EDGE('',*,*,#10255,.F.);
#15362=ORIENTED_EDGE('',*,*,#10256,.F.);
#15363=ORIENTED_EDGE('',*,*,#10389,.T.);
#15364=ORIENTED_EDGE('',*,*,#10390,.T.);
#15365=ORIENTED_EDGE('',*,*,#10391,.F.);
#15366=ORIENTED_EDGE('',*,*,#10257,.F.);
#15367=ORIENTED_EDGE('',*,*,#10390,.F.);
#15368=ORIENTED_EDGE('',*,*,#10388,.T.);
#15369=ORIENTED_EDGE('',*,*,#10392,.F.);
#15370=ORIENTED_EDGE('',*,*,#10393,.F.);
#15371=ORIENTED_EDGE('',*,*,#10394,.F.);
#15372=ORIENTED_EDGE('',*,*,#10259,.F.);
#15373=ORIENTED_EDGE('',*,*,#10260,.F.);
#15374=ORIENTED_EDGE('',*,*,#10394,.T.);
#15375=ORIENTED_EDGE('',*,*,#10395,.T.);
#15376=ORIENTED_EDGE('',*,*,#10396,.F.);
#15377=ORIENTED_EDGE('',*,*,#10261,.F.);
#15378=ORIENTED_EDGE('',*,*,#10395,.F.);
#15379=ORIENTED_EDGE('',*,*,#10393,.T.);
#15380=ORIENTED_EDGE('',*,*,#10397,.F.);
#15381=ORIENTED_EDGE('',*,*,#10398,.F.);
#15382=ORIENTED_EDGE('',*,*,#10399,.F.);
#15383=ORIENTED_EDGE('',*,*,#10263,.F.);
#15384=ORIENTED_EDGE('',*,*,#10264,.F.);
#15385=ORIENTED_EDGE('',*,*,#10399,.T.);
#15386=ORIENTED_EDGE('',*,*,#10400,.T.);
#15387=ORIENTED_EDGE('',*,*,#10401,.F.);
#15388=ORIENTED_EDGE('',*,*,#10265,.F.);
#15389=ORIENTED_EDGE('',*,*,#10400,.F.);
#15390=ORIENTED_EDGE('',*,*,#10398,.T.);
#15391=ORIENTED_EDGE('',*,*,#10402,.F.);
#15392=ORIENTED_EDGE('',*,*,#10403,.F.);
#15393=ORIENTED_EDGE('',*,*,#10404,.F.);
#15394=ORIENTED_EDGE('',*,*,#10267,.F.);
#15395=ORIENTED_EDGE('',*,*,#10268,.F.);
#15396=ORIENTED_EDGE('',*,*,#10404,.T.);
#15397=ORIENTED_EDGE('',*,*,#10405,.T.);
#15398=ORIENTED_EDGE('',*,*,#10406,.F.);
#15399=ORIENTED_EDGE('',*,*,#10269,.F.);
#15400=ORIENTED_EDGE('',*,*,#10405,.F.);
#15401=ORIENTED_EDGE('',*,*,#10403,.T.);
#15402=ORIENTED_EDGE('',*,*,#10407,.F.);
#15403=ORIENTED_EDGE('',*,*,#10408,.F.);
#15404=ORIENTED_EDGE('',*,*,#10409,.F.);
#15405=ORIENTED_EDGE('',*,*,#10271,.F.);
#15406=ORIENTED_EDGE('',*,*,#10272,.F.);
#15407=ORIENTED_EDGE('',*,*,#10409,.T.);
#15408=ORIENTED_EDGE('',*,*,#10410,.T.);
#15409=ORIENTED_EDGE('',*,*,#10411,.F.);
#15410=ORIENTED_EDGE('',*,*,#10273,.F.);
#15411=ORIENTED_EDGE('',*,*,#10410,.F.);
#15412=ORIENTED_EDGE('',*,*,#10408,.T.);
#15413=ORIENTED_EDGE('',*,*,#10412,.F.);
#15414=ORIENTED_EDGE('',*,*,#10413,.F.);
#15415=ORIENTED_EDGE('',*,*,#10414,.F.);
#15416=ORIENTED_EDGE('',*,*,#10275,.F.);
#15417=ORIENTED_EDGE('',*,*,#10276,.F.);
#15418=ORIENTED_EDGE('',*,*,#10414,.T.);
#15419=ORIENTED_EDGE('',*,*,#10415,.T.);
#15420=ORIENTED_EDGE('',*,*,#10416,.F.);
#15421=ORIENTED_EDGE('',*,*,#10277,.F.);
#15422=ORIENTED_EDGE('',*,*,#10415,.F.);
#15423=ORIENTED_EDGE('',*,*,#10413,.T.);
#15424=ORIENTED_EDGE('',*,*,#10417,.F.);
#15425=ORIENTED_EDGE('',*,*,#10418,.F.);
#15426=ORIENTED_EDGE('',*,*,#10419,.F.);
#15427=ORIENTED_EDGE('',*,*,#10279,.F.);
#15428=ORIENTED_EDGE('',*,*,#10280,.F.);
#15429=ORIENTED_EDGE('',*,*,#10419,.T.);
#15430=ORIENTED_EDGE('',*,*,#10420,.T.);
#15431=ORIENTED_EDGE('',*,*,#10421,.F.);
#15432=ORIENTED_EDGE('',*,*,#10281,.F.);
#15433=ORIENTED_EDGE('',*,*,#10420,.F.);
#15434=ORIENTED_EDGE('',*,*,#10418,.T.);
#15435=ORIENTED_EDGE('',*,*,#10422,.F.);
#15436=ORIENTED_EDGE('',*,*,#10423,.F.);
#15437=ORIENTED_EDGE('',*,*,#10424,.F.);
#15438=ORIENTED_EDGE('',*,*,#10283,.F.);
#15439=ORIENTED_EDGE('',*,*,#10284,.F.);
#15440=ORIENTED_EDGE('',*,*,#10424,.T.);
#15441=ORIENTED_EDGE('',*,*,#10425,.T.);
#15442=ORIENTED_EDGE('',*,*,#10426,.F.);
#15443=ORIENTED_EDGE('',*,*,#10285,.F.);
#15444=ORIENTED_EDGE('',*,*,#10425,.F.);
#15445=ORIENTED_EDGE('',*,*,#10423,.T.);
#15446=ORIENTED_EDGE('',*,*,#10427,.F.);
#15447=ORIENTED_EDGE('',*,*,#10428,.F.);
#15448=ORIENTED_EDGE('',*,*,#10429,.F.);
#15449=ORIENTED_EDGE('',*,*,#10287,.F.);
#15450=ORIENTED_EDGE('',*,*,#10288,.F.);
#15451=ORIENTED_EDGE('',*,*,#10429,.T.);
#15452=ORIENTED_EDGE('',*,*,#10430,.T.);
#15453=ORIENTED_EDGE('',*,*,#10431,.F.);
#15454=ORIENTED_EDGE('',*,*,#10289,.F.);
#15455=ORIENTED_EDGE('',*,*,#10430,.F.);
#15456=ORIENTED_EDGE('',*,*,#10428,.T.);
#15457=ORIENTED_EDGE('',*,*,#10432,.F.);
#15458=ORIENTED_EDGE('',*,*,#10433,.F.);
#15459=ORIENTED_EDGE('',*,*,#10434,.F.);
#15460=ORIENTED_EDGE('',*,*,#10291,.F.);
#15461=ORIENTED_EDGE('',*,*,#10292,.F.);
#15462=ORIENTED_EDGE('',*,*,#10434,.T.);
#15463=ORIENTED_EDGE('',*,*,#10435,.T.);
#15464=ORIENTED_EDGE('',*,*,#10436,.F.);
#15465=ORIENTED_EDGE('',*,*,#10293,.F.);
#15466=ORIENTED_EDGE('',*,*,#10435,.F.);
#15467=ORIENTED_EDGE('',*,*,#10433,.T.);
#15468=ORIENTED_EDGE('',*,*,#10437,.F.);
#15469=ORIENTED_EDGE('',*,*,#10438,.F.);
#15470=ORIENTED_EDGE('',*,*,#10439,.F.);
#15471=ORIENTED_EDGE('',*,*,#10295,.F.);
#15472=ORIENTED_EDGE('',*,*,#10296,.F.);
#15473=ORIENTED_EDGE('',*,*,#10439,.T.);
#15474=ORIENTED_EDGE('',*,*,#10440,.T.);
#15475=ORIENTED_EDGE('',*,*,#10441,.F.);
#15476=ORIENTED_EDGE('',*,*,#10297,.F.);
#15477=ORIENTED_EDGE('',*,*,#10440,.F.);
#15478=ORIENTED_EDGE('',*,*,#10438,.T.);
#15479=ORIENTED_EDGE('',*,*,#10442,.F.);
#15480=ORIENTED_EDGE('',*,*,#10443,.F.);
#15481=ORIENTED_EDGE('',*,*,#10444,.F.);
#15482=ORIENTED_EDGE('',*,*,#10299,.F.);
#15483=ORIENTED_EDGE('',*,*,#10300,.F.);
#15484=ORIENTED_EDGE('',*,*,#10444,.T.);
#15485=ORIENTED_EDGE('',*,*,#10445,.T.);
#15486=ORIENTED_EDGE('',*,*,#10446,.F.);
#15487=ORIENTED_EDGE('',*,*,#10301,.F.);
#15488=ORIENTED_EDGE('',*,*,#10445,.F.);
#15489=ORIENTED_EDGE('',*,*,#10443,.T.);
#15490=ORIENTED_EDGE('',*,*,#10447,.F.);
#15491=ORIENTED_EDGE('',*,*,#10448,.F.);
#15492=ORIENTED_EDGE('',*,*,#10449,.F.);
#15493=ORIENTED_EDGE('',*,*,#10303,.F.);
#15494=ORIENTED_EDGE('',*,*,#10304,.F.);
#15495=ORIENTED_EDGE('',*,*,#10449,.T.);
#15496=ORIENTED_EDGE('',*,*,#10450,.T.);
#15497=ORIENTED_EDGE('',*,*,#10451,.F.);
#15498=ORIENTED_EDGE('',*,*,#10305,.F.);
#15499=ORIENTED_EDGE('',*,*,#10450,.F.);
#15500=ORIENTED_EDGE('',*,*,#10448,.T.);
#15501=ORIENTED_EDGE('',*,*,#10452,.F.);
#15502=ORIENTED_EDGE('',*,*,#10172,.F.);
#15503=ORIENTED_EDGE('',*,*,#10081,.F.);
#15504=ORIENTED_EDGE('',*,*,#10173,.F.);
#15505=ORIENTED_EDGE('',*,*,#10453,.T.);
#15506=ORIENTED_EDGE('',*,*,#10452,.T.);
#15507=ORIENTED_EDGE('',*,*,#10453,.F.);
#15508=ORIENTED_EDGE('',*,*,#10122,.T.);
#15509=ORIENTED_EDGE('',*,*,#10169,.T.);
#15510=ORIENTED_EDGE('',*,*,#10454,.F.);
#15511=ORIENTED_EDGE('',*,*,#10178,.T.);
#15512=ORIENTED_EDGE('',*,*,#10455,.F.);
#15513=ORIENTED_EDGE('',*,*,#10454,.T.);
#15514=ORIENTED_EDGE('',*,*,#10168,.T.);
#15515=ORIENTED_EDGE('',*,*,#10127,.T.);
#15516=ORIENTED_EDGE('',*,*,#10177,.T.);
#15517=ORIENTED_EDGE('',*,*,#10243,.F.);
#15518=ORIENTED_EDGE('',*,*,#10456,.T.);
#15519=ORIENTED_EDGE('',*,*,#10455,.T.);
#15520=ORIENTED_EDGE('',*,*,#10456,.F.);
#15521=ORIENTED_EDGE('',*,*,#10457,.F.);
#15522=ORIENTED_EDGE('',*,*,#10458,.T.);
#15523=ORIENTED_EDGE('',*,*,#10372,.T.);
#15524=ORIENTED_EDGE('',*,*,#10239,.T.);
#15525=ORIENTED_EDGE('',*,*,#10371,.T.);
#15526=ORIENTED_EDGE('',*,*,#10367,.T.);
#15527=ORIENTED_EDGE('',*,*,#10235,.T.);
#15528=ORIENTED_EDGE('',*,*,#10366,.T.);
#15529=ORIENTED_EDGE('',*,*,#10362,.T.);
#15530=ORIENTED_EDGE('',*,*,#10231,.T.);
#15531=ORIENTED_EDGE('',*,*,#10361,.T.);
#15532=ORIENTED_EDGE('',*,*,#10357,.T.);
#15533=ORIENTED_EDGE('',*,*,#10227,.T.);
#15534=ORIENTED_EDGE('',*,*,#10356,.T.);
#15535=ORIENTED_EDGE('',*,*,#10352,.T.);
#15536=ORIENTED_EDGE('',*,*,#10223,.T.);
#15537=ORIENTED_EDGE('',*,*,#10351,.T.);
#15538=ORIENTED_EDGE('',*,*,#10347,.T.);
#15539=ORIENTED_EDGE('',*,*,#10219,.T.);
#15540=ORIENTED_EDGE('',*,*,#10346,.T.);
#15541=ORIENTED_EDGE('',*,*,#10342,.T.);
#15542=ORIENTED_EDGE('',*,*,#10215,.T.);
#15543=ORIENTED_EDGE('',*,*,#10341,.T.);
#15544=ORIENTED_EDGE('',*,*,#10337,.T.);
#15545=ORIENTED_EDGE('',*,*,#10211,.T.);
#15546=ORIENTED_EDGE('',*,*,#10336,.T.);
#15547=ORIENTED_EDGE('',*,*,#10332,.T.);
#15548=ORIENTED_EDGE('',*,*,#10207,.T.);
#15549=ORIENTED_EDGE('',*,*,#10331,.T.);
#15550=ORIENTED_EDGE('',*,*,#10327,.T.);
#15551=ORIENTED_EDGE('',*,*,#10203,.T.);
#15552=ORIENTED_EDGE('',*,*,#10326,.T.);
#15553=ORIENTED_EDGE('',*,*,#10322,.T.);
#15554=ORIENTED_EDGE('',*,*,#10199,.T.);
#15555=ORIENTED_EDGE('',*,*,#10321,.T.);
#15556=ORIENTED_EDGE('',*,*,#10317,.T.);
#15557=ORIENTED_EDGE('',*,*,#10195,.T.);
#15558=ORIENTED_EDGE('',*,*,#10316,.T.);
#15559=ORIENTED_EDGE('',*,*,#10312,.T.);
#15560=ORIENTED_EDGE('',*,*,#10191,.T.);
#15561=ORIENTED_EDGE('',*,*,#10311,.T.);
#15562=ORIENTED_EDGE('',*,*,#10307,.T.);
#15563=ORIENTED_EDGE('',*,*,#10187,.T.);
#15564=ORIENTED_EDGE('',*,*,#10185,.T.);
#15565=ORIENTED_EDGE('',*,*,#10179,.T.);
#15566=ORIENTED_EDGE('',*,*,#10306,.T.);
#15567=ORIENTED_EDGE('',*,*,#10451,.T.);
#15568=ORIENTED_EDGE('',*,*,#10447,.T.);
#15569=ORIENTED_EDGE('',*,*,#10302,.T.);
#15570=ORIENTED_EDGE('',*,*,#10446,.T.);
#15571=ORIENTED_EDGE('',*,*,#10442,.T.);
#15572=ORIENTED_EDGE('',*,*,#10298,.T.);
#15573=ORIENTED_EDGE('',*,*,#10441,.T.);
#15574=ORIENTED_EDGE('',*,*,#10437,.T.);
#15575=ORIENTED_EDGE('',*,*,#10294,.T.);
#15576=ORIENTED_EDGE('',*,*,#10436,.T.);
#15577=ORIENTED_EDGE('',*,*,#10432,.T.);
#15578=ORIENTED_EDGE('',*,*,#10290,.T.);
#15579=ORIENTED_EDGE('',*,*,#10431,.T.);
#15580=ORIENTED_EDGE('',*,*,#10427,.T.);
#15581=ORIENTED_EDGE('',*,*,#10286,.T.);
#15582=ORIENTED_EDGE('',*,*,#10426,.T.);
#15583=ORIENTED_EDGE('',*,*,#10422,.T.);
#15584=ORIENTED_EDGE('',*,*,#10282,.T.);
#15585=ORIENTED_EDGE('',*,*,#10421,.T.);
#15586=ORIENTED_EDGE('',*,*,#10417,.T.);
#15587=ORIENTED_EDGE('',*,*,#10278,.T.);
#15588=ORIENTED_EDGE('',*,*,#10416,.T.);
#15589=ORIENTED_EDGE('',*,*,#10412,.T.);
#15590=ORIENTED_EDGE('',*,*,#10274,.T.);
#15591=ORIENTED_EDGE('',*,*,#10411,.T.);
#15592=ORIENTED_EDGE('',*,*,#10407,.T.);
#15593=ORIENTED_EDGE('',*,*,#10270,.T.);
#15594=ORIENTED_EDGE('',*,*,#10406,.T.);
#15595=ORIENTED_EDGE('',*,*,#10402,.T.);
#15596=ORIENTED_EDGE('',*,*,#10266,.T.);
#15597=ORIENTED_EDGE('',*,*,#10401,.T.);
#15598=ORIENTED_EDGE('',*,*,#10397,.T.);
#15599=ORIENTED_EDGE('',*,*,#10262,.T.);
#15600=ORIENTED_EDGE('',*,*,#10396,.T.);
#15601=ORIENTED_EDGE('',*,*,#10392,.T.);
#15602=ORIENTED_EDGE('',*,*,#10258,.T.);
#15603=ORIENTED_EDGE('',*,*,#10391,.T.);
#15604=ORIENTED_EDGE('',*,*,#10387,.T.);
#15605=ORIENTED_EDGE('',*,*,#10254,.T.);
#15606=ORIENTED_EDGE('',*,*,#10386,.T.);
#15607=ORIENTED_EDGE('',*,*,#10382,.T.);
#15608=ORIENTED_EDGE('',*,*,#10250,.T.);
#15609=ORIENTED_EDGE('',*,*,#10381,.T.);
#15610=ORIENTED_EDGE('',*,*,#10377,.T.);
#15611=ORIENTED_EDGE('',*,*,#10246,.T.);
#15612=ORIENTED_EDGE('',*,*,#10376,.T.);
#15613=ORIENTED_EDGE('',*,*,#10458,.F.);
#15614=ORIENTED_EDGE('',*,*,#10457,.T.);
#15995=PLANE('',#18840);
#15996=PLANE('',#18845);
#15997=PLANE('',#18846);
#15998=PLANE('',#18848);
#15999=PLANE('',#18911);
#16000=PLANE('',#18912);
#16001=PLANE('',#18913);
#16002=PLANE('',#18914);
#16003=PLANE('',#18915);
#16004=PLANE('',#18916);
#16005=PLANE('',#18917);
#16006=PLANE('',#18918);
#16007=PLANE('',#18919);
#16008=PLANE('',#18920);
#16009=PLANE('',#18921);
#16010=PLANE('',#18922);
#16011=PLANE('',#18923);
#16012=PLANE('',#18924);
#16013=PLANE('',#18925);
#16014=PLANE('',#18926);
#16015=PLANE('',#18927);
#16016=PLANE('',#18928);
#16017=PLANE('',#18929);
#16018=PLANE('',#18930);
#16019=PLANE('',#18931);
#16020=PLANE('',#18932);
#16021=PLANE('',#18933);
#16022=PLANE('',#18934);
#16023=PLANE('',#18935);
#16024=PLANE('',#18936);
#16025=PLANE('',#18937);
#16026=PLANE('',#18938);
#16027=PLANE('',#18939);
#16028=PLANE('',#18940);
#16029=PLANE('',#18941);
#16030=PLANE('',#18942);
#16031=PLANE('',#18943);
#16032=PLANE('',#18944);
#16033=PLANE('',#18945);
#16034=PLANE('',#18946);
#16035=PLANE('',#18947);
#16036=PLANE('',#18948);
#16037=PLANE('',#18949);
#16038=PLANE('',#18950);
#16039=PLANE('',#18951);
#16040=PLANE('',#18952);
#16041=PLANE('',#18953);
#16042=PLANE('',#18954);
#16043=PLANE('',#18955);
#16044=PLANE('',#18956);
#16045=PLANE('',#18957);
#16046=PLANE('',#18958);
#16047=PLANE('',#18959);
#16048=PLANE('',#18960);
#16049=PLANE('',#18961);
#16050=PLANE('',#18962);
#16051=PLANE('',#18963);
#16052=PLANE('',#18964);
#16053=PLANE('',#18965);
#16054=PLANE('',#18966);
#16055=PLANE('',#18967);
#16056=PLANE('',#18968);
#16057=PLANE('',#18969);
#16058=PLANE('',#18970);
#16059=PLANE('',#18971);
#16060=PLANE('',#18972);
#16061=PLANE('',#18973);
#16062=PLANE('',#18974);
#16063=PLANE('',#18975);
#16064=PLANE('',#18976);
#16065=PLANE('',#18977);
#16066=PLANE('',#18978);
#16067=PLANE('',#18979);
#16068=PLANE('',#18980);
#16069=PLANE('',#18981);
#16070=PLANE('',#18982);
#16071=PLANE('',#18983);
#16072=PLANE('',#18984);
#16073=PLANE('',#18985);
#16074=PLANE('',#18986);
#16075=PLANE('',#18987);
#16076=PLANE('',#18988);
#16077=PLANE('',#18989);
#16078=PLANE('',#18990);
#16079=PLANE('',#18991);
#16080=PLANE('',#18992);
#16081=PLANE('',#18993);
#16082=PLANE('',#18994);
#16083=PLANE('',#18995);
#16084=PLANE('',#18996);
#16085=PLANE('',#18997);
#16086=PLANE('',#18998);
#16087=PLANE('',#19003);
#16088=PLANE('',#19008);
#16941=ADVANCED_FACE('',(#3132),#396,.T.);
#16942=ADVANCED_FACE('',(#3133),#397,.T.);
#16943=ADVANCED_FACE('',(#3134),#398,.T.);
#16944=ADVANCED_FACE('',(#3135),#399,.T.);
#16945=ADVANCED_FACE('',(#3136),#400,.T.);
#16946=ADVANCED_FACE('',(#3137),#401,.T.);
#16947=ADVANCED_FACE('',(#3138),#402,.T.);
#16948=ADVANCED_FACE('',(#3139),#403,.T.);
#16949=ADVANCED_FACE('',(#3140),#404,.T.);
#16950=ADVANCED_FACE('',(#3141),#405,.T.);
#16951=ADVANCED_FACE('',(#3142),#406,.T.);
#16952=ADVANCED_FACE('',(#3143),#407,.T.);
#16953=ADVANCED_FACE('',(#3144),#408,.T.);
#16954=ADVANCED_FACE('',(#3145),#409,.T.);
#16955=ADVANCED_FACE('',(#3146),#410,.T.);
#16956=ADVANCED_FACE('',(#3147),#411,.T.);
#16957=ADVANCED_FACE('',(#3148),#412,.T.);
#16958=ADVANCED_FACE('',(#3149),#413,.T.);
#16959=ADVANCED_FACE('',(#3150),#414,.T.);
#16960=ADVANCED_FACE('',(#3151),#415,.T.);
#16961=ADVANCED_FACE('',(#3152),#416,.T.);
#16962=ADVANCED_FACE('',(#3153),#417,.T.);
#16963=ADVANCED_FACE('',(#3154),#418,.T.);
#16964=ADVANCED_FACE('',(#3155),#419,.T.);
#16965=ADVANCED_FACE('',(#3156),#420,.T.);
#16966=ADVANCED_FACE('',(#3157),#421,.T.);
#16967=ADVANCED_FACE('',(#3158),#422,.T.);
#16968=ADVANCED_FACE('',(#3159),#423,.T.);
#16969=ADVANCED_FACE('',(#3160),#424,.T.);
#16970=ADVANCED_FACE('',(#3161),#89,.F.);
#16971=ADVANCED_FACE('',(#3162),#15995,.T.);
#16972=ADVANCED_FACE('',(#3163),#425,.T.);
#16973=ADVANCED_FACE('',(#3164),#90,.F.);
#16974=ADVANCED_FACE('',(#3165),#15996,.F.);
#16975=ADVANCED_FACE('',(#3166),#15997,.T.);
#16976=ADVANCED_FACE('',(#3167),#15998,.F.);
#16977=ADVANCED_FACE('',(#3168),#426,.T.);
#16978=ADVANCED_FACE('',(#3169),#15999,.F.);
#16979=ADVANCED_FACE('',(#3170),#16000,.T.);
#16980=ADVANCED_FACE('',(#3171),#16001,.F.);
#16981=ADVANCED_FACE('',(#3172),#16002,.F.);
#16982=ADVANCED_FACE('',(#3173),#16003,.T.);
#16983=ADVANCED_FACE('',(#3174),#16004,.F.);
#16984=ADVANCED_FACE('',(#3175),#16005,.F.);
#16985=ADVANCED_FACE('',(#3176),#16006,.T.);
#16986=ADVANCED_FACE('',(#3177),#16007,.F.);
#16987=ADVANCED_FACE('',(#3178),#16008,.F.);
#16988=ADVANCED_FACE('',(#3179),#16009,.T.);
#16989=ADVANCED_FACE('',(#3180),#16010,.F.);
#16990=ADVANCED_FACE('',(#3181),#16011,.F.);
#16991=ADVANCED_FACE('',(#3182),#16012,.T.);
#16992=ADVANCED_FACE('',(#3183),#16013,.F.);
#16993=ADVANCED_FACE('',(#3184),#16014,.F.);
#16994=ADVANCED_FACE('',(#3185),#16015,.T.);
#16995=ADVANCED_FACE('',(#3186),#16016,.F.);
#16996=ADVANCED_FACE('',(#3187),#16017,.F.);
#16997=ADVANCED_FACE('',(#3188),#16018,.T.);
#16998=ADVANCED_FACE('',(#3189),#16019,.F.);
#16999=ADVANCED_FACE('',(#3190),#16020,.F.);
#17000=ADVANCED_FACE('',(#3191),#16021,.T.);
#17001=ADVANCED_FACE('',(#3192),#16022,.F.);
#17002=ADVANCED_FACE('',(#3193),#16023,.F.);
#17003=ADVANCED_FACE('',(#3194),#16024,.T.);
#17004=ADVANCED_FACE('',(#3195),#16025,.F.);
#17005=ADVANCED_FACE('',(#3196),#16026,.F.);
#17006=ADVANCED_FACE('',(#3197),#16027,.T.);
#17007=ADVANCED_FACE('',(#3198),#16028,.F.);
#17008=ADVANCED_FACE('',(#3199),#16029,.F.);
#17009=ADVANCED_FACE('',(#3200),#16030,.T.);
#17010=ADVANCED_FACE('',(#3201),#16031,.F.);
#17011=ADVANCED_FACE('',(#3202),#16032,.F.);
#17012=ADVANCED_FACE('',(#3203),#16033,.T.);
#17013=ADVANCED_FACE('',(#3204),#16034,.F.);
#17014=ADVANCED_FACE('',(#3205),#16035,.F.);
#17015=ADVANCED_FACE('',(#3206),#16036,.T.);
#17016=ADVANCED_FACE('',(#3207),#16037,.F.);
#17017=ADVANCED_FACE('',(#3208),#16038,.F.);
#17018=ADVANCED_FACE('',(#3209),#16039,.T.);
#17019=ADVANCED_FACE('',(#3210),#16040,.F.);
#17020=ADVANCED_FACE('',(#3211),#16041,.F.);
#17021=ADVANCED_FACE('',(#3212),#16042,.T.);
#17022=ADVANCED_FACE('',(#3213),#16043,.F.);
#17023=ADVANCED_FACE('',(#3214),#16044,.F.);
#17024=ADVANCED_FACE('',(#3215),#16045,.T.);
#17025=ADVANCED_FACE('',(#3216),#16046,.F.);
#17026=ADVANCED_FACE('',(#3217),#16047,.F.);
#17027=ADVANCED_FACE('',(#3218),#16048,.T.);
#17028=ADVANCED_FACE('',(#3219),#16049,.F.);
#17029=ADVANCED_FACE('',(#3220),#16050,.F.);
#17030=ADVANCED_FACE('',(#3221),#16051,.T.);
#17031=ADVANCED_FACE('',(#3222),#16052,.F.);
#17032=ADVANCED_FACE('',(#3223),#16053,.F.);
#17033=ADVANCED_FACE('',(#3224),#16054,.T.);
#17034=ADVANCED_FACE('',(#3225),#16055,.F.);
#17035=ADVANCED_FACE('',(#3226),#16056,.F.);
#17036=ADVANCED_FACE('',(#3227),#16057,.T.);
#17037=ADVANCED_FACE('',(#3228),#16058,.F.);
#17038=ADVANCED_FACE('',(#3229),#16059,.F.);
#17039=ADVANCED_FACE('',(#3230),#16060,.T.);
#17040=ADVANCED_FACE('',(#3231),#16061,.F.);
#17041=ADVANCED_FACE('',(#3232),#16062,.F.);
#17042=ADVANCED_FACE('',(#3233),#16063,.T.);
#17043=ADVANCED_FACE('',(#3234),#16064,.F.);
#17044=ADVANCED_FACE('',(#3235),#16065,.F.);
#17045=ADVANCED_FACE('',(#3236),#16066,.T.);
#17046=ADVANCED_FACE('',(#3237),#16067,.F.);
#17047=ADVANCED_FACE('',(#3238),#16068,.F.);
#17048=ADVANCED_FACE('',(#3239),#16069,.T.);
#17049=ADVANCED_FACE('',(#3240),#16070,.F.);
#17050=ADVANCED_FACE('',(#3241),#16071,.F.);
#17051=ADVANCED_FACE('',(#3242),#16072,.T.);
#17052=ADVANCED_FACE('',(#3243),#16073,.F.);
#17053=ADVANCED_FACE('',(#3244),#16074,.F.);
#17054=ADVANCED_FACE('',(#3245),#16075,.T.);
#17055=ADVANCED_FACE('',(#3246),#16076,.F.);
#17056=ADVANCED_FACE('',(#3247),#16077,.F.);
#17057=ADVANCED_FACE('',(#3248),#16078,.T.);
#17058=ADVANCED_FACE('',(#3249),#16079,.F.);
#17059=ADVANCED_FACE('',(#3250),#16080,.F.);
#17060=ADVANCED_FACE('',(#3251),#16081,.T.);
#17061=ADVANCED_FACE('',(#3252),#16082,.F.);
#17062=ADVANCED_FACE('',(#3253),#16083,.F.);
#17063=ADVANCED_FACE('',(#3254),#16084,.T.);
#17064=ADVANCED_FACE('',(#3255),#16085,.F.);
#17065=ADVANCED_FACE('',(#3256),#16086,.T.);
#17066=ADVANCED_FACE('',(#3257),#1048,.T.);
#17067=ADVANCED_FACE('',(#3258),#427,.T.);
#17068=ADVANCED_FACE('',(#3259,#1476),#16087,.T.);
#17069=ADVANCED_FACE('',(#3260),#1049,.T.);
#17070=ADVANCED_FACE('',(#3261),#1050,.T.);
#17071=ADVANCED_FACE('',(#3262),#16088,.T.);
#17083=CLOSED_SHELL('',(#16941,#16942,#16943,#16944,#16945,#16946,#16947,
#16948,#16949,#16950,#16951,#16952,#16953,#16954,#16955,#16956,#16957,#16958,
#16959,#16960,#16961,#16962,#16963,#16964,#16965,#16966,#16967,#16968,#16969,
#16970,#16971,#16972,#16973,#16974,#16975,#16976,#16977,#16978,#16979,#16980,
#16981,#16982,#16983,#16984,#16985,#16986,#16987,#16988,#16989,#16990,#16991,
#16992,#16993,#16994,#16995,#16996,#16997,#16998,#16999,#17000,#17001,#17002,
#17003,#17004,#17005,#17006,#17007,#17008,#17009,#17010,#17011,#17012,#17013,
#17014,#17015,#17016,#17017,#17018,#17019,#17020,#17021,#17022,#17023,#17024,
#17025,#17026,#17027,#17028,#17029,#17030,#17031,#17032,#17033,#17034,#17035,
#17036,#17037,#17038,#17039,#17040,#17041,#17042,#17043,#17044,#17045,#17046,
#17047,#17048,#17049,#17050,#17051,#17052,#17053,#17054,#17055,#17056,#17057,
#17058,#17059,#17060,#17061,#17062,#17063,#17064,#17065,#17066,#17067,#17068,
#17069,#17070,#17071));
#18808=AXIS2_PLACEMENT_3D('',#35571,#22999,#23000);
#18809=AXIS2_PLACEMENT_3D('',#35572,#23001,#23002);
#18810=AXIS2_PLACEMENT_3D('',#35588,#23004,#23005);
#18811=AXIS2_PLACEMENT_3D('',#35596,#23006,#23007);
#18812=AXIS2_PLACEMENT_3D('',#35644,#23009,#23010);
#18813=AXIS2_PLACEMENT_3D('',#35692,#23012,#23013);
#18814=AXIS2_PLACEMENT_3D('',#35746,#23015,#23016);
#18815=AXIS2_PLACEMENT_3D('',#35794,#23018,#23019);
#18816=AXIS2_PLACEMENT_3D('',#35842,#23021,#23022);
#18817=AXIS2_PLACEMENT_3D('',#35890,#23024,#23025);
#18818=AXIS2_PLACEMENT_3D('',#35944,#23027,#23028);
#18819=AXIS2_PLACEMENT_3D('',#35992,#23030,#23031);
#18820=AXIS2_PLACEMENT_3D('',#36040,#23033,#23034);
#18821=AXIS2_PLACEMENT_3D('',#36094,#23036,#23037);
#18822=AXIS2_PLACEMENT_3D('',#36142,#23039,#23040);
#18823=AXIS2_PLACEMENT_3D('',#36190,#23042,#23043);
#18824=AXIS2_PLACEMENT_3D('',#36244,#23045,#23046);
#18825=AXIS2_PLACEMENT_3D('',#36292,#23048,#23049);
#18826=AXIS2_PLACEMENT_3D('',#36307,#23051,#23052);
#18827=AXIS2_PLACEMENT_3D('',#36316,#23053,#23054);
#18828=AXIS2_PLACEMENT_3D('',#36341,#23056,#23057);
#18829=AXIS2_PLACEMENT_3D('',#36366,#23059,#23060);
#18830=AXIS2_PLACEMENT_3D('',#36390,#23062,#23063);
#18831=AXIS2_PLACEMENT_3D('',#36415,#23065,#23066);
#18832=AXIS2_PLACEMENT_3D('',#36440,#23068,#23069);
#18833=AXIS2_PLACEMENT_3D('',#36464,#23071,#23072);
#18834=AXIS2_PLACEMENT_3D('',#36489,#23074,#23075);
#18835=AXIS2_PLACEMENT_3D('',#36514,#23077,#23078);
#18836=AXIS2_PLACEMENT_3D('',#36538,#23080,#23081);
#18837=AXIS2_PLACEMENT_3D('',#36562,#23083,#23084);
#18838=AXIS2_PLACEMENT_3D('',#36587,#23086,#23087);
#18839=AXIS2_PLACEMENT_3D('',#36612,#23089,#23090);
#18840=AXIS2_PLACEMENT_3D('',#37218,#23092,#23093);
#18841=AXIS2_PLACEMENT_3D('',#37220,#23094,#23095);
#18842=AXIS2_PLACEMENT_3D('',#37221,#23096,#23097);
#18843=AXIS2_PLACEMENT_3D('',#37311,#23098,#23099);
#18844=AXIS2_PLACEMENT_3D('',#37312,#23100,#23101);
#18845=AXIS2_PLACEMENT_3D('',#37802,#23102,#23103);
#18846=AXIS2_PLACEMENT_3D('',#37813,#23107,#23108);
#18847=AXIS2_PLACEMENT_3D('',#37815,#23109,#23110);
#18848=AXIS2_PLACEMENT_3D('',#37817,#23112,#23113);
#18849=AXIS2_PLACEMENT_3D('',#37823,#23115,#23116);
#18850=AXIS2_PLACEMENT_3D('',#37825,#23117,#23118);
#18851=AXIS2_PLACEMENT_3D('',#37829,#23120,#23121);
#18852=AXIS2_PLACEMENT_3D('',#37833,#23123,#23124);
#18853=AXIS2_PLACEMENT_3D('',#37837,#23126,#23127);
#18854=AXIS2_PLACEMENT_3D('',#37841,#23129,#23130);
#18855=AXIS2_PLACEMENT_3D('',#37845,#23132,#23133);
#18856=AXIS2_PLACEMENT_3D('',#37849,#23135,#23136);
#18857=AXIS2_PLACEMENT_3D('',#37853,#23138,#23139);
#18858=AXIS2_PLACEMENT_3D('',#37857,#23141,#23142);
#18859=AXIS2_PLACEMENT_3D('',#37861,#23144,#23145);
#18860=AXIS2_PLACEMENT_3D('',#37865,#23147,#23148);
#18861=AXIS2_PLACEMENT_3D('',#37869,#23150,#23151);
#18862=AXIS2_PLACEMENT_3D('',#37873,#23153,#23154);
#18863=AXIS2_PLACEMENT_3D('',#37877,#23156,#23157);
#18864=AXIS2_PLACEMENT_3D('',#37881,#23159,#23160);
#18865=AXIS2_PLACEMENT_3D('',#37885,#23162,#23163);
#18866=AXIS2_PLACEMENT_3D('',#37889,#23165,#23166);
#18867=AXIS2_PLACEMENT_3D('',#37893,#23168,#23169);
#18868=AXIS2_PLACEMENT_3D('',#37897,#23171,#23172);
#18869=AXIS2_PLACEMENT_3D('',#37901,#23174,#23175);
#18870=AXIS2_PLACEMENT_3D('',#37905,#23177,#23178);
#18871=AXIS2_PLACEMENT_3D('',#37909,#23180,#23181);
#18872=AXIS2_PLACEMENT_3D('',#37913,#23183,#23184);
#18873=AXIS2_PLACEMENT_3D('',#37917,#23186,#23187);
#18874=AXIS2_PLACEMENT_3D('',#37921,#23189,#23190);
#18875=AXIS2_PLACEMENT_3D('',#37925,#23192,#23193);
#18876=AXIS2_PLACEMENT_3D('',#37929,#23195,#23196);
#18877=AXIS2_PLACEMENT_3D('',#37933,#23198,#23199);
#18878=AXIS2_PLACEMENT_3D('',#37936,#23201,#23202);
#18879=AXIS2_PLACEMENT_3D('',#37938,#23203,#23204);
#18880=AXIS2_PLACEMENT_3D('',#37942,#23206,#23207);
#18881=AXIS2_PLACEMENT_3D('',#37946,#23209,#23210);
#18882=AXIS2_PLACEMENT_3D('',#37950,#23212,#23213);
#18883=AXIS2_PLACEMENT_3D('',#37954,#23215,#23216);
#18884=AXIS2_PLACEMENT_3D('',#37958,#23218,#23219);
#18885=AXIS2_PLACEMENT_3D('',#37962,#23221,#23222);
#18886=AXIS2_PLACEMENT_3D('',#37966,#23224,#23225);
#18887=AXIS2_PLACEMENT_3D('',#37970,#23227,#23228);
#18888=AXIS2_PLACEMENT_3D('',#37974,#23230,#23231);
#18889=AXIS2_PLACEMENT_3D('',#37978,#23233,#23234);
#18890=AXIS2_PLACEMENT_3D('',#37982,#23236,#23237);
#18891=AXIS2_PLACEMENT_3D('',#37986,#23239,#23240);
#18892=AXIS2_PLACEMENT_3D('',#37990,#23242,#23243);
#18893=AXIS2_PLACEMENT_3D('',#37994,#23245,#23246);
#18894=AXIS2_PLACEMENT_3D('',#37998,#23248,#23249);
#18895=AXIS2_PLACEMENT_3D('',#38002,#23251,#23252);
#18896=AXIS2_PLACEMENT_3D('',#38006,#23254,#23255);
#18897=AXIS2_PLACEMENT_3D('',#38010,#23257,#23258);
#18898=AXIS2_PLACEMENT_3D('',#38014,#23260,#23261);
#18899=AXIS2_PLACEMENT_3D('',#38018,#23263,#23264);
#18900=AXIS2_PLACEMENT_3D('',#38022,#23266,#23267);
#18901=AXIS2_PLACEMENT_3D('',#38026,#23269,#23270);
#18902=AXIS2_PLACEMENT_3D('',#38030,#23272,#23273);
#18903=AXIS2_PLACEMENT_3D('',#38034,#23275,#23276);
#18904=AXIS2_PLACEMENT_3D('',#38038,#23278,#23279);
#18905=AXIS2_PLACEMENT_3D('',#38042,#23281,#23282);
#18906=AXIS2_PLACEMENT_3D('',#38046,#23284,#23285);
#18907=AXIS2_PLACEMENT_3D('',#38050,#23287,#23288);
#18908=AXIS2_PLACEMENT_3D('',#38054,#23290,#23291);
#18909=AXIS2_PLACEMENT_3D('',#38058,#23293,#23294);
#18910=AXIS2_PLACEMENT_3D('',#38061,#23296,#23297);
#18911=AXIS2_PLACEMENT_3D('',#38062,#23298,#23299);
#18912=AXIS2_PLACEMENT_3D('',#38070,#23302,#23303);
#18913=AXIS2_PLACEMENT_3D('',#38072,#23305,#23306);
#18914=AXIS2_PLACEMENT_3D('',#38076,#23307,#23308);
#18915=AXIS2_PLACEMENT_3D('',#38084,#23311,#23312);
#18916=AXIS2_PLACEMENT_3D('',#38086,#23314,#23315);
#18917=AXIS2_PLACEMENT_3D('',#38090,#23316,#23317);
#18918=AXIS2_PLACEMENT_3D('',#38098,#23320,#23321);
#18919=AXIS2_PLACEMENT_3D('',#38100,#23323,#23324);
#18920=AXIS2_PLACEMENT_3D('',#38104,#23325,#23326);
#18921=AXIS2_PLACEMENT_3D('',#38112,#23329,#23330);
#18922=AXIS2_PLACEMENT_3D('',#38114,#23332,#23333);
#18923=AXIS2_PLACEMENT_3D('',#38118,#23334,#23335);
#18924=AXIS2_PLACEMENT_3D('',#38126,#23338,#23339);
#18925=AXIS2_PLACEMENT_3D('',#38128,#23341,#23342);
#18926=AXIS2_PLACEMENT_3D('',#38132,#23343,#23344);
#18927=AXIS2_PLACEMENT_3D('',#38140,#23347,#23348);
#18928=AXIS2_PLACEMENT_3D('',#38142,#23350,#23351);
#18929=AXIS2_PLACEMENT_3D('',#38146,#23352,#23353);
#18930=AXIS2_PLACEMENT_3D('',#38154,#23356,#23357);
#18931=AXIS2_PLACEMENT_3D('',#38156,#23359,#23360);
#18932=AXIS2_PLACEMENT_3D('',#38160,#23361,#23362);
#18933=AXIS2_PLACEMENT_3D('',#38168,#23365,#23366);
#18934=AXIS2_PLACEMENT_3D('',#38170,#23368,#23369);
#18935=AXIS2_PLACEMENT_3D('',#38174,#23370,#23371);
#18936=AXIS2_PLACEMENT_3D('',#38182,#23374,#23375);
#18937=AXIS2_PLACEMENT_3D('',#38184,#23377,#23378);
#18938=AXIS2_PLACEMENT_3D('',#38188,#23379,#23380);
#18939=AXIS2_PLACEMENT_3D('',#38196,#23383,#23384);
#18940=AXIS2_PLACEMENT_3D('',#38198,#23386,#23387);
#18941=AXIS2_PLACEMENT_3D('',#38202,#23388,#23389);
#18942=AXIS2_PLACEMENT_3D('',#38210,#23392,#23393);
#18943=AXIS2_PLACEMENT_3D('',#38212,#23395,#23396);
#18944=AXIS2_PLACEMENT_3D('',#38216,#23397,#23398);
#18945=AXIS2_PLACEMENT_3D('',#38224,#23401,#23402);
#18946=AXIS2_PLACEMENT_3D('',#38226,#23404,#23405);
#18947=AXIS2_PLACEMENT_3D('',#38230,#23406,#23407);
#18948=AXIS2_PLACEMENT_3D('',#38238,#23410,#23411);
#18949=AXIS2_PLACEMENT_3D('',#38240,#23413,#23414);
#18950=AXIS2_PLACEMENT_3D('',#38244,#23415,#23416);
#18951=AXIS2_PLACEMENT_3D('',#38252,#23419,#23420);
#18952=AXIS2_PLACEMENT_3D('',#38254,#23422,#23423);
#18953=AXIS2_PLACEMENT_3D('',#38258,#23424,#23425);
#18954=AXIS2_PLACEMENT_3D('',#38266,#23428,#23429);
#18955=AXIS2_PLACEMENT_3D('',#38268,#23431,#23432);
#18956=AXIS2_PLACEMENT_3D('',#38272,#23433,#23434);
#18957=AXIS2_PLACEMENT_3D('',#38280,#23437,#23438);
#18958=AXIS2_PLACEMENT_3D('',#38282,#23440,#23441);
#18959=AXIS2_PLACEMENT_3D('',#38286,#23442,#23443);
#18960=AXIS2_PLACEMENT_3D('',#38294,#23446,#23447);
#18961=AXIS2_PLACEMENT_3D('',#38296,#23449,#23450);
#18962=AXIS2_PLACEMENT_3D('',#38300,#23451,#23452);
#18963=AXIS2_PLACEMENT_3D('',#38308,#23455,#23456);
#18964=AXIS2_PLACEMENT_3D('',#38310,#23458,#23459);
#18965=AXIS2_PLACEMENT_3D('',#38314,#23460,#23461);
#18966=AXIS2_PLACEMENT_3D('',#38322,#23464,#23465);
#18967=AXIS2_PLACEMENT_3D('',#38324,#23467,#23468);
#18968=AXIS2_PLACEMENT_3D('',#38328,#23469,#23470);
#18969=AXIS2_PLACEMENT_3D('',#38336,#23473,#23474);
#18970=AXIS2_PLACEMENT_3D('',#38338,#23476,#23477);
#18971=AXIS2_PLACEMENT_3D('',#38342,#23478,#23479);
#18972=AXIS2_PLACEMENT_3D('',#38350,#23482,#23483);
#18973=AXIS2_PLACEMENT_3D('',#38352,#23485,#23486);
#18974=AXIS2_PLACEMENT_3D('',#38356,#23487,#23488);
#18975=AXIS2_PLACEMENT_3D('',#38364,#23491,#23492);
#18976=AXIS2_PLACEMENT_3D('',#38366,#23494,#23495);
#18977=AXIS2_PLACEMENT_3D('',#38370,#23496,#23497);
#18978=AXIS2_PLACEMENT_3D('',#38378,#23500,#23501);
#18979=AXIS2_PLACEMENT_3D('',#38380,#23503,#23504);
#18980=AXIS2_PLACEMENT_3D('',#38384,#23505,#23506);
#18981=AXIS2_PLACEMENT_3D('',#38392,#23509,#23510);
#18982=AXIS2_PLACEMENT_3D('',#38394,#23512,#23513);
#18983=AXIS2_PLACEMENT_3D('',#38398,#23514,#23515);
#18984=AXIS2_PLACEMENT_3D('',#38406,#23518,#23519);
#18985=AXIS2_PLACEMENT_3D('',#38408,#23521,#23522);
#18986=AXIS2_PLACEMENT_3D('',#38412,#23523,#23524);
#18987=AXIS2_PLACEMENT_3D('',#38420,#23527,#23528);
#18988=AXIS2_PLACEMENT_3D('',#38422,#23530,#23531);
#18989=AXIS2_PLACEMENT_3D('',#38426,#23532,#23533);
#18990=AXIS2_PLACEMENT_3D('',#38434,#23536,#23537);
#18991=AXIS2_PLACEMENT_3D('',#38436,#23539,#23540);
#18992=AXIS2_PLACEMENT_3D('',#38440,#23541,#23542);
#18993=AXIS2_PLACEMENT_3D('',#38448,#23545,#23546);
#18994=AXIS2_PLACEMENT_3D('',#38450,#23548,#23549);
#18995=AXIS2_PLACEMENT_3D('',#38454,#23550,#23551);
#18996=AXIS2_PLACEMENT_3D('',#38462,#23554,#23555);
#18997=AXIS2_PLACEMENT_3D('',#38464,#23557,#23558);
#18998=AXIS2_PLACEMENT_3D('',#38468,#23559,#23560);
#18999=AXIS2_PLACEMENT_3D('',#38470,#23561,#23562);
#19000=AXIS2_PLACEMENT_3D('',#38471,#23563,#23564);
#19001=AXIS2_PLACEMENT_3D('',#38473,#23566,#23567);
#19002=AXIS2_PLACEMENT_3D('',#38474,#23568,#23569);
#19003=AXIS2_PLACEMENT_3D('',#38475,#23570,#23571);
#19004=AXIS2_PLACEMENT_3D('',#38477,#23572,#23573);
#19005=AXIS2_PLACEMENT_3D('',#38478,#23574,#23575);
#19006=AXIS2_PLACEMENT_3D('',#38480,#23577,#23578);
#19007=AXIS2_PLACEMENT_3D('',#38482,#23579,#23580);
#19008=AXIS2_PLACEMENT_3D('',#38484,#23582,#23583);
#22999=DIRECTION('axis',(0.,0.,1.));
#23000=DIRECTION('refdir',(1.,0.,0.));
#23001=DIRECTION('center_axis',(1.,0.,0.));
#23002=DIRECTION('ref_axis',(0.,1.,0.));
#23003=DIRECTION('',(-1.,0.,0.));
#23004=DIRECTION('center_axis',(1.,0.,0.));
#23005=DIRECTION('ref_axis',(0.,1.,0.));
#23006=DIRECTION('center_axis',(1.,0.,0.));
#23007=DIRECTION('ref_axis',(0.,1.,0.));
#23008=DIRECTION('',(-1.,0.,0.));
#23009=DIRECTION('center_axis',(1.,0.,0.));
#23010=DIRECTION('ref_axis',(0.,1.,0.));
#23011=DIRECTION('',(-1.,0.,0.));
#23012=DIRECTION('center_axis',(1.,0.,0.));
#23013=DIRECTION('ref_axis',(0.,1.,0.));
#23014=DIRECTION('',(-1.,0.,0.));
#23015=DIRECTION('center_axis',(1.,0.,0.));
#23016=DIRECTION('ref_axis',(0.,1.,0.));
#23017=DIRECTION('',(-1.,0.,0.));
#23018=DIRECTION('center_axis',(1.,0.,0.));
#23019=DIRECTION('ref_axis',(0.,1.,0.));
#23020=DIRECTION('',(-1.,0.,0.));
#23021=DIRECTION('center_axis',(1.,0.,0.));
#23022=DIRECTION('ref_axis',(0.,1.,0.));
#23023=DIRECTION('',(-1.,0.,0.));
#23024=DIRECTION('center_axis',(1.,0.,0.));
#23025=DIRECTION('ref_axis',(0.,1.,0.));
#23026=DIRECTION('',(-1.,0.,0.));
#23027=DIRECTION('center_axis',(1.,0.,0.));
#23028=DIRECTION('ref_axis',(0.,1.,0.));
#23029=DIRECTION('',(-1.,0.,0.));
#23030=DIRECTION('center_axis',(1.,0.,0.));
#23031=DIRECTION('ref_axis',(0.,1.,0.));
#23032=DIRECTION('',(-1.,0.,0.));
#23033=DIRECTION('center_axis',(1.,0.,0.));
#23034=DIRECTION('ref_axis',(0.,1.,0.));
#23035=DIRECTION('',(-1.,0.,0.));
#23036=DIRECTION('center_axis',(1.,0.,0.));
#23037=DIRECTION('ref_axis',(0.,1.,0.));
#23038=DIRECTION('',(-1.,0.,0.));
#23039=DIRECTION('center_axis',(1.,0.,0.));
#23040=DIRECTION('ref_axis',(0.,1.,0.));
#23041=DIRECTION('',(-1.,0.,0.));
#23042=DIRECTION('center_axis',(1.,0.,0.));
#23043=DIRECTION('ref_axis',(0.,1.,0.));
#23044=DIRECTION('',(-1.,0.,0.));
#23045=DIRECTION('center_axis',(1.,0.,0.));
#23046=DIRECTION('ref_axis',(0.,1.,0.));
#23047=DIRECTION('',(-1.,0.,0.));
#23048=DIRECTION('center_axis',(1.,0.,0.));
#23049=DIRECTION('ref_axis',(0.,0.960826707559551,-0.27714984762809));
#23050=DIRECTION('',(1.,0.,0.));
#23051=DIRECTION('center_axis',(1.,0.,0.));
#23052=DIRECTION('ref_axis',(0.,1.,9.63181083013289E-14));
#23053=DIRECTION('center_axis',(1.,0.,0.));
#23054=DIRECTION('ref_axis',(0.,1.,9.63181083013289E-14));
#23055=DIRECTION('',(1.,0.,0.));
#23056=DIRECTION('center_axis',(1.,0.,0.));
#23057=DIRECTION('ref_axis',(0.,1.,9.63181083013289E-14));
#23058=DIRECTION('',(1.,0.,0.));
#23059=DIRECTION('center_axis',(1.,0.,0.));
#23060=DIRECTION('ref_axis',(0.,1.,9.63181083013289E-14));
#23061=DIRECTION('',(1.,0.,0.));
#23062=DIRECTION('center_axis',(1.,0.,0.));
#23063=DIRECTION('ref_axis',(0.,1.,9.63181083013289E-14));
#23064=DIRECTION('',(1.,0.,0.));
#23065=DIRECTION('center_axis',(1.,0.,0.));
#23066=DIRECTION('ref_axis',(0.,1.,9.63181083013289E-14));
#23067=DIRECTION('',(1.,0.,0.));
#23068=DIRECTION('center_axis',(1.,0.,0.));
#23069=DIRECTION('ref_axis',(0.,1.,9.63181083013289E-14));
#23070=DIRECTION('',(1.,0.,0.));
#23071=DIRECTION('center_axis',(1.,0.,0.));
#23072=DIRECTION('ref_axis',(0.,1.,9.63181083013289E-14));
#23073=DIRECTION('',(1.,0.,0.));
#23074=DIRECTION('center_axis',(1.,0.,0.));
#23075=DIRECTION('ref_axis',(0.,1.,9.63181083013289E-14));
#23076=DIRECTION('',(1.,0.,0.));
#23077=DIRECTION('center_axis',(1.,0.,0.));
#23078=DIRECTION('ref_axis',(0.,1.,9.63181083013289E-14));
#23079=DIRECTION('',(1.,0.,0.));
#23080=DIRECTION('center_axis',(1.,0.,0.));
#23081=DIRECTION('ref_axis',(0.,1.,9.63181083013289E-14));
#23082=DIRECTION('',(1.,0.,0.));
#23083=DIRECTION('center_axis',(1.,0.,0.));
#23084=DIRECTION('ref_axis',(0.,1.,9.63181083013289E-14));
#23085=DIRECTION('',(1.,0.,0.));
#23086=DIRECTION('center_axis',(1.,0.,0.));
#23087=DIRECTION('ref_axis',(0.,1.,9.63181083013289E-14));
#23088=DIRECTION('',(1.,0.,0.));
#23089=DIRECTION('center_axis',(1.,0.,0.));
#23090=DIRECTION('ref_axis',(0.,1.,9.63181083013289E-14));
#23091=DIRECTION('',(1.,0.,0.));
#23092=DIRECTION('center_axis',(1.,0.,0.));
#23093=DIRECTION('ref_axis',(0.,0.,-1.));
#23094=DIRECTION('center_axis',(1.,0.,0.));
#23095=DIRECTION('ref_axis',(0.,1.,0.));
#23096=DIRECTION('center_axis',(1.,0.,0.));
#23097=DIRECTION('ref_axis',(0.,1.,0.));
#23098=DIRECTION('center_axis',(-1.,0.,0.));
#23099=DIRECTION('ref_axis',(0.,1.,9.63181083013289E-14));
#23100=DIRECTION('center_axis',(1.,0.,0.));
#23101=DIRECTION('ref_axis',(0.,1.,9.63181083013289E-14));
#23102=DIRECTION('center_axis',(0.,-0.499806704490841,0.866136974240221));
#23103=DIRECTION('ref_axis',(0.,-0.866136974240221,-0.499806704490841));
#23104=DIRECTION('',(1.,0.,0.));
#23105=DIRECTION('',(0.,-0.866136974240221,-0.499806704490841));
#23106=DIRECTION('',(-1.,0.,0.));
#23107=DIRECTION('center_axis',(1.,0.,0.));
#23108=DIRECTION('ref_axis',(0.,-0.20791169081776,-0.978147600733805));
#23109=DIRECTION('center_axis',(-1.,0.,0.));
#23110=DIRECTION('ref_axis',(0.,1.,0.));
#23111=DIRECTION('',(0.,0.587965797342076,-0.808885789933225));
#23112=DIRECTION('center_axis',(0.,-0.808885789933225,-0.587965797342076));
#23113=DIRECTION('ref_axis',(0.,0.587965797342076,-0.808885789933225));
#23114=DIRECTION('',(1.,0.,0.));
#23115=DIRECTION('center_axis',(1.,0.,0.));
#23116=DIRECTION('ref_axis',(0.,1.,0.));
#23117=DIRECTION('center_axis',(1.,0.,0.));
#23118=DIRECTION('ref_axis',(0.,0.,-1.));
#23119=DIRECTION('',(-1.,0.,0.));
#23120=DIRECTION('center_axis',(-1.,0.,0.));
#23121=DIRECTION('ref_axis',(0.,1.,0.));
#23122=DIRECTION('',(1.,0.,0.));
#23123=DIRECTION('center_axis',(1.,0.,0.));
#23124=DIRECTION('ref_axis',(0.,0.,-1.));
#23125=DIRECTION('',(-1.,0.,0.));
#23126=DIRECTION('center_axis',(-1.,0.,0.));
#23127=DIRECTION('ref_axis',(0.,1.,0.));
#23128=DIRECTION('',(1.,0.,0.));
#23129=DIRECTION('center_axis',(1.,0.,0.));
#23130=DIRECTION('ref_axis',(0.,0.,-1.));
#23131=DIRECTION('',(-1.,0.,0.));
#23132=DIRECTION('center_axis',(-1.,0.,0.));
#23133=DIRECTION('ref_axis',(0.,1.,0.));
#23134=DIRECTION('',(1.,0.,0.));
#23135=DIRECTION('center_axis',(1.,0.,0.));
#23136=DIRECTION('ref_axis',(0.,0.,-1.));
#23137=DIRECTION('',(-1.,0.,0.));
#23138=DIRECTION('center_axis',(-1.,0.,0.));
#23139=DIRECTION('ref_axis',(0.,1.,0.));
#23140=DIRECTION('',(1.,0.,0.));
#23141=DIRECTION('center_axis',(1.,0.,0.));
#23142=DIRECTION('ref_axis',(0.,0.,-1.));
#23143=DIRECTION('',(-1.,0.,0.));
#23144=DIRECTION('center_axis',(-1.,0.,0.));
#23145=DIRECTION('ref_axis',(0.,1.,0.));
#23146=DIRECTION('',(1.,0.,0.));
#23147=DIRECTION('center_axis',(1.,0.,0.));
#23148=DIRECTION('ref_axis',(0.,0.,-1.));
#23149=DIRECTION('',(-1.,0.,0.));
#23150=DIRECTION('center_axis',(-1.,0.,0.));
#23151=DIRECTION('ref_axis',(0.,1.,0.));
#23152=DIRECTION('',(1.,0.,0.));
#23153=DIRECTION('center_axis',(1.,0.,0.));
#23154=DIRECTION('ref_axis',(0.,0.,-1.));
#23155=DIRECTION('',(-1.,0.,0.));
#23156=DIRECTION('center_axis',(-1.,0.,0.));
#23157=DIRECTION('ref_axis',(0.,1.,0.));
#23158=DIRECTION('',(1.,0.,0.));
#23159=DIRECTION('center_axis',(1.,0.,0.));
#23160=DIRECTION('ref_axis',(0.,0.,-1.));
#23161=DIRECTION('',(-1.,0.,0.));
#23162=DIRECTION('center_axis',(-1.,0.,0.));
#23163=DIRECTION('ref_axis',(0.,1.,0.));
#23164=DIRECTION('',(1.,0.,0.));
#23165=DIRECTION('center_axis',(1.,0.,0.));
#23166=DIRECTION('ref_axis',(0.,0.,-1.));
#23167=DIRECTION('',(-1.,0.,0.));
#23168=DIRECTION('center_axis',(-1.,0.,0.));
#23169=DIRECTION('ref_axis',(0.,1.,0.));
#23170=DIRECTION('',(1.,0.,0.));
#23171=DIRECTION('center_axis',(1.,0.,0.));
#23172=DIRECTION('ref_axis',(0.,0.,-1.));
#23173=DIRECTION('',(-1.,0.,0.));
#23174=DIRECTION('center_axis',(-1.,0.,0.));
#23175=DIRECTION('ref_axis',(0.,1.,0.));
#23176=DIRECTION('',(1.,0.,0.));
#23177=DIRECTION('center_axis',(1.,0.,0.));
#23178=DIRECTION('ref_axis',(0.,0.,-1.));
#23179=DIRECTION('',(-1.,0.,0.));
#23180=DIRECTION('center_axis',(-1.,0.,0.));
#23181=DIRECTION('ref_axis',(0.,1.,0.));
#23182=DIRECTION('',(1.,0.,0.));
#23183=DIRECTION('center_axis',(1.,0.,0.));
#23184=DIRECTION('ref_axis',(0.,0.,-1.));
#23185=DIRECTION('',(-1.,0.,0.));
#23186=DIRECTION('center_axis',(-1.,0.,0.));
#23187=DIRECTION('ref_axis',(0.,1.,0.));
#23188=DIRECTION('',(1.,0.,0.));
#23189=DIRECTION('center_axis',(1.,0.,0.));
#23190=DIRECTION('ref_axis',(0.,0.,-1.));
#23191=DIRECTION('',(-1.,0.,0.));
#23192=DIRECTION('center_axis',(-1.,0.,0.));
#23193=DIRECTION('ref_axis',(0.,1.,0.));
#23194=DIRECTION('',(1.,0.,0.));
#23195=DIRECTION('center_axis',(1.,0.,0.));
#23196=DIRECTION('ref_axis',(0.,0.,-1.));
#23197=DIRECTION('',(-1.,0.,0.));
#23198=DIRECTION('center_axis',(-1.,0.,0.));
#23199=DIRECTION('ref_axis',(0.,1.,0.));
#23200=DIRECTION('',(-1.,0.,0.));
#23201=DIRECTION('center_axis',(1.,0.,0.));
#23202=DIRECTION('ref_axis',(0.,0.,-1.));
#23203=DIRECTION('center_axis',(-1.,0.,0.));
#23204=DIRECTION('ref_axis',(0.,1.,0.));
#23205=DIRECTION('',(1.,0.,0.));
#23206=DIRECTION('center_axis',(1.,0.,0.));
#23207=DIRECTION('ref_axis',(0.,0.,-1.));
#23208=DIRECTION('',(-1.,0.,0.));
#23209=DIRECTION('center_axis',(-1.,0.,0.));
#23210=DIRECTION('ref_axis',(0.,1.,0.));
#23211=DIRECTION('',(1.,0.,0.));
#23212=DIRECTION('center_axis',(1.,0.,0.));
#23213=DIRECTION('ref_axis',(0.,0.,-1.));
#23214=DIRECTION('',(-1.,0.,0.));
#23215=DIRECTION('center_axis',(-1.,0.,0.));
#23216=DIRECTION('ref_axis',(0.,1.,0.));
#23217=DIRECTION('',(1.,0.,0.));
#23218=DIRECTION('center_axis',(1.,0.,0.));
#23219=DIRECTION('ref_axis',(0.,0.,-1.));
#23220=DIRECTION('',(-1.,0.,0.));
#23221=DIRECTION('center_axis',(-1.,0.,0.));
#23222=DIRECTION('ref_axis',(0.,1.,0.));
#23223=DIRECTION('',(1.,0.,0.));
#23224=DIRECTION('center_axis',(1.,0.,0.));
#23225=DIRECTION('ref_axis',(0.,0.,-1.));
#23226=DIRECTION('',(-1.,0.,0.));
#23227=DIRECTION('center_axis',(-1.,0.,0.));
#23228=DIRECTION('ref_axis',(0.,1.,0.));
#23229=DIRECTION('',(1.,0.,0.));
#23230=DIRECTION('center_axis',(1.,0.,0.));
#23231=DIRECTION('ref_axis',(0.,0.,-1.));
#23232=DIRECTION('',(-1.,0.,0.));
#23233=DIRECTION('center_axis',(-1.,0.,0.));
#23234=DIRECTION('ref_axis',(0.,1.,0.));
#23235=DIRECTION('',(1.,0.,0.));
#23236=DIRECTION('center_axis',(1.,0.,0.));
#23237=DIRECTION('ref_axis',(0.,0.,-1.));
#23238=DIRECTION('',(-1.,0.,0.));
#23239=DIRECTION('center_axis',(-1.,0.,0.));
#23240=DIRECTION('ref_axis',(0.,1.,0.));
#23241=DIRECTION('',(1.,0.,0.));
#23242=DIRECTION('center_axis',(1.,0.,0.));
#23243=DIRECTION('ref_axis',(0.,0.,-1.));
#23244=DIRECTION('',(-1.,0.,0.));
#23245=DIRECTION('center_axis',(-1.,0.,0.));
#23246=DIRECTION('ref_axis',(0.,1.,0.));
#23247=DIRECTION('',(1.,0.,0.));
#23248=DIRECTION('center_axis',(1.,0.,0.));
#23249=DIRECTION('ref_axis',(0.,0.,-1.));
#23250=DIRECTION('',(-1.,0.,0.));
#23251=DIRECTION('center_axis',(-1.,0.,0.));
#23252=DIRECTION('ref_axis',(0.,1.,0.));
#23253=DIRECTION('',(1.,0.,0.));
#23254=DIRECTION('center_axis',(1.,0.,0.));
#23255=DIRECTION('ref_axis',(0.,0.,-1.));
#23256=DIRECTION('',(-1.,0.,0.));
#23257=DIRECTION('center_axis',(-1.,0.,0.));
#23258=DIRECTION('ref_axis',(0.,1.,0.));
#23259=DIRECTION('',(1.,0.,0.));
#23260=DIRECTION('center_axis',(1.,0.,0.));
#23261=DIRECTION('ref_axis',(0.,0.,-1.));
#23262=DIRECTION('',(-1.,0.,0.));
#23263=DIRECTION('center_axis',(-1.,0.,0.));
#23264=DIRECTION('ref_axis',(0.,1.,0.));
#23265=DIRECTION('',(1.,0.,0.));
#23266=DIRECTION('center_axis',(1.,0.,0.));
#23267=DIRECTION('ref_axis',(0.,0.,-1.));
#23268=DIRECTION('',(-1.,0.,0.));
#23269=DIRECTION('center_axis',(-1.,0.,0.));
#23270=DIRECTION('ref_axis',(0.,1.,0.));
#23271=DIRECTION('',(1.,0.,0.));
#23272=DIRECTION('center_axis',(1.,0.,0.));
#23273=DIRECTION('ref_axis',(0.,0.,-1.));
#23274=DIRECTION('',(-1.,0.,0.));
#23275=DIRECTION('center_axis',(-1.,0.,0.));
#23276=DIRECTION('ref_axis',(0.,1.,0.));
#23277=DIRECTION('',(1.,0.,0.));
#23278=DIRECTION('center_axis',(1.,0.,0.));
#23279=DIRECTION('ref_axis',(0.,0.,-1.));
#23280=DIRECTION('',(-1.,0.,0.));
#23281=DIRECTION('center_axis',(-1.,0.,0.));
#23282=DIRECTION('ref_axis',(0.,1.,0.));
#23283=DIRECTION('',(1.,0.,0.));
#23284=DIRECTION('center_axis',(1.,0.,0.));
#23285=DIRECTION('ref_axis',(0.,0.,-1.));
#23286=DIRECTION('',(-1.,0.,0.));
#23287=DIRECTION('center_axis',(-1.,0.,0.));
#23288=DIRECTION('ref_axis',(0.,1.,0.));
#23289=DIRECTION('',(1.,0.,0.));
#23290=DIRECTION('center_axis',(1.,0.,0.));
#23291=DIRECTION('ref_axis',(0.,0.,-1.));
#23292=DIRECTION('',(-1.,0.,0.));
#23293=DIRECTION('center_axis',(-1.,0.,0.));
#23294=DIRECTION('ref_axis',(0.,1.,0.));
#23295=DIRECTION('',(1.,0.,0.));
#23296=DIRECTION('center_axis',(1.,0.,0.));
#23297=DIRECTION('ref_axis',(0.,0.,-1.));
#23298=DIRECTION('center_axis',(0.,-0.308804726034324,0.951125460272653));
#23299=DIRECTION('ref_axis',(0.,-0.951125460272653,-0.308804726034324));
#23300=DIRECTION('',(1.,0.,0.));
#23301=DIRECTION('',(0.,-0.951125460272653,-0.308804726034324));
#23302=DIRECTION('center_axis',(1.,0.,0.));
#23303=DIRECTION('ref_axis',(0.,-0.406736643075801,-0.913545457642601));
#23304=DIRECTION('',(0.,0.406940521720215,-0.913454657759256));
#23305=DIRECTION('center_axis',(0.,-0.913454657759256,-0.406940521720215));
#23306=DIRECTION('ref_axis',(0.,0.406940521720215,-0.913454657759256));
#23307=DIRECTION('center_axis',(0.,-0.104306499240628,0.994545199684843));
#23308=DIRECTION('ref_axis',(0.,-0.994545199684843,-0.104306499240628));
#23309=DIRECTION('',(1.,0.,0.));
#23310=DIRECTION('',(0.,-0.994545199684843,-0.104306499240628));
#23311=DIRECTION('center_axis',(1.,0.,0.));
#23312=DIRECTION('ref_axis',(0.,-0.587785252292473,-0.809016994374947));
#23313=DIRECTION('',(0.,0.208129992581907,-0.978101173799447));
#23314=DIRECTION('center_axis',(0.,-0.978101173799447,-0.208129992581907));
#23315=DIRECTION('ref_axis',(0.,0.208129992581907,-0.978101173799447));
#23316=DIRECTION('center_axis',(0.,0.104750422088,0.994498541513454));
#23317=DIRECTION('ref_axis',(0.,-0.994498541513453,0.104750422088));
#23318=DIRECTION('',(1.,0.,0.));
#23319=DIRECTION('',(0.,-0.994498541513453,0.104750422088));
#23320=DIRECTION('center_axis',(1.,0.,0.));
#23321=DIRECTION('ref_axis',(0.,-0.743144825477395,-0.669130606358858));
#23322=DIRECTION('',(0.,0.000223184049258973,-0.99999997509444));
#23323=DIRECTION('center_axis',(0.,-0.99999997509444,-0.000223184049258973));
#23324=DIRECTION('ref_axis',(0.,0.000223184049258973,-0.99999997509444));
#23325=DIRECTION('center_axis',(0.,0.309229247323088,0.950987524944463));
#23326=DIRECTION('ref_axis',(0.,-0.950987524944463,0.309229247323088));
#23327=DIRECTION('',(1.,0.,0.));
#23328=DIRECTION('',(0.,-0.950987524944463,0.309229247323088));
#23329=DIRECTION('center_axis',(1.,0.,0.));
#23330=DIRECTION('ref_axis',(0.,-0.866025403784439,-0.499999999999999));
#23331=DIRECTION('',(0.,-0.207693378697298,-0.978193978945537));
#23332=DIRECTION('center_axis',(0.,-0.978193978945537,0.207693378697298));
#23333=DIRECTION('ref_axis',(0.,-0.207693378697298,-0.978193978945537));
#23334=DIRECTION('center_axis',(0.,0.500193270603598,0.865913790190961));
#23335=DIRECTION('ref_axis',(0.,-0.865913790190961,0.500193270603598));
#23336=DIRECTION('',(1.,0.,0.));
#23337=DIRECTION('',(0.,-0.865913790190961,0.500193270603598));
#23338=DIRECTION('center_axis',(1.,0.,0.));
#23339=DIRECTION('ref_axis',(0.,-0.951056516295154,-0.309016994374947));
#23340=DIRECTION('',(0.,-0.406532744171377,-0.913636212021223));
#23341=DIRECTION('center_axis',(0.,-0.913636212021223,0.406532744171377));
#23342=DIRECTION('ref_axis',(0.,-0.406532744171377,-0.913636212021223));
#23343=DIRECTION('center_axis',(0.,0.669296447765122,0.742995467690745));
#23344=DIRECTION('ref_axis',(0.,-0.742995467690745,0.669296447765122));
#23345=DIRECTION('',(1.,0.,0.));
#23346=DIRECTION('',(0.,-0.742995467690745,0.669296447765122));
#23347=DIRECTION('center_axis',(1.,0.,0.));
#23348=DIRECTION('ref_axis',(0.,-0.994521895368273,-0.104528463267653));
#23349=DIRECTION('',(0.,-0.587604677964628,-0.809148158518627));
#23350=DIRECTION('center_axis',(0.,-0.809148158518627,0.587604677964628));
#23351=DIRECTION('ref_axis',(0.,-0.587604677964628,-0.809148158518627));
#23352=DIRECTION('center_axis',(0.,0.809148158518628,0.587604677964627));
#23353=DIRECTION('ref_axis',(0.,-0.587604677964627,0.809148158518628));
#23354=DIRECTION('',(1.,0.,0.));
#23355=DIRECTION('',(0.,-0.587604677964627,0.809148158518628));
#23356=DIRECTION('center_axis',(1.,0.,0.));
#23357=DIRECTION('ref_axis',(0.,-0.994521895368273,0.104528463267654));
#23358=DIRECTION('',(0.,-0.742995467690746,-0.669296447765121));
#23359=DIRECTION('center_axis',(0.,-0.669296447765121,0.742995467690746));
#23360=DIRECTION('ref_axis',(0.,-0.742995467690746,-0.669296447765121));
#23361=DIRECTION('center_axis',(0.,0.913636212021223,0.406532744171377));
#23362=DIRECTION('ref_axis',(0.,-0.406532744171377,0.913636212021223));
#23363=DIRECTION('',(1.,0.,0.));
#23364=DIRECTION('',(0.,-0.406532744171377,0.913636212021223));
#23365=DIRECTION('center_axis',(1.,0.,0.));
#23366=DIRECTION('ref_axis',(0.,-0.951056516295153,0.309016994374948));
#23367=DIRECTION('',(0.,-0.865913790190961,-0.500193270603598));
#23368=DIRECTION('center_axis',(0.,-0.500193270603598,0.865913790190961));
#23369=DIRECTION('ref_axis',(0.,-0.865913790190961,-0.500193270603598));
#23370=DIRECTION('center_axis',(0.,0.978193978945537,0.207693378697297));
#23371=DIRECTION('ref_axis',(0.,-0.207693378697296,0.978193978945537));
#23372=DIRECTION('',(1.,0.,0.));
#23373=DIRECTION('',(0.,-0.207693378697296,0.978193978945537));
#23374=DIRECTION('center_axis',(1.,0.,0.));
#23375=DIRECTION('ref_axis',(0.,-0.866025403784438,0.5));
#23376=DIRECTION('',(0.,-0.950987524944464,-0.309229247323087));
#23377=DIRECTION('center_axis',(0.,-0.309229247323087,0.950987524944464));
#23378=DIRECTION('ref_axis',(0.,-0.950987524944464,-0.309229247323087));
#23379=DIRECTION('center_axis',(0.,0.99999997509444,-0.000223184049259806));
#23380=DIRECTION('ref_axis',(0.,0.000223184049259806,0.99999997509444));
#23381=DIRECTION('',(1.,0.,0.));
#23382=DIRECTION('',(0.,0.000223184049259806,0.99999997509444));
#23383=DIRECTION('center_axis',(1.,0.,0.));
#23384=DIRECTION('ref_axis',(0.,-0.743144825477394,0.669130606358858));
#23385=DIRECTION('',(0.,-0.994498541513453,-0.104750422087999));
#23386=DIRECTION('center_axis',(0.,-0.104750422087999,0.994498541513454));
#23387=DIRECTION('ref_axis',(0.,-0.994498541513453,-0.104750422087999));
#23388=DIRECTION('center_axis',(0.,0.978101173799447,-0.208129992581908));
#23389=DIRECTION('ref_axis',(0.,0.208129992581907,0.978101173799446));
#23390=DIRECTION('',(1.,0.,0.));
#23391=DIRECTION('',(0.,0.208129992581907,0.978101173799446));
#23392=DIRECTION('center_axis',(1.,0.,0.));
#23393=DIRECTION('ref_axis',(0.,-0.587785252292473,0.809016994374947));
#23394=DIRECTION('',(0.,-0.994545199684843,0.104306499240628));
#23395=DIRECTION('center_axis',(0.,0.104306499240628,0.994545199684843));
#23396=DIRECTION('ref_axis',(0.,-0.994545199684843,0.104306499240628));
#23397=DIRECTION('center_axis',(0.,0.913454657759255,-0.406940521720216));
#23398=DIRECTION('ref_axis',(0.,0.406940521720216,0.913454657759255));
#23399=DIRECTION('',(1.,0.,0.));
#23400=DIRECTION('',(0.,0.406940521720216,0.913454657759255));
#23401=DIRECTION('center_axis',(1.,0.,0.));
#23402=DIRECTION('ref_axis',(0.,-0.4067366430758,0.913545457642601));
#23403=DIRECTION('',(0.,-0.951125460272653,0.308804726034325));
#23404=DIRECTION('center_axis',(0.,0.308804726034325,0.951125460272653));
#23405=DIRECTION('ref_axis',(0.,-0.951125460272653,0.308804726034325));
#23406=DIRECTION('center_axis',(0.,0.808885789933224,-0.587965797342077));
#23407=DIRECTION('ref_axis',(0.,0.587965797342077,0.808885789933224));
#23408=DIRECTION('',(1.,0.,0.));
#23409=DIRECTION('',(0.,0.587965797342077,0.808885789933224));
#23410=DIRECTION('center_axis',(1.,0.,0.));
#23411=DIRECTION('ref_axis',(0.,-0.207911690817759,0.978147600733806));
#23412=DIRECTION('',(0.,-0.86613697424022,0.499806704490842));
#23413=DIRECTION('center_axis',(0.,0.499806704490842,0.86613697424022));
#23414=DIRECTION('ref_axis',(0.,-0.86613697424022,0.499806704490842));
#23415=DIRECTION('center_axis',(0.,0.668964731622449,-0.743294146247167));
#23416=DIRECTION('ref_axis',(0.,0.743294146247167,0.668964731622449));
#23417=DIRECTION('',(1.,0.,0.));
#23418=DIRECTION('',(0.,0.743294146247167,0.668964731622449));
#23419=DIRECTION('center_axis',(1.,0.,0.));
#23420=DIRECTION('ref_axis',(0.,1.22464679914735E-16,1.));
#23421=DIRECTION('',(0.,-0.743294146247166,0.668964731622449));
#23422=DIRECTION('center_axis',(0.,0.66896473162245,0.743294146247167));
#23423=DIRECTION('ref_axis',(0.,-0.743294146247166,0.668964731622449));
#23424=DIRECTION('center_axis',(0.,0.499806704490841,-0.866136974240221));
#23425=DIRECTION('ref_axis',(0.,0.866136974240221,0.499806704490841));
#23426=DIRECTION('',(1.,0.,0.));
#23427=DIRECTION('',(0.,0.866136974240221,0.499806704490841));
#23428=DIRECTION('center_axis',(1.,0.,0.));
#23429=DIRECTION('ref_axis',(0.,0.20791169081776,0.978147600733805));
#23430=DIRECTION('',(0.,-0.587965797342076,0.808885789933224));
#23431=DIRECTION('center_axis',(0.,0.808885789933225,0.587965797342076));
#23432=DIRECTION('ref_axis',(0.,-0.587965797342076,0.808885789933224));
#23433=DIRECTION('center_axis',(0.,0.308804726034324,-0.951125460272653));
#23434=DIRECTION('ref_axis',(0.,0.951125460272653,0.308804726034324));
#23435=DIRECTION('',(1.,0.,0.));
#23436=DIRECTION('',(0.,0.951125460272653,0.308804726034324));
#23437=DIRECTION('center_axis',(1.,0.,0.));
#23438=DIRECTION('ref_axis',(0.,0.4067366430758,0.913545457642601));
#23439=DIRECTION('',(0.,-0.406940521720215,0.913454657759256));
#23440=DIRECTION('center_axis',(0.,0.913454657759256,0.406940521720215));
#23441=DIRECTION('ref_axis',(0.,-0.406940521720215,0.913454657759256));
#23442=DIRECTION('center_axis',(0.,0.104306499240628,-0.994545199684843));
#23443=DIRECTION('ref_axis',(0.,0.994545199684843,0.104306499240628));
#23444=DIRECTION('',(1.,0.,0.));
#23445=DIRECTION('',(0.,0.994545199684843,0.104306499240628));
#23446=DIRECTION('center_axis',(1.,0.,0.));
#23447=DIRECTION('ref_axis',(0.,0.587785252292473,0.809016994374947));
#23448=DIRECTION('',(0.,-0.208129992581907,0.978101173799447));
#23449=DIRECTION('center_axis',(0.,0.978101173799447,0.208129992581907));
#23450=DIRECTION('ref_axis',(0.,-0.208129992581907,0.978101173799447));
#23451=DIRECTION('center_axis',(0.,-0.104750422087999,-0.994498541513453));
#23452=DIRECTION('ref_axis',(0.,0.994498541513453,-0.104750422087999));
#23453=DIRECTION('',(1.,0.,0.));
#23454=DIRECTION('',(0.,0.994498541513453,-0.104750422087999));
#23455=DIRECTION('center_axis',(1.,0.,0.));
#23456=DIRECTION('ref_axis',(0.,0.743144825477394,0.669130606358858));
#23457=DIRECTION('',(0.,-0.000223184049259084,0.99999997509444));
#23458=DIRECTION('center_axis',(0.,0.99999997509444,0.000223184049259084));
#23459=DIRECTION('ref_axis',(0.,-0.000223184049259084,0.99999997509444));
#23460=DIRECTION('center_axis',(0.,-0.309229247323088,-0.950987524944464));
#23461=DIRECTION('ref_axis',(0.,0.950987524944463,-0.309229247323088));
#23462=DIRECTION('',(1.,0.,0.));
#23463=DIRECTION('',(0.,0.950987524944463,-0.309229247323088));
#23464=DIRECTION('center_axis',(1.,0.,0.));
#23465=DIRECTION('ref_axis',(0.,0.866025403784439,0.5));
#23466=DIRECTION('',(0.,0.207693378697297,0.978193978945537));
#23467=DIRECTION('center_axis',(0.,0.978193978945537,-0.207693378697297));
#23468=DIRECTION('ref_axis',(0.,0.207693378697297,0.978193978945537));
#23469=DIRECTION('center_axis',(0.,-0.500193270603598,-0.865913790190961));
#23470=DIRECTION('ref_axis',(0.,0.865913790190961,-0.500193270603598));
#23471=DIRECTION('',(1.,0.,0.));
#23472=DIRECTION('',(0.,0.865913790190961,-0.500193270603598));
#23473=DIRECTION('center_axis',(1.,0.,0.));
#23474=DIRECTION('ref_axis',(0.,0.951056516295154,0.309016994374947));
#23475=DIRECTION('',(0.,0.406532744171377,0.913636212021223));
#23476=DIRECTION('center_axis',(0.,0.913636212021223,-0.406532744171377));
#23477=DIRECTION('ref_axis',(0.,0.406532744171377,0.913636212021223));
#23478=DIRECTION('center_axis',(0.,-0.669296447765122,-0.742995467690745));
#23479=DIRECTION('ref_axis',(0.,0.742995467690745,-0.669296447765122));
#23480=DIRECTION('',(1.,0.,0.));
#23481=DIRECTION('',(0.,0.742995467690745,-0.669296447765122));
#23482=DIRECTION('center_axis',(1.,0.,0.));
#23483=DIRECTION('ref_axis',(0.,0.994521895368273,0.104528463267653));
#23484=DIRECTION('',(0.,0.587604677964628,0.809148158518628));
#23485=DIRECTION('center_axis',(0.,0.809148158518628,-0.587604677964628));
#23486=DIRECTION('ref_axis',(0.,0.587604677964628,0.809148158518628));
#23487=DIRECTION('center_axis',(0.,-0.809148158518628,-0.587604677964628));
#23488=DIRECTION('ref_axis',(0.,0.587604677964628,-0.809148158518628));
#23489=DIRECTION('',(1.,0.,0.));
#23490=DIRECTION('',(0.,0.587604677964628,-0.809148158518628));
#23491=DIRECTION('center_axis',(1.,0.,0.));
#23492=DIRECTION('ref_axis',(0.,0.994521895368273,-0.104528463267654));
#23493=DIRECTION('',(0.,0.742995467690746,0.669296447765122));
#23494=DIRECTION('center_axis',(0.,0.669296447765122,-0.742995467690746));
#23495=DIRECTION('ref_axis',(0.,0.742995467690746,0.669296447765122));
#23496=DIRECTION('center_axis',(0.,-0.913636212021223,-0.406532744171377));
#23497=DIRECTION('ref_axis',(0.,0.406532744171377,-0.913636212021223));
#23498=DIRECTION('',(1.,0.,0.));
#23499=DIRECTION('',(0.,0.406532744171377,-0.913636212021223));
#23500=DIRECTION('center_axis',(1.,0.,0.));
#23501=DIRECTION('ref_axis',(0.,0.951056516295154,-0.309016994374948));
#23502=DIRECTION('',(0.,0.865913790190961,0.500193270603598));
#23503=DIRECTION('center_axis',(0.,0.500193270603598,-0.865913790190961));
#23504=DIRECTION('ref_axis',(0.,0.865913790190961,0.500193270603598));
#23505=DIRECTION('center_axis',(0.,-0.978193978945537,-0.207693378697297));
#23506=DIRECTION('ref_axis',(0.,0.207693378697297,-0.978193978945537));
#23507=DIRECTION('',(1.,0.,0.));
#23508=DIRECTION('',(0.,0.207693378697297,-0.978193978945537));
#23509=DIRECTION('center_axis',(1.,0.,0.));
#23510=DIRECTION('ref_axis',(0.,0.866025403784439,-0.5));
#23511=DIRECTION('',(0.,0.950987524944464,0.309229247323087));
#23512=DIRECTION('center_axis',(0.,0.309229247323087,-0.950987524944464));
#23513=DIRECTION('ref_axis',(0.,0.950987524944464,0.309229247323087));
#23514=DIRECTION('center_axis',(0.,-0.99999997509444,0.000223184049259584));
#23515=DIRECTION('ref_axis',(0.,-0.000223184049259584,-0.99999997509444));
#23516=DIRECTION('',(1.,0.,0.));
#23517=DIRECTION('',(0.,-0.000223184049259584,-0.99999997509444));
#23518=DIRECTION('center_axis',(1.,0.,0.));
#23519=DIRECTION('ref_axis',(0.,0.743144825477394,-0.669130606358858));
#23520=DIRECTION('',(0.,0.994498541513454,0.104750422087999));
#23521=DIRECTION('center_axis',(0.,0.104750422087999,-0.994498541513454));
#23522=DIRECTION('ref_axis',(0.,0.994498541513454,0.104750422087999));
#23523=DIRECTION('center_axis',(0.,-0.978101173799447,0.208129992581907));
#23524=DIRECTION('ref_axis',(0.,-0.208129992581907,-0.978101173799446));
#23525=DIRECTION('',(1.,0.,0.));
#23526=DIRECTION('',(0.,-0.208129992581907,-0.978101173799446));
#23527=DIRECTION('center_axis',(1.,0.,0.));
#23528=DIRECTION('ref_axis',(0.,0.587785252292473,-0.809016994374947));
#23529=DIRECTION('',(0.,0.994545199684843,-0.104306499240628));
#23530=DIRECTION('center_axis',(0.,-0.104306499240628,-0.994545199684843));
#23531=DIRECTION('ref_axis',(0.,0.994545199684843,-0.104306499240628));
#23532=DIRECTION('center_axis',(0.,-0.913454657759256,0.406940521720216));
#23533=DIRECTION('ref_axis',(0.,-0.406940521720215,-0.913454657759256));
#23534=DIRECTION('',(1.,0.,0.));
#23535=DIRECTION('',(0.,-0.406940521720215,-0.913454657759256));
#23536=DIRECTION('center_axis',(1.,0.,0.));
#23537=DIRECTION('ref_axis',(0.,0.4067366430758,-0.913545457642601));
#23538=DIRECTION('',(0.,0.951125460272653,-0.308804726034325));
#23539=DIRECTION('center_axis',(0.,-0.308804726034325,-0.951125460272653));
#23540=DIRECTION('ref_axis',(0.,0.951125460272653,-0.308804726034325));
#23541=DIRECTION('center_axis',(0.,-0.808885789933224,0.587965797342076));
#23542=DIRECTION('ref_axis',(0.,-0.587965797342076,-0.808885789933224));
#23543=DIRECTION('',(1.,0.,0.));
#23544=DIRECTION('',(0.,-0.587965797342076,-0.808885789933224));
#23545=DIRECTION('center_axis',(1.,0.,0.));
#23546=DIRECTION('ref_axis',(0.,0.207911690817759,-0.978147600733806));
#23547=DIRECTION('',(0.,0.866136974240221,-0.499806704490842));
#23548=DIRECTION('center_axis',(0.,-0.499806704490842,-0.866136974240221));
#23549=DIRECTION('ref_axis',(0.,0.866136974240221,-0.499806704490842));
#23550=DIRECTION('center_axis',(0.,-0.668964731622449,0.743294146247167));
#23551=DIRECTION('ref_axis',(0.,-0.743294146247167,-0.668964731622449));
#23552=DIRECTION('',(1.,0.,0.));
#23553=DIRECTION('',(0.,-0.743294146247167,-0.668964731622449));
#23554=DIRECTION('center_axis',(1.,0.,0.));
#23555=DIRECTION('ref_axis',(0.,0.,-1.));
#23556=DIRECTION('',(0.,0.743294146247167,-0.668964731622449));
#23557=DIRECTION('center_axis',(0.,-0.668964731622449,-0.743294146247167));
#23558=DIRECTION('ref_axis',(0.,0.743294146247167,-0.668964731622449));
#23559=DIRECTION('center_axis',(-1.,0.,0.));
#23560=DIRECTION('ref_axis',(0.,0.,1.));
#23561=DIRECTION('center_axis',(1.,0.,0.));
#23562=DIRECTION('ref_axis',(0.,0.,-1.));
#23563=DIRECTION('center_axis',(1.,0.,0.));
#23564=DIRECTION('ref_axis',(0.,1.,0.));
#23565=DIRECTION('',(-0.707106781186548,0.707106781186547,8.65956056235493E-17));
#23566=DIRECTION('center_axis',(1.,0.,0.));
#23567=DIRECTION('ref_axis',(0.,1.,0.));
#23568=DIRECTION('center_axis',(1.,0.,0.));
#23569=DIRECTION('ref_axis',(0.,1.,0.));
#23570=DIRECTION('center_axis',(-1.,0.,0.));
#23571=DIRECTION('ref_axis',(0.,0.,1.));
#23572=DIRECTION('center_axis',(1.,0.,0.));
#23573=DIRECTION('ref_axis',(0.,0.,-1.));
#23574=DIRECTION('center_axis',(1.,0.,0.));
#23575=DIRECTION('ref_axis',(0.,1.,0.));
#23576=DIRECTION('',(-0.707106781186548,0.707106781186547,8.65956056235493E-17));
#23577=DIRECTION('center_axis',(-1.,0.,0.));
#23578=DIRECTION('ref_axis',(0.,1.,0.));
#23579=DIRECTION('center_axis',(1.,0.,0.));
#23580=DIRECTION('ref_axis',(0.,0.,-1.));
#23581=DIRECTION('',(-0.707106781186548,-0.707106781186547,-8.65956056235493E-17));
#23582=DIRECTION('center_axis',(1.,0.,0.));
#23583=DIRECTION('ref_axis',(0.,0.,-1.));
#35571=CARTESIAN_POINT('',(0.,0.,0.));
#35572=CARTESIAN_POINT('Origin',(-5.8,0.,0.));
#35573=CARTESIAN_POINT('',(-11.3916725037879,-2.45326874606972,0.00165903621109187));
#35574=CARTESIAN_POINT('',(-11.5073274962121,-2.45271280748372,0.00261884364159621));
#35575=CARTESIAN_POINT('',(-5.8,-2.4505,-3.00099698131059E-16));
#35576=CARTESIAN_POINT('',(-11.6495,1.0763698230184,2.20363939945498));
#35577=CARTESIAN_POINT('Ctrl Pts',(-11.3916725037879,-2.45326874606972,
0.00165903621109187));
#35578=CARTESIAN_POINT('Ctrl Pts',(-11.396350692832,-2.45391416980342,0.0913991870340253));
#35579=CARTESIAN_POINT('Ctrl Pts',(-11.401028881876,-2.44941587367896,0.181069995962132));
#35580=CARTESIAN_POINT('Ctrl Pts',(-11.4057070709201,-2.43955857964069,
0.270142727834855));
#35581=CARTESIAN_POINT('Ctrl Pts',(-11.447950430442,-2.35054866318539,1.07445640577286));
#35582=CARTESIAN_POINT('Ctrl Pts',(-11.4901937899639,-1.82457545773628,
1.83000392977773));
#35583=CARTESIAN_POINT('Ctrl Pts',(-11.5324371494858,-1.10120406205714,
2.19334617876553));
#35584=CARTESIAN_POINT('Ctrl Pts',(-11.5714580996572,-0.433012907147874,
2.52897194227881));
#35585=CARTESIAN_POINT('Ctrl Pts',(-11.6104790498286,0.403609217336298,
2.52994664001211));
#35586=CARTESIAN_POINT('Ctrl Pts',(-11.6495,1.07765118568551,2.20520362934388));
#35587=CARTESIAN_POINT('',(-11.6495,-1.07508846035132,2.20207516956607));
#35588=CARTESIAN_POINT('Origin',(-11.6495,0.,0.));
#35589=CARTESIAN_POINT('Ctrl Pts',(-11.6495,-1.07508846035132,2.20207516956607));
#35590=CARTESIAN_POINT('Ctrl Pts',(-11.6072566404781,-1.80568981079581,
1.84538385773644));
#35591=CARTESIAN_POINT('Ctrl Pts',(-11.5650132809561,-2.33864379958948,
1.09973146804981));
#35592=CARTESIAN_POINT('Ctrl Pts',(-11.5227699214342,-2.43617762455603,
0.297632529466726));
#35593=CARTESIAN_POINT('Ctrl Pts',(-11.5176224463602,-2.4480624021536,0.199894462702958));
#35594=CARTESIAN_POINT('Ctrl Pts',(-11.5124749712861,-2.4534820068687,0.10131827054319));
#35595=CARTESIAN_POINT('Ctrl Pts',(-11.5073274962121,-2.45271280748372,
0.00261884364159621));
#35596=CARTESIAN_POINT('Origin',(-5.8,0.,0.));
#35597=CARTESIAN_POINT('',(-10.5916725037879,-2.44690286424559,0.000985173157012215));
#35598=CARTESIAN_POINT('',(-10.7073274962121,-2.44679512213092,0.000865365862940725));
#35599=CARTESIAN_POINT('',(-5.8,-2.4505,-3.00099698131059E-16));
#35600=CARTESIAN_POINT('Ctrl Pts',(-10.5916725037879,-2.44690286424559,
0.000985173157012215));
#35601=CARTESIAN_POINT('Ctrl Pts',(-10.6095572023671,-2.44815484704989,
0.346377013341112));
#35602=CARTESIAN_POINT('Ctrl Pts',(-10.6274419009462,-2.37991493328307,
0.691295890238114));
#35603=CARTESIAN_POINT('Ctrl Pts',(-10.6453265995254,-2.23975584232974,
1.00397534838721));
#35604=CARTESIAN_POINT('Ctrl Pts',(-10.6875699590473,-1.90870240896011,
1.74251900945362));
#35605=CARTESIAN_POINT('Ctrl Pts',(-10.7298133185692,-1.1764143924686,2.30120007687742));
#35606=CARTESIAN_POINT('Ctrl Pts',(-10.7720566780912,-0.376649708717779,
2.42540263668847));
#35607=CARTESIAN_POINT('Ctrl Pts',(-10.8143000376131,0.423114975033042,
2.54960519649952));
#35608=CARTESIAN_POINT('Ctrl Pts',(-10.856543397135,1.29035632604318,2.23932924869781));
#35609=CARTESIAN_POINT('Ctrl Pts',(-10.8987867566569,1.82979774721867,1.63595568520028));
#35610=CARTESIAN_POINT('Ctrl Pts',(-10.9410301161789,2.36923916839415,1.03258212170276));
#35611=CARTESIAN_POINT('Ctrl Pts',(-10.9832734757008,2.58088065973499,0.13611094250942));
#35612=CARTESIAN_POINT('Ctrl Pts',(-11.0255168352227,2.36827281982661,-0.644796181245458));
#35613=CARTESIAN_POINT('Ctrl Pts',(-11.0677601947446,2.15566497991823,-1.42570330500034));
#35614=CARTESIAN_POINT('Ctrl Pts',(-11.1100035542666,1.51880780876064,-2.09104637331676));
#35615=CARTESIAN_POINT('Ctrl Pts',(-11.1522469137885,0.747943825078181,
-2.33770810284367));
#35616=CARTESIAN_POINT('Ctrl Pts',(-11.1944902733104,-0.0229201586042772,
-2.58436983237059));
#35617=CARTESIAN_POINT('Ctrl Pts',(-11.2367336328323,-0.927790954811604,
-2.412350223108));
#35618=CARTESIAN_POINT('Ctrl Pts',(-11.2789769923543,-1.55420303918453,
-1.89980050254114));
#35619=CARTESIAN_POINT('Ctrl Pts',(-11.3165421628322,-2.11124388548996,
-1.44401247220008));
#35620=CARTESIAN_POINT('Ctrl Pts',(-11.35410733331,-2.44808608834503,-0.718941185934915));
#35621=CARTESIAN_POINT('Ctrl Pts',(-11.3916725037879,-2.45326874606972,
0.00165903621109187));
#35622=CARTESIAN_POINT('Ctrl Pts',(-11.5073274962121,-2.45271280748372,
0.00261884364159621));
#35623=CARTESIAN_POINT('Ctrl Pts',(-11.4702316117642,-2.44716948166043,
-0.708670183063881));
#35624=CARTESIAN_POINT('Ctrl Pts',(-11.4331357273163,-2.12020852811566,
-1.42635944763925));
#35625=CARTESIAN_POINT('Ctrl Pts',(-11.3960398428684,-1.57526873372546,
-1.88288102370373));
#35626=CARTESIAN_POINT('Ctrl Pts',(-11.3537964833465,-0.954712356788896,
-2.40275015081152));
#35627=CARTESIAN_POINT('Ctrl Pts',(-11.3115531238246,-0.0514859417763487,
-2.58394291754756));
#35628=CARTESIAN_POINT('Ctrl Pts',(-11.2693097643027,0.722133127858049,
-2.34562133189025));
#35629=CARTESIAN_POINT('Ctrl Pts',(-11.2270664047807,1.49575219749244,-2.10729974623295));
#35630=CARTESIAN_POINT('Ctrl Pts',(-11.1848230452588,2.13976392174869,-1.44946380818232));
#35631=CARTESIAN_POINT('Ctrl Pts',(-11.1425796857369,2.36095443699346,-0.671056592573343));
#35632=CARTESIAN_POINT('Ctrl Pts',(-11.100336326215,2.58214495223823,0.107350623035637));
#35633=CARTESIAN_POINT('Ctrl Pts',(-11.058092966693,2.38051425847153,1.00632911620296));
#35634=CARTESIAN_POINT('Ctrl Pts',(-11.0158496071711,1.847797719222,1.61568322182738));
#35635=CARTESIAN_POINT('Ctrl Pts',(-10.9736062476492,1.31508117997247,2.22503732745181));
#35636=CARTESIAN_POINT('Ctrl Pts',(-10.9313628881273,0.451278795240105,
2.54476704553332));
#35637=CARTESIAN_POINT('Ctrl Pts',(-10.8891195286053,-0.349820928189299,
2.42938746378778));
#35638=CARTESIAN_POINT('Ctrl Pts',(-10.8468761690834,-1.15092065161871,
2.31400788204225));
#35639=CARTESIAN_POINT('Ctrl Pts',(-10.8046328095615,-1.88931771374515,
1.76351900046965));
#35640=CARTESIAN_POINT('Ctrl Pts',(-10.7623894500395,-2.22851142489181,
1.02869552114519));
#35641=CARTESIAN_POINT('Ctrl Pts',(-10.7440354654304,-2.37588502927285,
0.709427854401686));
#35642=CARTESIAN_POINT('Ctrl Pts',(-10.7256814808212,-2.44789913409454,
0.355362476156112));
#35643=CARTESIAN_POINT('Ctrl Pts',(-10.7073274962121,-2.44679512213092,
0.000865365862940725));
#35644=CARTESIAN_POINT('Origin',(-5.8,0.,0.));
#35645=CARTESIAN_POINT('',(-9.79167250378794,-2.44974976939592,-0.00219261657894043));
#35646=CARTESIAN_POINT('',(-9.90732749621206,-2.45001435398628,-0.00220888930837992));
#35647=CARTESIAN_POINT('',(-5.8,-2.4505,-3.00099698131059E-16));
#35648=CARTESIAN_POINT('Ctrl Pts',(-9.79167250378794,-2.44974976939592,
-0.00219261657894043));
#35649=CARTESIAN_POINT('Ctrl Pts',(-9.8227637119022,-2.44448661548819,0.596485312663463));
#35650=CARTESIAN_POINT('Ctrl Pts',(-9.85385492001645,-2.22318596315255,
1.19864597202315));
#35651=CARTESIAN_POINT('Ctrl Pts',(-9.88494612813071,-1.82480365830791,
1.64151179239929));
#35652=CARTESIAN_POINT('Ctrl Pts',(-9.92718948765264,-1.28352501551987,
2.24322980867486));
#35653=CARTESIAN_POINT('Ctrl Pts',(-9.96943284717457,-0.415346110241138,
2.55088277676885));
#35654=CARTESIAN_POINT('Ctrl Pts',(-10.0116762066965,0.384035657178238,
2.42424941641526));
#35655=CARTESIAN_POINT('Ctrl Pts',(-10.0539195662184,1.18341742459761,2.29761605606167));
#35656=CARTESIAN_POINT('Ctrl Pts',(-10.0961629257403,1.91400205415762,1.73669636726052));
#35657=CARTESIAN_POINT('Ctrl Pts',(-10.1384062852623,2.24280448406768,0.997144853200805));
#35658=CARTESIAN_POINT('Ctrl Pts',(-10.1806496447842,2.57160691397774,0.257593339141094));
#35659=CARTESIAN_POINT('Ctrl Pts',(-10.2228930043061,2.49862714423785,-0.660590000177178));
#35660=CARTESIAN_POINT('Ctrl Pts',(-10.2651363638281,2.05712805657016,-1.33891529767941));
#35661=CARTESIAN_POINT('Ctrl Pts',(-10.30737972335,1.61562896890247,-2.01724059518164));
#35662=CARTESIAN_POINT('Ctrl Pts',(-10.3496230828719,0.80561056330699,-2.45570785086783));
#35663=CARTESIAN_POINT('Ctrl Pts',(-10.3918664423938,-0.00373849514181471,
-2.45447576463479));
#35664=CARTESIAN_POINT('Ctrl Pts',(-10.4341098019158,-0.813087553590622,
-2.45324367840176));
#35665=CARTESIAN_POINT('Ctrl Pts',(-10.4763531614377,-1.62176726489275,
-2.01231225024949));
#35666=CARTESIAN_POINT('Ctrl Pts',(-10.5185965209596,-2.06119769541993,
-1.33264340881885));
#35667=CARTESIAN_POINT('Ctrl Pts',(-10.5429551819024,-2.31458513870779,
-0.940728015508654));
#35668=CARTESIAN_POINT('Ctrl Pts',(-10.5673138428452,-2.44519768456358,
-0.469432748074029));
#35669=CARTESIAN_POINT('Ctrl Pts',(-10.5916725037879,-2.44690286424559,
0.000985173157012215));
#35670=CARTESIAN_POINT('Ctrl Pts',(-10.7073274962121,-2.44679512213092,
0.000865365862940725));
#35671=CARTESIAN_POINT('Ctrl Pts',(-10.6834381212993,-2.44535815047224,
-0.460544761344943));
#35672=CARTESIAN_POINT('Ctrl Pts',(-10.6595487463865,-2.32004898097106,
-0.922686302325035));
#35673=CARTESIAN_POINT('Ctrl Pts',(-10.6356593714738,-2.07581002964994,
-1.30977971176545));
#35674=CARTESIAN_POINT('Ctrl Pts',(-10.5934160119518,-1.64392456309453,
-1.99427338827529));
#35675=CARTESIAN_POINT('Ctrl Pts',(-10.5511726524299,-0.84016326981684,
-2.44410266421862));
#35676=CARTESIAN_POINT('Ctrl Pts',(-10.508929292908,-0.0308758190729953,
-2.45427970781378));
#35677=CARTESIAN_POINT('Ctrl Pts',(-10.4666859333861,0.778411631670846,
-2.46445675140895));
#35678=CARTESIAN_POINT('Ctrl Pts',(-10.4244425738641,1.59322523988084,-2.03498156265595));
#35679=CARTESIAN_POINT('Ctrl Pts',(-10.3821992143422,2.04219679318729,-1.3615815498271));
#35680=CARTESIAN_POINT('Ctrl Pts',(-10.3399558548203,2.49116834649374,-0.68818153699824));
#35681=CARTESIAN_POINT('Ctrl Pts',(-10.2977124952984,2.57429784489666,0.229143299906478));
#35682=CARTESIAN_POINT('Ctrl Pts',(-10.2554691357764,2.2536932268818,0.972286250652608));
#35683=CARTESIAN_POINT('Ctrl Pts',(-10.2132257762545,1.93308860886695,1.71542920139874));
#35684=CARTESIAN_POINT('Ctrl Pts',(-10.1709824167326,1.20874987443433,2.28439026598628));
#35685=CARTESIAN_POINT('Ctrl Pts',(-10.1287390572107,0.410816991349512,
2.41985411814018));
#35686=CARTESIAN_POINT('Ctrl Pts',(-10.0864956976887,-0.387115891735307,
2.55531797029409));
#35687=CARTESIAN_POINT('Ctrl Pts',(-10.0442523381668,-1.25864292347232,
2.25728461001436));
#35688=CARTESIAN_POINT('Ctrl Pts',(-10.0020089786449,-1.80654156532024,
1.66158866780937));
#35689=CARTESIAN_POINT('Ctrl Pts',(-9.97044848450061,-2.21588286945397,
1.21653745719321));
#35690=CARTESIAN_POINT('Ctrl Pts',(-9.93888799035633,-2.44458276857899,
0.605338316737112));
#35691=CARTESIAN_POINT('Ctrl Pts',(-9.90732749621206,-2.45001435398628,
-0.00220888930837992));
#35692=CARTESIAN_POINT('Origin',(-5.8,0.,0.));
#35693=CARTESIAN_POINT('',(-8.99167250378794,-2.45422282275285,0.000713024433140873));
#35694=CARTESIAN_POINT('',(-9.10732749621206,-2.45409992352044,0.000866640446018732));
#35695=CARTESIAN_POINT('',(-5.8,-2.4505,-3.00099698131059E-16));
#35696=CARTESIAN_POINT('Ctrl Pts',(-8.99167250378794,-2.45422282275285,
0.000713024433140873));
#35697=CARTESIAN_POINT('Ctrl Pts',(-8.99372686191538,-2.45437476902073,
0.0400839655821273));
#35698=CARTESIAN_POINT('Ctrl Pts',(-8.99578122004282,-2.45350899743941,
0.0794480827888193));
#35699=CARTESIAN_POINT('Ctrl Pts',(-8.99783557817026,-2.45160453815159,
0.11876188335754));
#35700=CARTESIAN_POINT('Ctrl Pts',(-9.04007893769219,-2.41244351879692,
0.927163782429675));
#35701=CARTESIAN_POINT('Ctrl Pts',(-9.08232229721412,-1.93409539353615,
1.71429035642438));
#35702=CARTESIAN_POINT('Ctrl Pts',(-9.12456565673604,-1.23458105964887,
2.12138605820959));
#35703=CARTESIAN_POINT('Ctrl Pts',(-9.16680901625797,-0.535066725761605,
2.52848175999481));
#35704=CARTESIAN_POINT('Ctrl Pts',(-9.2090523757799,0.385613816752166,2.55554658957053));
#35705=CARTESIAN_POINT('Ctrl Pts',(-9.25129573530183,1.10783396964644,2.19024498177808));
#35706=CARTESIAN_POINT('Ctrl Pts',(-9.29353909482375,1.83005412254071,1.82494337398563));
#35707=CARTESIAN_POINT('Ctrl Pts',(-9.33578245434568,2.3538138858155,1.06727532882499));
#35708=CARTESIAN_POINT('Ctrl Pts',(-9.3780258138676,2.44039470189646,0.262569802819703));
#35709=CARTESIAN_POINT('Ctrl Pts',(-9.42026917338953,2.52697551797742,-0.542135723185592));
#35710=CARTESIAN_POINT('Ctrl Pts',(-9.46251253291146,2.17637738686455,-1.39387873003553));
#35711=CARTESIAN_POINT('Ctrl Pts',(-9.50475589243338,1.54839548150531,-1.90445284987471));
#35712=CARTESIAN_POINT('Ctrl Pts',(-9.54699925195531,0.920413576146068,
-2.41502696971389));
#35713=CARTESIAN_POINT('Ctrl Pts',(-9.58924261147723,0.0150478965404477,
-2.58443220254231));
#35714=CARTESIAN_POINT('Ctrl Pts',(-9.63148597099916,-0.755055156366603,
-2.33545730519316));
#35715=CARTESIAN_POINT('Ctrl Pts',(-9.67372933052108,-1.52515820927365,
-2.08648240784401));
#35716=CARTESIAN_POINT('Ctrl Pts',(-9.71597269004301,-2.15999863548214,
-1.41912738031729));
#35717=CARTESIAN_POINT('Ctrl Pts',(-9.75821604956493,-2.37022965843771,
-0.637558334325361));
#35718=CARTESIAN_POINT('Ctrl Pts',(-9.7693682009726,-2.42573017319607,-0.431225873197954));
#35719=CARTESIAN_POINT('Ctrl Pts',(-9.78052035238027,-2.4516376178528,-0.216933288179889));
#35720=CARTESIAN_POINT('Ctrl Pts',(-9.79167250378794,-2.44974976939592,
-0.00219261657894043));
#35721=CARTESIAN_POINT('Ctrl Pts',(-9.90732749621206,-2.45001435398628,
-0.00220888930837992));
#35722=CARTESIAN_POINT('Ctrl Pts',(-9.8966446308344,-2.45185288336507,-0.207856652080567));
#35723=CARTESIAN_POINT('Ctrl Pts',(-9.88596176545675,-2.42811056017536,
-0.413085996340104));
#35724=CARTESIAN_POINT('Ctrl Pts',(-9.87527890007909,-2.37713422124245,
-0.611311718253279));
#35725=CARTESIAN_POINT('Ctrl Pts',(-9.83303554055717,-2.17555798335793,
-1.39515763798067));
#35726=CARTESIAN_POINT('Ctrl Pts',(-9.79079218103525,-1.54813525563007,
-2.06949095330521));
#35727=CARTESIAN_POINT('Ctrl Pts',(-9.74854882151333,-0.780832223944534,
-2.32696561304611));
#35728=CARTESIAN_POINT('Ctrl Pts',(-9.7063054619914,-0.013529192258997,
-2.58444027278702));
#35729=CARTESIAN_POINT('Ctrl Pts',(-9.66406210246947,0.893654143384223,
-2.42505627694429));
#35730=CARTESIAN_POINT('Ctrl Pts',(-9.62181874294754,1.52724305817981,-1.92145707918132));
#35731=CARTESIAN_POINT('Ctrl Pts',(-9.57957538342561,2.1608319729754,-1.41785788141836));
#35732=CARTESIAN_POINT('Ctrl Pts',(-9.53733202390369,2.52082646692336,-0.570043481735153));
#35733=CARTESIAN_POINT('Ctrl Pts',(-9.49508866438176,2.44314863923228,0.235570158161625));
#35734=CARTESIAN_POINT('Ctrl Pts',(-9.45284530485984,2.36547081154121,1.04118379805841));
#35735=CARTESIAN_POINT('Ctrl Pts',(-9.41060194533792,1.85012066221109,1.80459667816875));
#35736=CARTESIAN_POINT('Ctrl Pts',(-9.36835858581599,1.13198386014999,2.17786155730722));
#35737=CARTESIAN_POINT('Ctrl Pts',(-9.32611522629406,0.413847058088879,
2.55112643644568));
#35738=CARTESIAN_POINT('Ctrl Pts',(-9.28387186677213,-0.507076396703215,
2.53424331461225));
#35739=CARTESIAN_POINT('Ctrl Pts',(-9.2416285072502,-1.21104920978698,2.13490710462407));
#35740=CARTESIAN_POINT('Ctrl Pts',(-9.19938514772828,-1.91502202287073,
1.73557089463589));
#35741=CARTESIAN_POINT('Ctrl Pts',(-9.15714178820636,-2.40204419424616,
0.953781596492964));
#35742=CARTESIAN_POINT('Ctrl Pts',(-9.11489842868443,-2.45014137152306,
0.145862165020361));
#35743=CARTESIAN_POINT('Ctrl Pts',(-9.11237478452698,-2.45301472633666,
0.0975965636097421));
#35744=CARTESIAN_POINT('Ctrl Pts',(-9.10985114036952,-2.45432158385657,
0.0492377053017148));
#35745=CARTESIAN_POINT('Ctrl Pts',(-9.10732749621206,-2.45409992352044,
0.000866640446018732));
#35746=CARTESIAN_POINT('Origin',(-5.8,0.,0.));
#35747=CARTESIAN_POINT('',(-8.19167250378794,-2.44773723643955,0.00164077392830378));
#35748=CARTESIAN_POINT('',(-8.30732749621206,-2.44755708223661,0.00153710713373167));
#35749=CARTESIAN_POINT('',(-5.8,-2.4505,-3.00099698131059E-16));
#35750=CARTESIAN_POINT('Ctrl Pts',(-8.19167250378794,-2.44773723643955,
0.00164077392830378));
#35751=CARTESIAN_POINT('Ctrl Pts',(-8.2069333714505,-2.44955903509693,0.296108357714686));
#35752=CARTESIAN_POINT('Ctrl Pts',(-8.22219423911305,-2.40039019594895,
0.58998802961355));
#35753=CARTESIAN_POINT('Ctrl Pts',(-8.2374551067756,-2.2975061320399,0.863675152607228));
#35754=CARTESIAN_POINT('Ctrl Pts',(-8.27969846629752,-2.01271442839045,
1.62126402558554));
#35755=CARTESIAN_POINT('Ctrl Pts',(-8.32194182581944,-1.31634122677491,
2.22413178247212));
#35756=CARTESIAN_POINT('Ctrl Pts',(-8.36418518534137,-0.525778614071979,
2.39750412827805));
#35757=CARTESIAN_POINT('Ctrl Pts',(-8.4064285448633,0.264783998630956,2.57087647408397));
#35758=CARTESIAN_POINT('Ctrl Pts',(-8.44867190438523,1.14953602242128,2.31475340880925));
#35759=CARTESIAN_POINT('Ctrl Pts',(-8.49091526390716,1.72522631191578,1.7458703756214));
#35760=CARTESIAN_POINT('Ctrl Pts',(-8.53315862342908,2.30091660141027,1.17698734243355));
#35761=CARTESIAN_POINT('Ctrl Pts',(-8.57540198295101,2.56754515660894,0.295344341332577));
#35762=CARTESIAN_POINT('Ctrl Pts',(-8.61764534247293,2.40358835570123,-0.497224508978201));
#35763=CARTESIAN_POINT('Ctrl Pts',(-8.65988870199485,2.23963155479353,-1.28979335928898));
#35764=CARTESIAN_POINT('Ctrl Pts',(-8.70213206151678,1.64508939777945,-1.99328805880957));
#35765=CARTESIAN_POINT('Ctrl Pts',(-8.74437542103871,0.890941548410939,
-2.28707069285046));
#35766=CARTESIAN_POINT('Ctrl Pts',(-8.78661878056064,0.136793699042435,
-2.58085332689134));
#35767=CARTESIAN_POINT('Ctrl Pts',(-8.82886214008257,-0.776959842680494,
-2.46492389545253));
#35768=CARTESIAN_POINT('Ctrl Pts',(-8.87110549960449,-1.43384965681767,
-1.99212056765834));
#35769=CARTESIAN_POINT('Ctrl Pts',(-8.91129450099898,-2.05879393102198,
-1.54231037701346));
#35770=CARTESIAN_POINT('Ctrl Pts',(-8.95148350239346,-2.45125032799142,
-0.769492903931247));
#35771=CARTESIAN_POINT('Ctrl Pts',(-8.99167250378794,-2.45422282275285,
0.000713024433140873));
#35772=CARTESIAN_POINT('Ctrl Pts',(-9.10732749621206,-2.45409992352044,
0.000866640446018732));
#35773=CARTESIAN_POINT('Ctrl Pts',(-9.0676077808476,-2.45061120446613,-0.760447082120007));
#35774=CARTESIAN_POINT('Ctrl Pts',(-9.02788806548312,-2.06848244655717,
-1.5247845755012));
#35775=CARTESIAN_POINT('Ctrl Pts',(-8.98816835011865,-1.45578892873754,
-1.97614450095185));
#35776=CARTESIAN_POINT('Ctrl Pts',(-8.94592499059672,-0.804167125496714,
-2.45618217064918));
#35777=CARTESIAN_POINT('Ctrl Pts',(-8.9036816310748,0.108248664163322,-2.58220794524156));
#35778=CARTESIAN_POINT('Ctrl Pts',(-8.86143827155288,0.865598741831909,
-2.29678195051135));
#35779=CARTESIAN_POINT('Ctrl Pts',(-8.81919491203095,1.62294881950049,-2.01135595578114));
#35780=CARTESIAN_POINT('Ctrl Pts',(-8.77695155250902,2.22523318517763,-1.31447819172835));
#35781=CARTESIAN_POINT('Ctrl Pts',(-8.7347081929871,2.39794343978572,-0.523770718190494));
#35782=CARTESIAN_POINT('Ctrl Pts',(-8.69246483346517,2.5706536943938,0.266936755347366));
#35783=CARTESIAN_POINT('Ctrl Pts',(-8.65022147394324,2.31378983793283,1.1514739383703));
#35784=CARTESIAN_POINT('Ctrl Pts',(-8.60797811442132,1.74442495103308,1.72668760749301));
#35785=CARTESIAN_POINT('Ctrl Pts',(-8.56573475489939,1.17506006413332,2.30190127661573));
#35786=CARTESIAN_POINT('Ctrl Pts',(-8.52349139537747,0.293194146794787,
2.56779143183821));
#35787=CARTESIAN_POINT('Ctrl Pts',(-8.48124803585554,-0.499237081881421,
2.40317099726176));
#35788=CARTESIAN_POINT('Ctrl Pts',(-8.43900467633361,-1.29166831055762,
2.23855056268531));
#35789=CARTESIAN_POINT('Ctrl Pts',(-8.39676131681168,-1.99466485057149,
1.64341953830992));
#35790=CARTESIAN_POINT('Ctrl Pts',(-8.35451795728976,-2.28781583814602,
0.889025981588753));
#35791=CARTESIAN_POINT('Ctrl Pts',(-8.33878780359719,-2.39697642910899,
0.608112561676078));
#35792=CARTESIAN_POINT('Ctrl Pts',(-8.32305764990463,-2.44930811877369,
0.305115909000908));
#35793=CARTESIAN_POINT('Ctrl Pts',(-8.30732749621206,-2.44755708223661,
0.00153710713373167));
#35794=CARTESIAN_POINT('Origin',(-5.8,0.,0.));
#35795=CARTESIAN_POINT('',(-7.39167250378794,-2.44838374609482,-0.00191884294465761));
#35796=CARTESIAN_POINT('',(-7.50732749621206,-2.44860963519768,-0.00198937388838829));
#35797=CARTESIAN_POINT('',(-5.8,-2.4505,-3.00099698131059E-16));
#35798=CARTESIAN_POINT('Ctrl Pts',(-7.39167250378794,-2.44838374609482,
-0.00191884294465761));
#35799=CARTESIAN_POINT('Ctrl Pts',(-7.4201398809856,-2.44433948481649,0.547011082099126));
#35800=CARTESIAN_POINT('Ctrl Pts',(-7.44860725818326,-2.26174822597498,
1.09838028801556));
#35801=CARTESIAN_POINT('Ctrl Pts',(-7.47707463538092,-1.92273537771643,
1.52563359404597));
#35802=CARTESIAN_POINT('Ctrl Pts',(-7.51931799490285,-1.41966684660092,
2.15964405761116));
#35803=CARTESIAN_POINT('Ctrl Pts',(-7.56156135442478,-0.572154269872277,
2.52034836925077));
#35804=CARTESIAN_POINT('Ctrl Pts',(-7.60380471394671,0.233524154591539,
2.44334517930432));
#35805=CARTESIAN_POINT('Ctrl Pts',(-7.64604807346863,1.03920257905534,2.36634198935787));
#35806=CARTESIAN_POINT('Ctrl Pts',(-7.68829143299055,1.80304685125432,1.85163129782536));
#35807=CARTESIAN_POINT('Ctrl Pts',(-7.73053479251248,2.17691300610121,1.13380728515424));
#35808=CARTESIAN_POINT('Ctrl Pts',(-7.7727781520344,2.5507791609481,0.415983272483111));
#35809=CARTESIAN_POINT('Ctrl Pts',(-7.81502151155633,2.53466719844291,-0.504954061326639));
#35810=CARTESIAN_POINT('Ctrl Pts',(-7.85726487107826,2.1359206082407,-1.20926107656453));
#35811=CARTESIAN_POINT('Ctrl Pts',(-7.89950823060019,1.73717401803849,-1.91356809180241));
#35812=CARTESIAN_POINT('Ctrl Pts',(-7.94175159012211,0.955792800139277,
-2.40124478846844));
#35813=CARTESIAN_POINT('Ctrl Pts',(-7.98399494964404,0.147913886306987,
-2.45001850569757));
#35814=CARTESIAN_POINT('Ctrl Pts',(-8.02623830916596,-0.659965027525304,
-2.4987922229267));
#35815=CARTESIAN_POINT('Ctrl Pts',(-8.06848166868789,-1.49434163729067,
-2.10866296071894));
#35816=CARTESIAN_POINT('Ctrl Pts',(-8.11072502820981,-1.97492483933168,
-1.45744333508004));
#35817=CARTESIAN_POINT('Ctrl Pts',(-8.13770752006919,-2.28189219428585,
-1.04148379856765));
#35818=CARTESIAN_POINT('Ctrl Pts',(-8.16469001192857,-2.44451614386937,
-0.519002570739646));
#35819=CARTESIAN_POINT('Ctrl Pts',(-8.19167250378794,-2.44773723643955,
0.00164077392830378));
#35820=CARTESIAN_POINT('Ctrl Pts',(-8.30732749621206,-2.44755708223661,
0.00153710713373167));
#35821=CARTESIAN_POINT('Ctrl Pts',(-8.2808142903827,-2.44460570661564,-0.510145576751263));
#35822=CARTESIAN_POINT('Ctrl Pts',(-8.25430108455334,-2.28800979144261,
-1.02348209820766));
#35823=CARTESIAN_POINT('Ctrl Pts',(-8.22778787872398,-1.99091904313351,
-1.43551728262218));
#35824=CARTESIAN_POINT('Ctrl Pts',(-8.18554451920205,-1.5175658254113,-2.09201090104497));
#35825=CARTESIAN_POINT('Ctrl Pts',(-8.14330115968013,-0.687553954831687,
-2.49134204882359));
#35826=CARTESIAN_POINT('Ctrl Pts',(-8.1010578001582,0.12081482024383,-2.45150408617989));
#35827=CARTESIAN_POINT('Ctrl Pts',(-8.05881444063628,0.92918359531935,-2.4116661235362));
#35828=CARTESIAN_POINT('Ctrl Pts',(-8.01657108111435,1.71590927489077,-1.93265905047019));
#35829=CARTESIAN_POINT('Ctrl Pts',(-7.97432772159243,2.12241903526266,-1.23280409796831));
#35830=CARTESIAN_POINT('Ctrl Pts',(-7.9320843620705,2.52892879563455,-0.532949145466433));
#35831=CARTESIAN_POINT('Ctrl Pts',(-7.88984100254857,2.5552226368069,0.38775368647133));
#35832=CARTESIAN_POINT('Ctrl Pts',(-7.84759764302664,2.1893163855078,1.10966763913623));
#35833=CARTESIAN_POINT('Ctrl Pts',(-7.80535428350472,1.82341013420869,1.83158159180114));
#35834=CARTESIAN_POINT('Ctrl Pts',(-7.7631109239828,1.06530379043812,2.3547066651932));
#35835=CARTESIAN_POINT('Ctrl Pts',(-7.72086756446087,0.260526093597759,
2.4406135826465));
#35836=CARTESIAN_POINT('Ctrl Pts',(-7.67862420493894,-0.544251603242596,
2.52652050009981));
#35837=CARTESIAN_POINT('Ctrl Pts',(-7.63638084541701,-1.39570065315274,
2.17520926161437));
#35838=CARTESIAN_POINT('Ctrl Pts',(-7.59413748589509,-1.90574869754042,
1.54680005399698));
#35839=CARTESIAN_POINT('Ctrl Pts',(-7.56520082266741,-2.25513114859099,
1.11634031273146));
#35840=CARTESIAN_POINT('Ctrl Pts',(-7.53626415943974,-2.44432013405833,
0.555859618793608));
#35841=CARTESIAN_POINT('Ctrl Pts',(-7.50732749621206,-2.44860963519768,
-0.00198937388838829));
#35842=CARTESIAN_POINT('Origin',(-5.8,0.,0.));
#35843=CARTESIAN_POINT('',(-6.59167250378794,-2.45445842439397,-0.000201612658930761));
#35844=CARTESIAN_POINT('',(-6.70732749621206,-2.45447886332923,-3.55310500964387E-5));
#35845=CARTESIAN_POINT('',(-5.8,-2.4505,-3.00099698131059E-16));
#35846=CARTESIAN_POINT('Ctrl Pts',(-6.59167250378794,-2.45445842439397,
-0.000201612658930761));
#35847=CARTESIAN_POINT('Ctrl Pts',(-6.63334639052071,-2.45351233450644,
0.798256039998315));
#35848=CARTESIAN_POINT('Ctrl Pts',(-6.67502027725348,-2.02724189688927,
1.59758088060811));
#35849=CARTESIAN_POINT('Ctrl Pts',(-6.71669416398626,-1.36328849779505,
2.04105699768142));
#35850=CARTESIAN_POINT('Ctrl Pts',(-6.75893752350818,-0.690262189411743,
2.49059320660392));
#35851=CARTESIAN_POINT('Ctrl Pts',(-6.80118088303011,0.226987328759221,
2.57448891306526));
#35852=CARTESIAN_POINT('Ctrl Pts',(-6.84342424255203,0.970397244894051,
2.25450623931421));
#35853=CARTESIAN_POINT('Ctrl Pts',(-6.88566760207396,1.71380716102889,1.93452356556316));
#35854=CARTESIAN_POINT('Ctrl Pts',(-6.92791096159588,2.2833774751276,1.2106625115997));
#35855=CARTESIAN_POINT('Ctrl Pts',(-6.97015432111781,2.41951015816283,0.412843542460657));
#35856=CARTESIAN_POINT('Ctrl Pts',(-7.01239768063973,2.55564284119806,-0.384975426678379));
#35857=CARTESIAN_POINT('Ctrl Pts',(-7.05464104016167,2.25833789316983,-1.25675231099299));
#35858=CARTESIAN_POINT('Ctrl Pts',(-7.09688439968359,1.66310058290577,-1.80514975753896));
#35859=CARTESIAN_POINT('Ctrl Pts',(-7.13912775920552,1.06786327264172,-2.35354720408493));
#35860=CARTESIAN_POINT('Ctrl Pts',(-7.18137111872744,0.174693600141851,
-2.57856521286225));
#35861=CARTESIAN_POINT('Ctrl Pts',(-7.22361447824936,-0.609320704021191,
-2.37764536372776));
#35862=CARTESIAN_POINT('Ctrl Pts',(-7.26585783777129,-1.39333500818423,
-2.17672551459328));
#35863=CARTESIAN_POINT('Ctrl Pts',(-7.30810119729323,-2.06819394401045,
-1.549867807547));
#35864=CARTESIAN_POINT('Ctrl Pts',(-7.35034455681515,-2.32631116917237,
-0.782780646278478));
#35865=CARTESIAN_POINT('Ctrl Pts',(-7.36412053913942,-2.41048577961199,
-0.532625845751297));
#35866=CARTESIAN_POINT('Ctrl Pts',(-7.37789652146368,-2.45034085199531,
-0.267557960034949));
#35867=CARTESIAN_POINT('Ctrl Pts',(-7.39167250378794,-2.44838374609482,
-0.00191884294465761));
#35868=CARTESIAN_POINT('Ctrl Pts',(-7.50732749621206,-2.44860963519768,
-0.00198937388838829));
#35869=CARTESIAN_POINT('Ctrl Pts',(-7.49402079991781,-2.45058218775034,
-0.25851954342685));
#35870=CARTESIAN_POINT('Ctrl Pts',(-7.48071410362356,-2.41345451229918,
-0.514493193732628));
#35871=CARTESIAN_POINT('Ctrl Pts',(-7.46740740732931,-2.33482408253866,
-0.757010573783298));
#35872=CARTESIAN_POINT('Ctrl Pts',(-7.42516404780739,-2.08520438428399,
-1.52690481719685));
#35873=CARTESIAN_POINT('Ctrl Pts',(-7.38292068828546,-1.41731794890942,
-2.16118612727461));
#35874=CARTESIAN_POINT('Ctrl Pts',(-7.34067732876353,-0.63557320140634,
-2.37076258003248));
#35875=CARTESIAN_POINT('Ctrl Pts',(-7.2984339692416,0.146171546096736,-2.58033903279034));
#35876=CARTESIAN_POINT('Ctrl Pts',(-7.25619060971968,1.04177460572832,-2.36521062822831));
#35877=CARTESIAN_POINT('Ctrl Pts',(-7.21394725019776,1.64303916084166,-1.82342831533501));
#35878=CARTESIAN_POINT('Ctrl Pts',(-7.17170389067583,2.24430371595499,-1.28164600244171));
#35879=CARTESIAN_POINT('Ctrl Pts',(-7.1294605311539,2.55122976655008,-0.413209781217136));
#35880=CARTESIAN_POINT('Ctrl Pts',(-7.08721717163197,2.42392694998131,0.386065598544276));
#35881=CARTESIAN_POINT('Ctrl Pts',(-7.04497381211005,2.29662413341254,1.18534097830569));
#35882=CARTESIAN_POINT('Ctrl Pts',(-7.00273045258812,1.73509244967992,1.91545551660394));
#35883=CARTESIAN_POINT('Ctrl Pts',(-6.9604870930662,0.995266091147326,2.24363854331265));
#35884=CARTESIAN_POINT('Ctrl Pts',(-6.91824373354427,0.255439732614725,
2.57182157002137));
#35885=CARTESIAN_POINT('Ctrl Pts',(-6.87600037402234,-0.662681300717852,
2.49807308514054));
#35886=CARTESIAN_POINT('Ctrl Pts',(-6.83375701450042,-1.34063697896121,
2.05600607875245));
#35887=CARTESIAN_POINT('Ctrl Pts',(-6.79161384173763,-2.01698477887735,
1.61498750367272));
#35888=CARTESIAN_POINT('Ctrl Pts',(-6.74947066897485,-2.45430505252168,
0.807395385780097));
#35889=CARTESIAN_POINT('Ctrl Pts',(-6.70732749621206,-2.45447861156877,
-3.55288018881491E-5));
#35890=CARTESIAN_POINT('Origin',(-5.8,0.,0.));
#35891=CARTESIAN_POINT('',(-5.79167250378794,-2.44894776685357,0.00207433421441847));
#35892=CARTESIAN_POINT('',(-5.90732749621206,-2.44870895001949,0.00201676521443267));
#35893=CARTESIAN_POINT('',(-5.8,-2.4505,-3.00099698131059E-16));
#35894=CARTESIAN_POINT('Ctrl Pts',(-5.79167250378794,-2.44894776685357,
0.00207433421441847));
#35895=CARTESIAN_POINT('Ctrl Pts',(-5.80430954053389,-2.45092058764,0.245609603055973));
#35896=CARTESIAN_POINT('Ctrl Pts',(-5.81694657727985,-2.4175077934881,0.48861571488764));
#35897=CARTESIAN_POINT('Ctrl Pts',(-5.8295836140258,-2.34647756527096,0.720077934452022));
#35898=CARTESIAN_POINT('Ctrl Pts',(-5.87182697354773,-2.10903618341683,
1.49381484393203));
#35899=CARTESIAN_POINT('Ctrl Pts',(-5.91407033306966,-1.45124042784645,
2.13855503354418));
#35900=CARTESIAN_POINT('Ctrl Pts',(-5.95631369259159,-0.672899606421731,
2.36043964457516));
#35901=CARTESIAN_POINT('Ctrl Pts',(-5.99855705211351,0.105441215002987,
2.58232425560614));
#35902=CARTESIAN_POINT('Ctrl Pts',(-6.04080041163544,1.00432710228205,2.38135328805594));
#35903=CARTESIAN_POINT('Ctrl Pts',(-6.08304377115736,1.61406499578435,1.84912503238377));
#35904=CARTESIAN_POINT('Ctrl Pts',(-6.12528713067929,2.22380288928667,1.31689677671159));
#35905=CARTESIAN_POINT('Ctrl Pts',(-6.16753049020121,2.54439278901222,0.453411232917425));
#35906=CARTESIAN_POINT('Ctrl Pts',(-6.20977384972314,2.4297166406405,-0.347773262628461));
#35907=CARTESIAN_POINT('Ctrl Pts',(-6.25201720924507,2.31504049226878,-1.14895775817434));
#35908=CARTESIAN_POINT('Ctrl Pts',(-6.29426056876699,1.7650982957998,-1.88784120547194));
#35909=CARTESIAN_POINT('Ctrl Pts',(-6.33650392828892,1.03054200192067,-2.22765625227097));
#35910=CARTESIAN_POINT('Ctrl Pts',(-6.37874728781084,0.295985708041539,
-2.56747129907001));
#35911=CARTESIAN_POINT('Ctrl Pts',(-6.42099064733277,-0.623184683247735,
-2.50821794537048));
#35912=CARTESIAN_POINT('Ctrl Pts',(-6.4632340068547,-1.30803086703115,-2.07690260891029));
#35913=CARTESIAN_POINT('Ctrl Pts',(-6.50547736637662,-1.99287705081456,
-1.6455872724501));
#35914=CARTESIAN_POINT('Ctrl Pts',(-6.54772072589855,-2.44339902709211,
-0.842209953229236));
#35915=CARTESIAN_POINT('Ctrl Pts',(-6.58996408542048,-2.45425846593306,
-0.03293293792698));
#35916=CARTESIAN_POINT('Ctrl Pts',(-6.59053355820963,-2.45440485947267,
-0.0220232649199538));
#35917=CARTESIAN_POINT('Ctrl Pts',(-6.59110303099879,-2.45447135269246,
-0.0111125197551619));
#35918=CARTESIAN_POINT('Ctrl Pts',(-6.59167250378794,-2.45445842439397,
-0.000201612658930761));
#35919=CARTESIAN_POINT('Ctrl Pts',(-6.70732749621206,-2.45447861156877,
-3.55288018881219E-5));
#35920=CARTESIAN_POINT('Ctrl Pts',(-6.70722730945292,-2.45447902416985,
-0.00195503037850885));
#35921=CARTESIAN_POINT('Ctrl Pts',(-6.70712712269378,-2.45447696622223,
-0.00387453104408387));
#35922=CARTESIAN_POINT('Ctrl Pts',(-6.70702693593464,-2.45447243506411,
-0.00579402587139999));
#35923=CARTESIAN_POINT('Ctrl Pts',(-6.66478357641271,-2.45256188976951,
-0.815141596211808));
#35924=CARTESIAN_POINT('Ctrl Pts',(-6.62254021689079,-2.01095047602618,
-1.62345120899729));
#35925=CARTESIAN_POINT('Ctrl Pts',(-6.58029685736886,-1.33091527897354,
-2.06231254309822));
#35926=CARTESIAN_POINT('Ctrl Pts',(-6.53805349784693,-0.650880081920891,
-2.50117387719915));
#35927=CARTESIAN_POINT('Ctrl Pts',(-6.49581013832501,0.267578898441061,
-2.57058693261554));
#35928=CARTESIAN_POINT('Ctrl Pts',(-6.45356677880308,1.00584760315856,-2.23891471575975));
#35929=CARTESIAN_POINT('Ctrl Pts',(-6.41132341928116,1.74411630787607,-1.90724249890396));
#35930=CARTESIAN_POINT('Ctrl Pts',(-6.36908005975923,2.30219473694912,-1.17448500977598));
#35931=CARTESIAN_POINT('Ctrl Pts',(-6.32683670023731,2.42572261800414,-0.374617519249364));
#35932=CARTESIAN_POINT('Ctrl Pts',(-6.28459334071538,2.54925049905916,0.425249971277239));
#35933=CARTESIAN_POINT('Ctrl Pts',(-6.24234998119346,2.23822783209618,1.29222746320248));
#35934=CARTESIAN_POINT('Ctrl Pts',(-6.20010662167153,1.6344121303279,1.83116506450468));
#35935=CARTESIAN_POINT('Ctrl Pts',(-6.1578632621496,1.03059642855962,2.37010266580688));
#35936=CARTESIAN_POINT('Ctrl Pts',(-6.11561990262767,0.133987691986036,
2.58100037648602));
#35937=CARTESIAN_POINT('Ctrl Pts',(-6.07337654310574,-0.646758896596811,
2.36773550780029));
#35938=CARTESIAN_POINT('Ctrl Pts',(-6.03113318358382,-1.42750548517965,
2.15447063911456));
#35939=CARTESIAN_POINT('Ctrl Pts',(-5.98888982406189,-2.09238992577176,
1.51704319106397));
#35940=CARTESIAN_POINT('Ctrl Pts',(-5.94664646453997,-2.33837203872158,
0.74597903036914));
#35941=CARTESIAN_POINT('Ctrl Pts',(-5.933540141764,-2.41468985543694,0.506750524743217));
#35942=CARTESIAN_POINT('Ctrl Pts',(-5.92043381898803,-2.45068423041799,
0.254658179887264));
#35943=CARTESIAN_POINT('Ctrl Pts',(-5.90732749621206,-2.44870895001949,
0.00201676521443284));
#35944=CARTESIAN_POINT('Origin',(-5.8,0.,0.));
#35945=CARTESIAN_POINT('',(-4.99167250378794,-2.44732265144935,-0.00137759639247254));
#35946=CARTESIAN_POINT('',(-5.10732749621206,-2.44748408483923,-0.00149075522941132));
#35947=CARTESIAN_POINT('',(-5.8,-2.4505,-3.00099698131059E-16));
#35948=CARTESIAN_POINT('Ctrl Pts',(-4.99167250378794,-2.44732265144935,
-0.00137759639247254));
#35949=CARTESIAN_POINT('Ctrl Pts',(-5.01751605006901,-2.44475955460895,
0.497501199516291));
#35950=CARTESIAN_POINT('Ctrl Pts',(-5.04335959635007,-2.29653477948369,
0.9977790446417));
#35951=CARTESIAN_POINT('Ctrl Pts',(-5.06920314263114,-2.01332067653255,
1.40392629772763));
#35952=CARTESIAN_POINT('Ctrl Pts',(-5.11144650215306,-1.55038439671517,
2.06780672049767));
#35953=CARTESIAN_POINT('Ctrl Pts',(-5.15368986167499,-0.726776374453026,
2.48018396746088));
#35954=CARTESIAN_POINT('Ctrl Pts',(-5.19593322119691,0.0821203796264817,
2.45310526460945));
#35955=CARTESIAN_POINT('Ctrl Pts',(-5.23817658071884,0.89101713370599,2.42602656175802));
#35956=CARTESIAN_POINT('Ctrl Pts',(-5.28041994024077,1.68520261960285,1.95949190909194));
#35957=CARTESIAN_POINT('Ctrl Pts',(-5.3226632997627,2.10270399266982,1.266137873699));
#35958=CARTESIAN_POINT('Ctrl Pts',(-5.36490665928462,2.52020536573677,0.572783838306069));
#35959=CARTESIAN_POINT('Ctrl Pts',(-5.40715001880655,2.56102262597383,-0.347389579813734));
#35960=CARTESIAN_POINT('Ctrl Pts',(-5.44939337832847,2.20655213473348,-1.07498691745887));
#35961=CARTESIAN_POINT('Ctrl Pts',(-5.49163673785039,1.85208164349313,-1.80258425510401));
#35962=CARTESIAN_POINT('Ctrl Pts',(-5.53388009737232,1.10232340077537,-2.3376055122745));
#35963=CARTESIAN_POINT('Ctrl Pts',(-5.57612345689425,0.299001259173409,
-2.4361993849062));
#35964=CARTESIAN_POINT('Ctrl Pts',(-5.61836681641618,-0.504320882428552,
-2.53479325753789));
#35965=CARTESIAN_POINT('Ctrl Pts',(-5.66061017593811,-1.3612069229147,-2.19695974563081));
#35966=CARTESIAN_POINT('Ctrl Pts',(-5.70285353546003,-1.88110643908884,
-1.57667617500333));
#35967=CARTESIAN_POINT('Ctrl Pts',(-5.732459858236,-2.24547880580207,-1.14194949103548));
#35968=CARTESIAN_POINT('Ctrl Pts',(-5.76206618101197,-2.4443257996823,-0.568485356447488));
#35969=CARTESIAN_POINT('Ctrl Pts',(-5.79167250378794,-2.44894776685357,
0.00207433421441847));
#35970=CARTESIAN_POINT('Ctrl Pts',(-5.90732749621206,-2.44870895001949,
0.00201676521443267));
#35971=CARTESIAN_POINT('Ctrl Pts',(-5.8781904594661,-2.4443176483143,-0.559637507208111));
#35972=CARTESIAN_POINT('Ctrl Pts',(-5.84905342272015,-2.25226894435809,
-1.12400544701741));
#35973=CARTESIAN_POINT('Ctrl Pts',(-5.81991638597419,-1.89842474885524,
-1.55578018311049));
#35974=CARTESIAN_POINT('Ctrl Pts',(-5.77767302645226,-1.38541556073153,
-2.18177436255622));
#35975=CARTESIAN_POINT('Ctrl Pts',(-5.73542966693034,-0.532317399176566,
-2.52906184810862));
#35976=CARTESIAN_POINT('Ctrl Pts',(-5.69318630740841,0.27204574722632,-2.43935639393703));
#35977=CARTESIAN_POINT('Ctrl Pts',(-5.65094294788649,1.07640889362921,-2.34965093976544));
#35978=CARTESIAN_POINT('Ctrl Pts',(-5.60869958836456,1.83203702488002,-1.82295254586987));
#35979=CARTESIAN_POINT('Ctrl Pts',(-5.56645622884264,2.19453091810013,-1.09931913233965));
#35980=CARTESIAN_POINT('Ctrl Pts',(-5.52421286932071,2.55702481132025,-0.375685718809419));
#35981=CARTESIAN_POINT('Ctrl Pts',(-5.48196950979878,2.52638446650966,0.544882714355476));
#35982=CARTESIAN_POINT('Ctrl Pts',(-5.43972615027686,2.11657510082358,1.24281066450166));
#35983=CARTESIAN_POINT('Ctrl Pts',(-5.39748279075493,1.70676573513749,1.94073861464785));
#35984=CARTESIAN_POINT('Ctrl Pts',(-5.355239431233,0.917787348575927,2.41602608177533));
#35985=CARTESIAN_POINT('Ctrl Pts',(-5.31299607171108,0.109239500713276,
2.45204715221982));
#35986=CARTESIAN_POINT('Ctrl Pts',(-5.27075271218915,-0.699308347149369,
2.4880682226643));
#35987=CARTESIAN_POINT('Ctrl Pts',(-5.22850935266723,-1.52742565631309,
2.08482289642579));
#35988=CARTESIAN_POINT('Ctrl Pts',(-5.1862659931453,-1.99767417913586,1.42610181236799));
#35989=CARTESIAN_POINT('Ctrl Pts',(-5.15995316083422,-2.29058579093952,
1.01579312431041));
#35990=CARTESIAN_POINT('Ctrl Pts',(-5.13364032852314,-2.44464860689455,
0.506362907090105));
#35991=CARTESIAN_POINT('Ctrl Pts',(-5.10732749621206,-2.44748408483923,
-0.00149075522941132));
#35992=CARTESIAN_POINT('Origin',(-5.8,0.,0.));
#35993=CARTESIAN_POINT('',(-4.19167250378794,-2.45388990632559,-0.0010763688550719));
#35994=CARTESIAN_POINT('',(-4.30732749621206,-2.45404119041951,-0.000930649193247773));
#35995=CARTESIAN_POINT('',(-5.8,-2.4505,-3.00099698131059E-16));
#35996=CARTESIAN_POINT('Ctrl Pts',(-4.19167250378794,-2.45388990632559,
-0.0010763688550719));
#35997=CARTESIAN_POINT('Ctrl Pts',(-4.23072255960411,-2.4497607135484,0.747572201937431));
#35998=CARTESIAN_POINT('Ctrl Pts',(-4.26977261542029,-2.08207444069939,
1.49973049661193));
#35999=CARTESIAN_POINT('Ctrl Pts',(-4.30882267123646,-1.48678706708609,
1.95292944397715));
#36000=CARTESIAN_POINT('Ctrl Pts',(-4.35106603075839,-0.842820291192447,
2.44318856572151));
#36001=CARTESIAN_POINT('Ctrl Pts',(-4.39330939028032,0.0674935641221409,
2.58359459469071));
#36002=CARTESIAN_POINT('Ctrl Pts',(-4.43555274980224,0.829252814575512,
2.31015345064403));
#36003=CARTESIAN_POINT('Ctrl Pts',(-4.47779610932417,1.59101206502888,2.03671230659736));
#36004=CARTESIAN_POINT('Ctrl Pts',(-4.5200394688461,2.20421671062104,1.3494239895348));
#36005=CARTESIAN_POINT('Ctrl Pts',(-4.56228282836802,2.38938112254485,0.56153988926041));
#36006=CARTESIAN_POINT('Ctrl Pts',(-4.60452618788995,2.57454553446865,-0.226344211013978));
#36007=CARTESIAN_POINT('Ctrl Pts',(-4.64676954741187,2.3316697127241,-1.11482409450023));
#36008=CARTESIAN_POINT('Ctrl Pts',(-4.6890129069338,1.77145128859989,-1.69894953666164));
#36009=CARTESIAN_POINT('Ctrl Pts',(-4.73125626645573,1.21123286447566,-2.28307497882307));
#36010=CARTESIAN_POINT('Ctrl Pts',(-4.77349962597765,0.333671837971791,
-2.56284597965965));
#36011=CARTESIAN_POINT('Ctrl Pts',(-4.81574298549958,-0.461258149040667,
-2.41074887036126));
#36012=CARTESIAN_POINT('Ctrl Pts',(-4.85798634502151,-1.2561881360531,-2.25865176106287));
#36013=CARTESIAN_POINT('Ctrl Pts',(-4.90022970454343,-1.96848708357411,
-1.67468654162951));
#36014=CARTESIAN_POINT('Ctrl Pts',(-4.94247306406536,-2.27350428864831,
-0.925012132624398));
#36015=CARTESIAN_POINT('Ctrl Pts',(-4.95887287730622,-2.3919187626645,-0.63397182621235));
#36016=CARTESIAN_POINT('Ctrl Pts',(-4.97527269054708,-2.44894914299364,
-0.317956404646919));
#36017=CARTESIAN_POINT('Ctrl Pts',(-4.99167250378794,-2.44732265144935,
-0.00137759639247254));
#36018=CARTESIAN_POINT('Ctrl Pts',(-5.10732749621206,-2.44748408483923,
-0.00149075522941132));
#36019=CARTESIAN_POINT('Ctrl Pts',(-5.09139696900121,-2.4492007627711,-0.308959616470236));
#36020=CARTESIAN_POINT('Ctrl Pts',(-5.07546644179037,-2.39548609667096,
-0.615850602320005));
#36021=CARTESIAN_POINT('Ctrl Pts',(-5.05953591457952,-2.28359309607109,
-0.899817246334982));
#36022=CARTESIAN_POINT('Ctrl Pts',(-5.01729255505759,-1.98688375370171,
-1.65281837910306));
#36023=CARTESIAN_POINT('Ctrl Pts',(-4.97504919553567,-1.28108533248114,
-2.24462380276213));
#36024=CARTESIAN_POINT('Ctrl Pts',(-4.93280583601374,-0.487885733804657,
-2.40550119849799));
#36025=CARTESIAN_POINT('Ctrl Pts',(-4.89056247649182,0.305313864871833,
-2.56637859423385));
#36026=CARTESIAN_POINT('Ctrl Pts',(-4.84831911696989,1.18591464100422,-2.2963279620465));
#36027=CARTESIAN_POINT('Ctrl Pts',(-4.80607575744796,1.7525574995251,-1.71843263355995));
#36028=CARTESIAN_POINT('Ctrl Pts',(-4.76383239792604,2.31920035804599,-1.14053730507339));
#36029=CARTESIAN_POINT('Ctrl Pts',(-4.72158903840411,2.57188529895534,-0.254797280287638));
#36030=CARTESIAN_POINT('Ctrl Pts',(-4.67934567888219,2.39544390318143,0.535085985553977));
#36031=CARTESIAN_POINT('Ctrl Pts',(-4.63710231936026,2.21900250740753,1.32496925139559));
#36032=CARTESIAN_POINT('Ctrl Pts',(-4.59485895983833,1.61343477495037,2.01899575829307));
#36033=CARTESIAN_POINT('Ctrl Pts',(-4.55261560031641,0.854745592120015,
2.30084299289993));
#36034=CARTESIAN_POINT('Ctrl Pts',(-4.51037224079448,0.0960564092896574,
2.58269022750678));
#36035=CARTESIAN_POINT('Ctrl Pts',(-4.46812888127256,-0.815754223913907,
2.45235818982303));
#36036=CARTESIAN_POINT('Ctrl Pts',(-4.42588552175063,-1.46510242369844,
1.96924944923155));
#36037=CARTESIAN_POINT('Ctrl Pts',(-4.38636617990444,-2.07257810212248,
1.51729345699076));
#36038=CARTESIAN_POINT('Ctrl Pts',(-4.34684683805825,-2.45034919829134,
0.756590707680147));
#36039=CARTESIAN_POINT('Ctrl Pts',(-4.30732749621206,-2.45404119041951,
-0.000930649193247773));
#36040=CARTESIAN_POINT('Origin',(-5.8,0.,0.));
#36041=CARTESIAN_POINT('',(-3.39167250378793,-2.45039822849204,0.0022139813149212));
#36042=CARTESIAN_POINT('',(-3.50732749621206,-2.45012855430742,0.00221267815828837));
#36043=CARTESIAN_POINT('',(-5.8,-2.4505,-3.00099698131059E-16));
#36044=CARTESIAN_POINT('Ctrl Pts',(-3.39167250378793,-2.45039822849204,
0.0022139813149212));
#36045=CARTESIAN_POINT('Ctrl Pts',(-3.40168570961729,-2.45214961691583,
0.194893485098156));
#36046=CARTESIAN_POINT('Ctrl Pts',(-3.41169891544666,-2.43132697024435,
0.387198851168568));
#36047=CARTESIAN_POINT('Ctrl Pts',(-3.42171212127602,-2.38648354955538,
0.573729434054478));
#36048=CARTESIAN_POINT('Ctrl Pts',(-3.46395548079794,-2.19729970827227,
1.3606580769851));
#36049=CARTESIAN_POINT('Ctrl Pts',(-3.50619884031987,-1.58059471251749,
2.04480726859311));
#36050=CARTESIAN_POINT('Ctrl Pts',(-3.5484421998418,-0.817449576101223,
2.3143563655275));
#36051=CARTESIAN_POINT('Ctrl Pts',(-3.59068555936372,-0.0543044396849619,
2.58390546246189));
#36052=CARTESIAN_POINT('Ctrl Pts',(-3.63292891888565,0.855280837392778,
2.43885446472266));
#36053=CARTESIAN_POINT('Ctrl Pts',(-3.67517227840757,1.49673664124676,1.94531453054292));
#36054=CARTESIAN_POINT('Ctrl Pts',(-3.7174156379295,2.13819244510074,1.45177459636318));
#36055=CARTESIAN_POINT('Ctrl Pts',(-3.75965899745143,2.51151877573097,0.609745725742923));
#36056=CARTESIAN_POINT('Ctrl Pts',(-3.80190235697336,2.4465614358444,-0.196993240029851));
#36057=CARTESIAN_POINT('Ctrl Pts',(-3.84414571649528,2.38160409595783,-1.00373220580262));
#36058=CARTESIAN_POINT('Ctrl Pts',(-3.8863890760172,1.87836308555447,-1.77518126672792));
#36059=CARTESIAN_POINT('Ctrl Pts',(-3.92863243553913,1.16620494847117,-2.15973035682336));
#36060=CARTESIAN_POINT('Ctrl Pts',(-3.97087579506105,0.454046811387868,
-2.5442794469188));
#36061=CARTESIAN_POINT('Ctrl Pts',(-4.01311915458298,-0.467028452375371,
-2.54192856618438));
#36062=CARTESIAN_POINT('Ctrl Pts',(-4.05536251410491,-1.17721433755474,
-2.15374919604323));
#36063=CARTESIAN_POINT('Ctrl Pts',(-4.09760587362684,-1.88740022273411,
-1.76556982590208));
#36064=CARTESIAN_POINT('Ctrl Pts',(-4.13984923314876,-2.38669672932962,
-0.991561966354189));
#36065=CARTESIAN_POINT('Ctrl Pts',(-4.18209259267069,-2.44753513439102,
-0.184501929320475));
#36066=CARTESIAN_POINT('Ctrl Pts',(-4.18528589637644,-2.45213409400345,
-0.123493812632109));
#36067=CARTESIAN_POINT('Ctrl Pts',(-4.18847920008219,-2.45422756952021,
-0.0622968256623468));
#36068=CARTESIAN_POINT('Ctrl Pts',(-4.19167250378794,-2.45388990632559,
-0.0010763688550719));
#36069=CARTESIAN_POINT('Ctrl Pts',(-4.30732749621206,-2.45404119041951,
-0.000930649193247773));
#36070=CARTESIAN_POINT('Ctrl Pts',(-4.30460347853632,-2.45429567471368,
-0.0531456272134299));
#36071=CARTESIAN_POINT('Ctrl Pts',(-4.30187946086059,-2.45277284613908,
-0.105345489901966));
#36072=CARTESIAN_POINT('Ctrl Pts',(-4.29915544318485,-2.4494254231993,-0.157428083295025));
#36073=CARTESIAN_POINT('Ctrl Pts',(-4.25691208366292,-2.39751445655014,
-0.965111431730932));
#36074=CARTESIAN_POINT('Ctrl Pts',(-4.214668724141,-1.90680675688632,-1.74459268510356));
#36075=CARTESIAN_POINT('Ctrl Pts',(-4.17242536461907,-1.20095645172772,
-2.14060087505314));
#36076=CARTESIAN_POINT('Ctrl Pts',(-4.13018200509715,-0.495106146569108,
-2.53660906500273));
#36077=CARTESIAN_POINT('Ctrl Pts',(-4.08793864557522,0.425886764084292,
-2.54914419152929));
#36078=CARTESIAN_POINT('Ctrl Pts',(-4.04569528605329,1.14225330977148,-2.17249301070089));
#36079=CARTESIAN_POINT('Ctrl Pts',(-4.00345192653137,1.85861985545867,-1.7958418298725));
#36080=CARTESIAN_POINT('Ctrl Pts',(-3.96120856700944,2.37036003617965,-1.03000434168917));
#36081=CARTESIAN_POINT('Ctrl Pts',(-3.91896520748752,2.44423356710959,-0.224032976672993));
#36082=CARTESIAN_POINT('Ctrl Pts',(-3.87672184796559,2.51810709803952,0.581938388343184));
#36083=CARTESIAN_POINT('Ctrl Pts',(-3.83447848844366,2.1541139791784,1.42804363019219));
#36084=CARTESIAN_POINT('Ctrl Pts',(-3.79223512892174,1.5181545285287,1.92864598429309));
#36085=CARTESIAN_POINT('Ctrl Pts',(-3.74999176939981,0.882195077879015,
2.42924833839399));
#36086=CARTESIAN_POINT('Ctrl Pts',(-3.70774840987788,-0.0257307045592446,
2.5843478047468));
#36087=CARTESIAN_POINT('Ctrl Pts',(-3.66550505035596,-0.791809567298263,
2.32325334700692));
#36088=CARTESIAN_POINT('Ctrl Pts',(-3.62326169083403,-1.55788843003727,
2.06215888926704));
#36089=CARTESIAN_POINT('Ctrl Pts',(-3.58101833131211,-2.18212037307705,
1.38487050743447));
#36090=CARTESIAN_POINT('Ctrl Pts',(-3.53877497179018,-2.37999376010142,
0.60008183365056));
#36091=CARTESIAN_POINT('Ctrl Pts',(-3.52829247993081,-2.42909511454254,
0.405340199051181));
#36092=CARTESIAN_POINT('Ctrl Pts',(-3.51780998807143,-2.45194297250802,
0.203979115877225));
#36093=CARTESIAN_POINT('Ctrl Pts',(-3.50732749621206,-2.45012855430742,
0.00221267815828837));
#36094=CARTESIAN_POINT('Origin',(-5.8,0.,0.));
#36095=CARTESIAN_POINT('',(-2.59167250378793,-2.44668279904974,-0.000649636572573609));
#36096=CARTESIAN_POINT('',(-2.70732749621205,-2.44676251251288,-0.000789265007911526));
#36097=CARTESIAN_POINT('',(-5.8,-2.4505,-3.00099698131059E-16));
#36098=CARTESIAN_POINT('Ctrl Pts',(-2.59167250378793,-2.44668279904974,
-0.000649636572573609));
#36099=CARTESIAN_POINT('Ctrl Pts',(-2.6148922191524,-2.44561343820275,0.447872676063153));
#36100=CARTESIAN_POINT('Ctrl Pts',(-2.63811193451688,-2.32764197931026,
0.896918504753983));
#36101=CARTESIAN_POINT('Ctrl Pts',(-2.66133164988135,-2.0962134545358,1.2768548615758));
#36102=CARTESIAN_POINT('Ctrl Pts',(-2.70357500940327,-1.67517821692753,
1.96806867986544));
#36103=CARTESIAN_POINT('Ctrl Pts',(-2.7458183689252,-0.87862160346684,2.43054324988572));
#36104=CARTESIAN_POINT('Ctrl Pts',(-2.78806172844712,-0.0695971627017047,
2.45349249759474));
#36105=CARTESIAN_POINT('Ctrl Pts',(-2.83030508796905,0.739427278063431,
2.47644174530375));
#36106=CARTESIAN_POINT('Ctrl Pts',(-2.87254844749098,1.560919546133,2.05986567070149));
#36107=CARTESIAN_POINT('Ctrl Pts',(-2.9147918070129,2.02046094368866,1.3936307873511));
#36108=CARTESIAN_POINT('Ctrl Pts',(-2.95703516653483,2.48000234124432,0.727395904000699));
#36109=CARTESIAN_POINT('Ctrl Pts',(-2.99927852605676,2.57759286828607,-0.188497788097863));
#36110=CARTESIAN_POINT('Ctrl Pts',(-3.04152188557868,2.26875284079684,-0.936605435506233));
#36111=CARTESIAN_POINT('Ctrl Pts',(-3.08376524510061,1.9599128133076,-1.6847130829146));
#36112=CARTESIAN_POINT('Ctrl Pts',(-3.12600860462254,1.24464223128742,-2.2650346856328));
#36113=CARTESIAN_POINT('Ctrl Pts',(-3.16825196414446,0.448946204655884,
-2.41307200516384));
#36114=CARTESIAN_POINT('Ctrl Pts',(-3.21049532366639,-0.346749821975649,
-2.56110932469487));
#36115=CARTESIAN_POINT('Ctrl Pts',(-3.25273868318831,-1.22287129321851,
-2.27686236103874));
#36116=CARTESIAN_POINT('Ctrl Pts',(-3.29498204271024,-1.78010068543423,
-1.68988483208406));
#36117=CARTESIAN_POINT('Ctrl Pts',(-3.3272121964028,-2.20524653454231,-1.24204223181757));
#36118=CARTESIAN_POINT('Ctrl Pts',(-3.35944235009537,-2.44476092121642,
-0.617976008401615));
#36119=CARTESIAN_POINT('Ctrl Pts',(-3.39167250378793,-2.45039822849204,
0.0022139813149212));
#36120=CARTESIAN_POINT('Ctrl Pts',(-3.50732749621206,-2.45012855430742,
0.00221267815828837));
#36121=CARTESIAN_POINT('Ctrl Pts',(-3.4755666285495,-2.44463105455957,-0.609118788930331));
#36122=CARTESIAN_POINT('Ctrl Pts',(-3.44380576088695,-2.21272709940641,
-1.22417152185401));
#36123=CARTESIAN_POINT('Ctrl Pts',(-3.4120448932244,-1.79867693109158,-1.67009874042576));
#36124=CARTESIAN_POINT('Ctrl Pts',(-3.36980153370247,-1.24797188404843,
-2.26320167498284));
#36125=CARTESIAN_POINT('Ctrl Pts',(-3.32755817418055,-0.375046958953182,
-2.55711857836172));
#36126=CARTESIAN_POINT('Ctrl Pts',(-3.28531481465862,0.422237238642569,
-2.41788838031261));
#36127=CARTESIAN_POINT('Ctrl Pts',(-3.24307145513669,1.21952143623832,-2.27865818226351));
#36128=CARTESIAN_POINT('Ctrl Pts',(-3.20082809561477,1.94116490633457,-1.70628088278641));
#36129=CARTESIAN_POINT('Ctrl Pts',(-3.15858473609284,2.25825791152587,-0.961633875260976));
#36130=CARTESIAN_POINT('Ctrl Pts',(-3.11634137657092,2.57535091671716,-0.216986867735556));
#36131=CARTESIAN_POINT('Ctrl Pts',(-3.07409801704899,2.48789345700351,0.699929847838214));
#36132=CARTESIAN_POINT('Ctrl Pts',(-3.03185465752707,2.03574678129801,1.37120514426048));
#36133=CARTESIAN_POINT('Ctrl Pts',(-2.98961129800514,1.58360010559251,2.04248044068275));
#36134=CARTESIAN_POINT('Ctrl Pts',(-2.94736793848321,0.766764213895166,
2.46811431795353));
#36135=CARTESIAN_POINT('Ctrl Pts',(-2.90512457896129,-0.0424644758308468,
2.45411191152685));
#36136=CARTESIAN_POINT('Ctrl Pts',(-2.86288121943936,-0.851693165556859,
2.44010950510017));
#36137=CARTESIAN_POINT('Ctrl Pts',(-2.82063785991743,-1.65331465331153,
1.98647081497602));
#36138=CARTESIAN_POINT('Ctrl Pts',(-2.77839450039551,-2.08196692368307,
1.29995470395946));
#36139=CARTESIAN_POINT('Ctrl Pts',(-2.75470549900102,-2.32234421245695,
0.914973933129283));
#36140=CARTESIAN_POINT('Ctrl Pts',(-2.73101649760654,-2.44543457696559,
0.456760640272405));
#36141=CARTESIAN_POINT('Ctrl Pts',(-2.70732749621205,-2.44676251251288,
-0.000789265007911525));
#36142=CARTESIAN_POINT('Origin',(-5.8,0.,0.));
#36143=CARTESIAN_POINT('',(-1.79167250378793,-2.45275230455429,-0.00175416635020159));
#36144=CARTESIAN_POINT('',(-1.90732749621205,-2.4529852431004,-0.00165255154954544));
#36145=CARTESIAN_POINT('',(-5.8,-2.4505,-3.00099698131059E-16));
#36146=CARTESIAN_POINT('Ctrl Pts',(-1.79167250378793,-2.45275230455429,
-0.00175416635020159));
#36147=CARTESIAN_POINT('Ctrl Pts',(-1.82809872868751,-2.44708780047584,
0.697443506496413));
#36148=CARTESIAN_POINT('Ctrl Pts',(-1.8645249535871,-2.13271448402931,1.40109234088029));
#36149=CARTESIAN_POINT('Ctrl Pts',(-1.90095117848668,-1.60460482446254,
1.85734002710478));
#36150=CARTESIAN_POINT('Ctrl Pts',(-1.9431945380086,-0.992157987668917,
2.38644879677171));
#36151=CARTESIAN_POINT('Ctrl Pts',(-1.98543789753053,-0.0922580856068916,
2.58282885333754));
#36152=CARTESIAN_POINT('Ctrl Pts',(-2.02768125705246,0.684939924235908,
2.35697404655791));
#36153=CARTESIAN_POINT('Ctrl Pts',(-2.06992461657438,1.46213793407869,2.13111923977828));
#36154=CARTESIAN_POINT('Ctrl Pts',(-2.11216797609631,2.11663405170226,1.48302956965323));
#36155=CARTESIAN_POINT('Ctrl Pts',(-2.15441133561823,2.35012273319099,0.70809067381542));
#36156=CARTESIAN_POINT('Ctrl Pts',(-2.19665469514016,2.58361141467973,-0.0668482220224072));
#36157=CARTESIAN_POINT('Ctrl Pts',(-2.23889805466208,2.39609266003361,-0.968636343572973));
#36158=CARTESIAN_POINT('Ctrl Pts',(-2.28114141418401,1.87303360117565,-1.58625793690777));
#36159=CARTESIAN_POINT('Ctrl Pts',(-2.32338477370594,1.34997454231769,-2.20387953024255));
#36160=CARTESIAN_POINT('Ctrl Pts',(-2.36562813322786,0.491375179247872,
-2.53733459536155));
#36161=CARTESIAN_POINT('Ctrl Pts',(-2.40787149274979,-0.311433207592666,
-2.43464136614626));
#36162=CARTESIAN_POINT('Ctrl Pts',(-2.45011485227172,-1.11424159443319,
-2.33194813693097));
#36163=CARTESIAN_POINT('Ctrl Pts',(-2.49235821179364,-1.86125900504446,
-1.79310661338139));
#36164=CARTESIAN_POINT('Ctrl Pts',(-2.53460157131557,-2.21201077947218,
-1.06370931832713));
#36165=CARTESIAN_POINT('Ctrl Pts',(-2.55362521547302,-2.36996642078062,
-0.735236518162622));
#36166=CARTESIAN_POINT('Ctrl Pts',(-2.57264885963048,-2.4475589140197,-0.368118778133049));
#36167=CARTESIAN_POINT('Ctrl Pts',(-2.59167250378793,-2.44668279904974,
-0.000649636572573609));
#36168=CARTESIAN_POINT('Ctrl Pts',(-2.70732749621205,-2.44676251251288,
-0.000789265007911525));
#36169=CARTESIAN_POINT('Ctrl Pts',(-2.68877313808461,-2.44780261510329,
-0.359164219797027));
#36170=CARTESIAN_POINT('Ctrl Pts',(-2.67021877995717,-2.37414425470941,
-0.717132201493089));
#36171=CARTESIAN_POINT('Ctrl Pts',(-2.65166442182973,-2.22363693076463,
-1.03918588605928));
#36172=CARTESIAN_POINT('Ctrl Pts',(-2.60942106230781,-1.88097161448621,
-1.77241683315251));
#36173=CARTESIAN_POINT('Ctrl Pts',(-2.56717770278588,-1.13995792894096,
-2.31948519543));
#36174=CARTESIAN_POINT('Ctrl Pts',(-2.52493434326395,-0.338334145998326,
-2.4310488509504));
#36175=CARTESIAN_POINT('Ctrl Pts',(-2.48269098374203,0.463289636944311,
-2.54261250647081));
#36176=CARTESIAN_POINT('Ctrl Pts',(-2.4404476242201,1.32552351728434,-2.21867145523413));
#36177=CARTESIAN_POINT('Ctrl Pts',(-2.39820426469818,1.85537964471098,-1.60687114221059));
#36178=CARTESIAN_POINT('Ctrl Pts',(-2.35596090517625,2.38523577213763,-0.995070829187048));
#36179=CARTESIAN_POINT('Ctrl Pts',(-2.31371754565432,2.58271414665089,-0.0954112543766505));
#36180=CARTESIAN_POINT('Ctrl Pts',(-2.2714741861324,2.35780831881423,0.682061905814828));
#36181=CARTESIAN_POINT('Ctrl Pts',(-2.22923082661047,2.13290249097757,1.45953506600631));
#36182=CARTESIAN_POINT('Ctrl Pts',(-2.18698746708854,1.48561246079097,2.11482181157887));
#36183=CARTESIAN_POINT('Ctrl Pts',(-2.14474410756662,0.710959266367213,
2.34925636222754));
#36184=CARTESIAN_POINT('Ctrl Pts',(-2.10250074804469,-0.0636939280565581,
2.58369091287621));
#36185=CARTESIAN_POINT('Ctrl Pts',(-2.06025738852277,-0.965710286717498,
2.39727326860099));
#36186=CARTESIAN_POINT('Ctrl Pts',(-2.01801402900084,-1.58396997886496,
1.87496867400264));
#36187=CARTESIAN_POINT('Ctrl Pts',(-1.98111851807124,-2.12396034627677,
1.41878585387021));
#36188=CARTESIAN_POINT('Ctrl Pts',(-1.94422300714165,-2.44749142227523,
0.706376978662933));
#36189=CARTESIAN_POINT('Ctrl Pts',(-1.90732749621205,-2.4529852431004,-0.00165255154954544));
#36190=CARTESIAN_POINT('Origin',(-5.8,0.,0.));
#36191=CARTESIAN_POINT('',(-0.991672503787933,-2.45191048624635,0.00202700265848121));
#36192=CARTESIAN_POINT('',(-1.10732749621205,-2.45164311140852,0.00208312759044971));
#36193=CARTESIAN_POINT('',(-5.8,-2.4505,-3.00099698131059E-16));
#36194=CARTESIAN_POINT('Ctrl Pts',(-0.991672503787933,-2.45191048624635,
0.00202700265848121));
#36195=CARTESIAN_POINT('Ctrl Pts',(-0.999061878700698,-2.45317470252284,
0.143994484330699));
#36196=CARTESIAN_POINT('Ctrl Pts',(-1.00645125361346,-2.44190225774454,
0.28576134120172));
#36197=CARTESIAN_POINT('Ctrl Pts',(-1.01384062852623,-2.41737842412646,
0.425196841749238));
#36198=CARTESIAN_POINT('Ctrl Pts',(-1.05608398804815,-2.27718129884662,
1.22231757919796));
#36199=CARTESIAN_POINT('Ctrl Pts',(-1.09832734757008,-1.7039093940212,1.94324618025634));
#36200=CARTESIAN_POINT('Ctrl Pts',(-1.14057070709201,-0.958872451732294,
2.25942616043133));
#36201=CARTESIAN_POINT('Ctrl Pts',(-1.18281406661393,-0.213835509443387,
2.57560614060633));
#36202=CARTESIAN_POINT('Ctrl Pts',(-1.22505742613586,0.702966470309022,
2.48703749989794));
#36203=CARTESIAN_POINT('Ctrl Pts',(-1.26730078565778,1.37368755904065,2.03407355411655));
#36204=CARTESIAN_POINT('Ctrl Pts',(-1.30954414517971,2.04440864777229,1.58110960833516));
#36205=CARTESIAN_POINT('Ctrl Pts',(-1.35178750470164,2.46904884548314,0.763750357480772));
#36206=CARTESIAN_POINT('Ctrl Pts',(-1.39403086422356,2.45405941828723,-0.0454617002379226));
#36207=CARTESIAN_POINT('Ctrl Pts',(-1.43627422374549,2.43906999109132,-0.854673757956606));
#36208=CARTESIAN_POINT('Ctrl Pts',(-1.47851758326741,1.98445093898863,-1.65573862253959));
#36209=CARTESIAN_POINT('Ctrl Pts',(-1.52076094278934,1.29741150126341,-2.08355193165779));
#36210=CARTESIAN_POINT('Ctrl Pts',(-1.56300430231127,0.610372063538196,
-2.51136524077598));
#36211=CARTESIAN_POINT('Ctrl Pts',(-1.60524766183319,-0.309087759809568,
-2.56592699442941));
#36212=CARTESIAN_POINT('Ctrl Pts',(-1.64749102135512,-1.04189960834166,
-2.22236703125869));
#36213=CARTESIAN_POINT('Ctrl Pts',(-1.68973438087704,-1.77471145687375,
-1.87880706808797));
#36214=CARTESIAN_POINT('Ctrl Pts',(-1.73197774039897,-2.32087533059018,
-1.13712538809311));
#36215=CARTESIAN_POINT('Ctrl Pts',(-1.7742210999209,-2.43146038168579,-0.335365806711661));
#36216=CARTESIAN_POINT('Ctrl Pts',(-1.78003823454324,-2.44668852965324,
-0.224959260631187));
#36217=CARTESIAN_POINT('Ctrl Pts',(-1.78585536916559,-2.45365690509645,
-0.113413472297838));
#36218=CARTESIAN_POINT('Ctrl Pts',(-1.79167250378793,-2.45275230455429,
-0.00175416635020159));
#36219=CARTESIAN_POINT('Ctrl Pts',(-1.90732749621205,-2.4529852431004,-0.00165255154954544));
#36220=CARTESIAN_POINT('Ctrl Pts',(-1.90197964761972,-2.45378154924243,
-0.104278443726542));
#36221=CARTESIAN_POINT('Ctrl Pts',(-1.89663179902739,-2.44789612195828,
-0.206812329022707));
#36222=CARTESIAN_POINT('Ctrl Pts',(-1.89128395043506,-2.43501963539058,
-0.308460610226293));
#36223=CARTESIAN_POINT('Ctrl Pts',(-1.84904059091313,-2.33330657413478,
-1.11139375493544));
#36224=CARTESIAN_POINT('Ctrl Pts',(-1.80679723139121,-1.79537742598919,
-1.85906849943227));
#36225=CARTESIAN_POINT('Ctrl Pts',(-1.76455387186928,-1.06640896295346,
-2.21071042645277));
#36226=CARTESIAN_POINT('Ctrl Pts',(-1.72231051234736,-0.337440499917736,
-2.56235235347326));
#36227=CARTESIAN_POINT('Ctrl Pts',(-1.68006715282543,0.582567278008129,
-2.51796146301742));
#36228=CARTESIAN_POINT('Ctrl Pts',(-1.6378237933035,1.27429461852628,-2.09777051925233));
#36229=CARTESIAN_POINT('Ctrl Pts',(-1.59558043378158,1.96602195904445,-1.67757957548724));
#36230=CARTESIAN_POINT('Ctrl Pts',(-1.55333707425965,2.42946886215489,-0.881588578412895));
#36231=CARTESIAN_POINT('Ctrl Pts',(-1.51109371473772,2.45340568023822,-0.0725926363383835));
#36232=CARTESIAN_POINT('Ctrl Pts',(-1.4688503552158,2.47734249832155,0.736403305736105));
#36233=CARTESIAN_POINT('Ctrl Pts',(-1.42660699569387,2.06176923137779,1.55840419281076));
#36234=CARTESIAN_POINT('Ctrl Pts',(-1.38436363617195,1.39609611498331,2.01875827328353));
#36235=CARTESIAN_POINT('Ctrl Pts',(-1.34212027665002,0.73042299858883,2.47911235375631));
#36236=CARTESIAN_POINT('Ctrl Pts',(-1.2998769171281,-0.185349967256377,
2.57781962762719));
#36237=CARTESIAN_POINT('Ctrl Pts',(-1.25763355760617,-0.933834445849563,
2.26989378192159));
#36238=CARTESIAN_POINT('Ctrl Pts',(-1.21539019808424,-1.68231892444275,
1.96196793621599));
#36239=CARTESIAN_POINT('Ctrl Pts',(-1.17314683856232,-2.26351491578391,
1.24740897093391));
#36240=CARTESIAN_POINT('Ctrl Pts',(-1.13090347904039,-2.41252280639993,
0.451893154076523));
#36241=CARTESIAN_POINT('Ctrl Pts',(-1.12304481809761,-2.44024319851368,
0.303900921686603));
#36242=CARTESIAN_POINT('Ctrl Pts',(-1.11518615715483,-2.45300629731437,
0.153106910689909));
#36243=CARTESIAN_POINT('Ctrl Pts',(-1.10732749621205,-2.45164311140852,
0.00208312759044971));
#36244=CARTESIAN_POINT('Origin',(-5.8,0.,0.));
#36245=CARTESIAN_POINT('',(-0.191672503787931,-2.44602797108083,-0.000435857851394948));
#36246=CARTESIAN_POINT('',(-0.307327496212056,-2.44646461313235,-7.12799915801969E-5));
#36247=CARTESIAN_POINT('',(-5.8,-2.4505,-3.00099698131059E-16));
#36248=CARTESIAN_POINT('Ctrl Pts',(-0.191672503787931,-2.44601738174545,
-0.0004368899209653));
#36249=CARTESIAN_POINT('Ctrl Pts',(-0.212268388235807,-2.44653079006204,
0.397767213870827));
#36250=CARTESIAN_POINT('Ctrl Pts',(-0.232864272683682,-2.35532542844842,
0.796028585207236));
#36251=CARTESIAN_POINT('Ctrl Pts',(-0.253460157131558,-2.17142533223093,
1.14526153389913));
#36252=CARTESIAN_POINT('Ctrl Pts',(-0.295703516653484,-1.79423551548414,
1.86155866820433));
#36253=CARTESIAN_POINT('Ctrl Pts',(-0.337946876175409,-1.02709377158744,
2.37160106779288));
#36254=CARTESIAN_POINT('Ctrl Pts',(-0.380190235697335,-0.220869436790385,
2.44430655566939));
#36255=CARTESIAN_POINT('Ctrl Pts',(-0.422433595219262,0.585354898006676,
2.5170120435459));
#36256=CARTESIAN_POINT('Ctrl Pts',(-0.464676954741189,1.43066182370407,
2.15238061971035));
#36257=CARTESIAN_POINT('Ctrl Pts',(-0.506920314263115,1.93040321642611,
1.51590454149075));
#36258=CARTESIAN_POINT('Ctrl Pts',(-0.549163673785041,2.43014460914813,
0.879428463271162));
#36259=CARTESIAN_POINT('Ctrl Pts',(-0.591407033306968,2.58432046889479,
-0.0288922693324942));
#36260=CARTESIAN_POINT('Ctrl Pts',(-0.633650392828894,2.32233492104033,
-0.794700919203336));
#36261=CARTESIAN_POINT('Ctrl Pts',(-0.67589375235082,2.06034937318587,-1.56050956907417));
#36262=CARTESIAN_POINT('Ctrl Pts',(-0.718137111872745,1.38220241773032,
-2.18380613621221));
#36263=CARTESIAN_POINT('Ctrl Pts',(-0.760380471394671,0.597149656144279,
-2.38069557645246));
#36264=CARTESIAN_POINT('Ctrl Pts',(-0.802623830916597,-0.187903105441769,
-2.57758501669272));
#36265=CARTESIAN_POINT('Ctrl Pts',(-0.844867190438523,-1.07986167315829,
-2.34806733003518));
#36266=CARTESIAN_POINT('Ctrl Pts',(-0.88711054996045,-1.67227978414943,
-1.79665204978687));
#36267=CARTESIAN_POINT('Ctrl Pts',(-0.921964534569611,-2.16106978466905,
-1.3416925032798));
#36268=CARTESIAN_POINT('Ctrl Pts',(-0.956818519178772,-2.44594746837766,
-0.667601007778074));
#36269=CARTESIAN_POINT('Ctrl Pts',(-0.991672503787933,-2.45191048624635,
0.00202700265848121));
#36270=CARTESIAN_POINT('Ctrl Pts',(-1.10732749621205,-2.45164311140852,
0.00208312759044971));
#36271=CARTESIAN_POINT('Ctrl Pts',(-1.07294279763291,-2.4456786428023,-0.658704670479551));
#36272=CARTESIAN_POINT('Ctrl Pts',(-1.03855809905376,-2.16928017252217,
-1.32389123230908));
#36273=CARTESIAN_POINT('Ctrl Pts',(-1.00417340047461,-1.6920551196339,-1.77803867535403));
#36274=CARTESIAN_POINT('Ctrl Pts',(-0.961930040952687,-1.105759752361,-2.33598201949449));
#36275=CARTESIAN_POINT('Ctrl Pts',(-0.91968668143076,-0.216349227924323,
-2.57539603934272));
#36276=CARTESIAN_POINT('Ctrl Pts',(-0.877443321908835,0.5708124140107,-2.38717728466095));
#36277=CARTESIAN_POINT('Ctrl Pts',(-0.835199962386909,1.35797405594572,
-2.19895852997917));
#36278=CARTESIAN_POINT('Ctrl Pts',(-0.792956602864983,2.04288681537911,
-1.5831070007674));
#36279=CARTESIAN_POINT('Ctrl Pts',(-0.750713243343057,2.31336229750905,
-0.820283519894993));
#36280=CARTESIAN_POINT('Ctrl Pts',(-0.708469883821131,2.583837779639,-0.0574600390225732));
#36281=CARTESIAN_POINT('Ctrl Pts',(-0.666226524299204,2.43987598446552,
0.852335393510467));
#36282=CARTESIAN_POINT('Ctrl Pts',(-0.623983164777278,1.94712925542381,
1.49437790025489));
#36283=CARTESIAN_POINT('Ctrl Pts',(-0.581739805255351,1.4543825263821,2.13642040699932));
#36284=CARTESIAN_POINT('Ctrl Pts',(-0.539496445733424,0.61285086347215,
2.5107099879551));
#36285=CARTESIAN_POINT('Ctrl Pts',(-0.497253086211498,-0.193985232491749,
2.44676681777884));
#36286=CARTESIAN_POINT('Ctrl Pts',(-0.455009726689572,-1.00082132845564,
2.38282364760258));
#36287=CARTESIAN_POINT('Ctrl Pts',(-0.412766367167645,-1.77296185747349,
1.88064772629427));
#36288=CARTESIAN_POINT('Ctrl Pts',(-0.37052300764572,-2.15834482944737,
1.16890388041718));
#36289=CARTESIAN_POINT('Ctrl Pts',(-0.349457837167832,-2.3505207855214,
0.813984062967378));
#36290=CARTESIAN_POINT('Ctrl Pts',(-0.328392666689944,-2.4465240289526,
0.406952230065944));
#36291=CARTESIAN_POINT('Ctrl Pts',(-0.307327496212056,-2.44646461313235,
-7.12799915801969E-5));
#36292=CARTESIAN_POINT('Origin',(-13.1285451186048,0.,0.));
#36293=CARTESIAN_POINT('',(-0.72854511860476,-1.99589816055495,0.00165001573264543));
#36294=CARTESIAN_POINT('',(-0.570454881395212,-1.99146512427903,-5.80231641911233E-5));
#36295=CARTESIAN_POINT('',(-13.1285451186048,-1.99475,-1.92374832954336E-13));
#36296=CARTESIAN_POINT('',(-9.0205620750794E-16,-1.69189910824764,1.06268379792867));
#36297=CARTESIAN_POINT('Ctrl Pts',(-0.72854511860476,-1.99589816055495,
0.00165001573264557));
#36298=CARTESIAN_POINT('Ctrl Pts',(-0.6936911339956,-1.99104415937413,-0.543438935019565));
#36299=CARTESIAN_POINT('Ctrl Pts',(-0.616593789864514,-1.47808926389438,
-1.75721787381682));
#36300=CARTESIAN_POINT('Ctrl Pts',(-0.497253086211501,0.573113500662185,
-2.2850308579914));
#36301=CARTESIAN_POINT('Ctrl Pts',(-0.370523007645721,2.22918406511225,
-0.762907829264197));
#36302=CARTESIAN_POINT('Ctrl Pts',(-0.243792929079945,1.85267849943624,
1.45525921586262));
#36303=CARTESIAN_POINT('Ctrl Pts',(-0.120285259864702,-0.159116251582435,
2.32306659118204));
#36304=CARTESIAN_POINT('Ctrl Pts',(-0.039020950171389,-1.36508286981671,
1.57661195366552));
#36305=CARTESIAN_POINT('Ctrl Pts',(-6.86842076269567E-16,-1.69189910824764,
1.06268379792867));
#36306=CARTESIAN_POINT('',(0.,0.458732584425967,1.94128616604711));
#36307=CARTESIAN_POINT('Origin',(0.,0.,0.));
#36308=CARTESIAN_POINT('Ctrl Pts',(-0.570454881395212,-1.99146512427903,
-5.80231641910539E-5));
#36309=CARTESIAN_POINT('Ctrl Pts',(-0.549276692351179,-1.99141649926868,
-0.333159919088959));
#36310=CARTESIAN_POINT('Ctrl Pts',(-0.48585514378522,-1.75457861196001,
-1.3306674833886));
#36311=CARTESIAN_POINT('Ctrl Pts',(-0.380190235697333,-0.180414554165581,
-2.34831227349832));
#36312=CARTESIAN_POINT('Ctrl Pts',(-0.253460157131555,1.87363647225322,
-1.43076438289222));
#36313=CARTESIAN_POINT('Ctrl Pts',(-0.126730078565778,2.21660082027165,
0.796119646106798));
#36314=CARTESIAN_POINT('Ctrl Pts',(-0.0422433595219261,1.10280973225228,
1.78908852524606));
#36315=CARTESIAN_POINT('Ctrl Pts',(0.,0.458732584425967,1.94128616604711));
#36316=CARTESIAN_POINT('Origin',(-13.1285451186048,0.,0.));
#36317=CARTESIAN_POINT('',(-1.52854511860476,-1.99658341542937,-0.00142792219028397));
#36318=CARTESIAN_POINT('',(-1.37045488139521,-1.99568051274521,0.00169570241191928));
#36319=CARTESIAN_POINT('',(-13.1285451186048,-1.99475,-1.92374832954336E-13));
#36320=CARTESIAN_POINT('Ctrl Pts',(-1.52854511860476,-1.99658341542937,
-0.00142792219028407));
#36321=CARTESIAN_POINT('Ctrl Pts',(-1.52272798398241,-1.99731977614411,
-0.0923205565665347));
#36322=CARTESIAN_POINT('Ctrl Pts',(-1.47466748983814,-1.95045522889083,
-0.842501557985075));
#36323=CARTESIAN_POINT('Ctrl Pts',(-1.38436363617195,-1.00005929055416,
-2.13312382380668));
#36324=CARTESIAN_POINT('Ctrl Pts',(-1.25763355760617,1.24531000055737,-1.9998811491278));
#36325=CARTESIAN_POINT('Ctrl Pts',(-1.13090347904039,2.35551365799275,-0.0436385799048972));
#36326=CARTESIAN_POINT('Ctrl Pts',(-1.00417340047461,1.31851994113852,1.95239573836704));
#36327=CARTESIAN_POINT('Ctrl Pts',(-0.877443321908835,-0.920358755998121,
2.16868502143541));
#36328=CARTESIAN_POINT('Ctrl Pts',(-0.785567227952218,-1.93529438584288,
0.892334100294173));
#36329=CARTESIAN_POINT('Ctrl Pts',(-0.735934493517526,-1.99692725478777,
0.117214036979607));
#36330=CARTESIAN_POINT('Ctrl Pts',(-0.72854511860476,-1.99589816055495,
0.00165001573264557));
#36331=CARTESIAN_POINT('Ctrl Pts',(-1.37045488139521,-1.99568051274521,
0.0016957024119192));
#36332=CARTESIAN_POINT('Ctrl Pts',(-1.33607018281607,-1.99082533063853,
-0.536197160350763));
#36333=CARTESIAN_POINT('Ctrl Pts',(-1.259442124715,-1.48941647468376,-1.74289860347138));
#36334=CARTESIAN_POINT('Ctrl Pts',(-1.14057070709201,0.54788370586334,-2.29130478089007));
#36335=CARTESIAN_POINT('Ctrl Pts',(-1.01384062852623,2.22047671979483,-0.787362926702919));
#36336=CARTESIAN_POINT('Ctrl Pts',(-0.887110549960448,1.86891443749856,
1.43440541328318));
#36337=CARTESIAN_POINT('Ctrl Pts',(-0.760380471394668,-0.186150183504844,
2.34844027344827));
#36338=CARTESIAN_POINT('Ctrl Pts',(-0.654828581872924,-1.75664923517798,
1.3270370721541));
#36339=CARTESIAN_POINT('Ctrl Pts',(-0.591520051873105,-1.99151348979935,
0.331266256243046));
#36340=CARTESIAN_POINT('Ctrl Pts',(-0.570454881395212,-1.99146512427903,
-5.80231641910539E-5));
#36341=CARTESIAN_POINT('Origin',(-13.1285451186048,0.,0.));
#36342=CARTESIAN_POINT('',(-2.32854511860476,-1.99164273144438,-0.000528815569653849));
#36343=CARTESIAN_POINT('',(-2.17045488139521,-1.99677303149338,-0.00134520595961224));
#36344=CARTESIAN_POINT('',(-13.1285451186048,-1.99475,-1.92374832954336E-13));
#36345=CARTESIAN_POINT('Ctrl Pts',(-2.32854511860476,-1.99164273144438,
-0.000528815569653777));
#36346=CARTESIAN_POINT('Ctrl Pts',(-2.3095214744473,-1.99235590440349,-0.299655144942299));
#36347=CARTESIAN_POINT('Ctrl Pts',(-2.24825447076793,-1.7889392995189,-1.26209160177339));
#36348=CARTESIAN_POINT('Ctrl Pts',(-2.14474410756662,-0.298926929475087,
-2.33687315863848));
#36349=CARTESIAN_POINT('Ctrl Pts',(-2.01801402900084,1.79781791380199,-1.52255833577031));
#36350=CARTESIAN_POINT('Ctrl Pts',(-1.89128395043506,2.25574858406966,0.679655729273182));
#36351=CARTESIAN_POINT('Ctrl Pts',(-1.76455387186929,0.657434610640146,
2.26232482066099));
#36352=CARTESIAN_POINT('Ctrl Pts',(-1.64364092792585,-1.43929446373414,
1.80476751535916));
#36353=CARTESIAN_POINT('Ctrl Pts',(-1.56497134350434,-1.991972409712,0.567731252635601));
#36354=CARTESIAN_POINT('Ctrl Pts',(-1.52854511860476,-1.99658341542937,
-0.00142792219028407));
#36355=CARTESIAN_POINT('Ctrl Pts',(-2.17045488139521,-1.99677303149338,
-0.0013452059596123));
#36356=CARTESIAN_POINT('Ctrl Pts',(-2.16510703280289,-1.99742123866611,
-0.0848844830132346));
#36357=CARTESIAN_POINT('Ctrl Pts',(-2.11751582468863,-1.95478691364556,
-0.827644996443922));
#36358=CARTESIAN_POINT('Ctrl Pts',(-2.02768125705245,-1.02358496316198,
-2.12193474222715));
#36359=CARTESIAN_POINT('Ctrl Pts',(-1.90095117848668,1.22312246187489,-2.01352985089457));
#36360=CARTESIAN_POINT('Ctrl Pts',(-1.77422109992089,2.35488419618976,-0.0696779332279315));
#36361=CARTESIAN_POINT('Ctrl Pts',(-1.64749102135512,1.34003240157303,1.9376915050404));
#36362=CARTESIAN_POINT('Ctrl Pts',(-1.52076094278934,-0.896333389432558,
2.17873986401275));
#36363=CARTESIAN_POINT('Ctrl Pts',(-1.42841556280271,-1.93055379041261,
0.907204150401554));
#36364=CARTESIAN_POINT('Ctrl Pts',(-1.37831354233799,-1.99679016999301,
0.124631711935621));
#36365=CARTESIAN_POINT('Ctrl Pts',(-1.37045488139521,-1.99568051274521,
0.0016957024119192));
#36366=CARTESIAN_POINT('Origin',(-13.1285451186048,0.,0.));
#36367=CARTESIAN_POINT('',(-3.12854511860476,-1.99466715620669,0.00180221963998484));
#36368=CARTESIAN_POINT('',(-2.97045488139521,-1.99170761960215,-0.000642475566254852));
#36369=CARTESIAN_POINT('',(-13.1285451186048,-1.99475,-1.92374832954336E-13));
#36370=CARTESIAN_POINT('Ctrl Pts',(-3.12854511860476,-1.99466715620669,
0.00180221963998481));
#36371=CARTESIAN_POINT('Ctrl Pts',(-3.0963149649122,-1.99007828916401,-0.503043314735463));
#36372=CARTESIAN_POINT('Ctrl Pts',(-3.02184145169771,-1.53956787264023,
-1.67686981490333));
#36373=CARTESIAN_POINT('Ctrl Pts',(-2.90512457896129,0.430917811620456,
-2.31616994743447));
#36374=CARTESIAN_POINT('Ctrl Pts',(-2.77839450039551,2.1776462264151,-0.898994044122268));
#36375=CARTESIAN_POINT('Ctrl Pts',(-2.65166442182973,1.93932502198757,1.33766656674925));
#36376=CARTESIAN_POINT('Ctrl Pts',(-2.52493434326395,-0.066802341895476,
2.35496727045807));
#36377=CARTESIAN_POINT('Ctrl Pts',(-2.41722790885563,-1.72003362343411,
1.39511405581719));
#36378=CARTESIAN_POINT('Ctrl Pts',(-2.35176483396923,-1.99077225295041,
0.36457621733391));
#36379=CARTESIAN_POINT('Ctrl Pts',(-2.32854511860476,-1.99164273144438,
-0.000528815569653777));
#36380=CARTESIAN_POINT('Ctrl Pts',(-2.97045488139521,-1.99170761960215,
-0.000642475566254921));
#36381=CARTESIAN_POINT('Ctrl Pts',(-2.95190052326778,-1.99255428136185,
-0.292365977327294));
#36382=CARTESIAN_POINT('Ctrl Pts',(-2.89110280561841,-1.79608386950908,
-1.24718110513933));
#36383=CARTESIAN_POINT('Ctrl Pts',(-2.78806172844712,-0.324747614573964,
-2.33342489664845));
#36384=CARTESIAN_POINT('Ctrl Pts',(-2.66133164988135,1.78087291120639,-1.54234379652064));
#36385=CARTESIAN_POINT('Ctrl Pts',(-2.53460157131557,2.26312549748712,0.654672245331693));
#36386=CARTESIAN_POINT('Ctrl Pts',(-2.40787149274979,0.682409168923879,
2.25491697383304));
#36387=CARTESIAN_POINT('Ctrl Pts',(-2.28648926277634,-1.4274081023495,1.81888589547668));
#36388=CARTESIAN_POINT('Ctrl Pts',(-2.20735039232481,-1.99230096493927,
0.575003255738612));
#36389=CARTESIAN_POINT('Ctrl Pts',(-2.17045488139521,-1.99677303149338,
-0.0013452059596123));
#36390=CARTESIAN_POINT('Origin',(-13.1285451186048,0.,0.));
#36391=CARTESIAN_POINT('',(-3.92854511860476,-1.9975094432332,-0.000876183135553181));
#36392=CARTESIAN_POINT('',(-3.77045488139522,-1.99444763668832,0.00180115884744814));
#36393=CARTESIAN_POINT('',(-13.1285451186048,-1.99475,-1.92374832954336E-13));
#36394=CARTESIAN_POINT('Ctrl Pts',(-3.92854511860476,-1.9975094432332,-0.000876183135553477));
#36395=CARTESIAN_POINT('Ctrl Pts',(-3.92535181489901,-1.99778430699875,
-0.0507107092389343));
#36396=CARTESIAN_POINT('Ctrl Pts',(-3.87991515167134,-1.97353675729167,
-0.759520997005793));
#36397=CARTESIAN_POINT('Ctrl Pts',(-3.79223512892175,-1.12994078260249,
-2.06726079904157));
#36398=CARTESIAN_POINT('Ctrl Pts',(-3.66550505035595,1.11937349904418,-2.07300177355078));
#36399=CARTESIAN_POINT('Ctrl Pts',(-3.53877497179019,2.34831453822241,-0.189082555904491));
#36400=CARTESIAN_POINT('Ctrl Pts',(-3.4120448932244,1.43663198605998,1.86719627250164));
#36401=CARTESIAN_POINT('Ctrl Pts',(-3.28531481465863,-0.784623143241175,
2.22141844480153));
#36402=CARTESIAN_POINT('Ctrl Pts',(-3.19081488978541,-1.90763475622866,
0.9755918462161));
#36403=CARTESIAN_POINT('Ctrl Pts',(-3.13855832443412,-1.99609281711604,
0.158646716751444));
#36404=CARTESIAN_POINT('Ctrl Pts',(-3.12854511860476,-1.99466715620669,
0.00180221963998481));
#36405=CARTESIAN_POINT('Ctrl Pts',(-3.77045488139522,-1.99444763668832,
0.00180115884744803));
#36406=CARTESIAN_POINT('Ctrl Pts',(-3.73869401373267,-1.98997257542647,
-0.495833382664432));
#36407=CARTESIAN_POINT('Ctrl Pts',(-3.66468978654819,-1.55012106057463,
-1.6624019998815));
#36408=CARTESIAN_POINT('Ctrl Pts',(-3.5484421998418,0.405281400923077,-2.3207929105089));
#36409=CARTESIAN_POINT('Ctrl Pts',(-3.42171212127601,2.16757274388305,-0.923017413918032));
#36410=CARTESIAN_POINT('Ctrl Pts',(-3.29498204271024,1.95399702329888,1.3161414741343));
#36411=CARTESIAN_POINT('Ctrl Pts',(-3.16825196414445,-0.0407592243607493,
2.35556180878339));
#36412=CARTESIAN_POINT('Ctrl Pts',(-3.06007624370612,-1.71175158280605,
1.40994496059256));
#36413=CARTESIAN_POINT('Ctrl Pts',(-2.9941438827897,-1.99062665676483,0.371811176161177));
#36414=CARTESIAN_POINT('Ctrl Pts',(-2.97045488139521,-1.99170761960215,
-0.000642475566254921));
#36415=CARTESIAN_POINT('Origin',(-13.1285451186048,0.,0.));
#36416=CARTESIAN_POINT('',(-4.72854511860476,-1.99216358252544,-0.00112138763685431));
#36417=CARTESIAN_POINT('',(-4.57045488139521,-1.99763259114031,-0.000757564774075681));
#36418=CARTESIAN_POINT('',(-13.1285451186048,-1.99475,-1.92374832954336E-13));
#36419=CARTESIAN_POINT('Ctrl Pts',(-4.72854511860476,-1.99216358252544,
-0.00112138763685429));
#36420=CARTESIAN_POINT('Ctrl Pts',(-4.71214530536391,-1.99348757518324,
-0.258822092703375));
#36421=CARTESIAN_POINT('Ctrl Pts',(-4.65350213260112,-1.82748356051783,
-1.17867969093914));
#36422=CARTESIAN_POINT('Ctrl Pts',(-4.55261560031641,-0.442735343327605,
-2.31394010277285));
#36423=CARTESIAN_POINT('Ctrl Pts',(-4.42588552175063,1.70031488024139,-1.63072459093592));
#36424=CARTESIAN_POINT('Ctrl Pts',(-4.29915544318485,2.29343042248776,0.538990056177979));
#36425=CARTESIAN_POINT('Ctrl Pts',(-4.17242536461907,0.795952397437793,
2.21738430689477));
#36426=CARTESIAN_POINT('Ctrl Pts',(-4.04888858975905,-1.37106665451409,
1.88314514530358));
#36427=CARTESIAN_POINT('Ctrl Pts',(-3.96759517442094,-1.99414820785581,
0.608536890354887));
#36428=CARTESIAN_POINT('Ctrl Pts',(-3.92854511860476,-1.9975094432332,-0.000876183135553477));
#36429=CARTESIAN_POINT('Ctrl Pts',(-4.57045488139521,-1.99763259114031,
-0.000757564774075889));
#36430=CARTESIAN_POINT('Ctrl Pts',(-4.56773086371948,-1.99783974582131,
-0.0432614731215861));
#36431=CARTESIAN_POINT('Ctrl Pts',(-4.52276348652182,-1.97737659900053,
-0.744701853234392));
#36432=CARTESIAN_POINT('Ctrl Pts',(-4.43555274980225,-1.15272948149133,
-2.05464047695385));
#36433=CARTESIAN_POINT('Ctrl Pts',(-4.30882267123646,1.09638368952585,-2.08525191580977));
#36434=CARTESIAN_POINT('Ctrl Pts',(-4.18209259267069,2.34608015003573,-0.215036454205511));
#36435=CARTESIAN_POINT('Ctrl Pts',(-4.0553625141049,1.45718979233537,1.85119708733083));
#36436=CARTESIAN_POINT('Ctrl Pts',(-3.92863243553913,-0.760012763696535,
2.22995814895977));
#36437=CARTESIAN_POINT('Ctrl Pts',(-3.8336632246359,-1.90237578262565,0.990500269268093));
#36438=CARTESIAN_POINT('Ctrl Pts',(-3.78093737325459,-1.99592460494202,
0.166042579635038));
#36439=CARTESIAN_POINT('Ctrl Pts',(-3.77045488139522,-1.99444763668832,
0.00180115884744803));
#36440=CARTESIAN_POINT('Origin',(-13.1285451186048,0.,0.));
#36441=CARTESIAN_POINT('',(-5.52854511860476,-1.99348645498109,0.0016885444496981));
#36442=CARTESIAN_POINT('',(-5.37045488139522,-1.99229499213755,-0.00121350091589825));
#36443=CARTESIAN_POINT('',(-13.1285451186048,-1.99475,-1.92374832954336E-13));
#36444=CARTESIAN_POINT('Ctrl Pts',(-5.52854511860476,-1.99348645498109,
0.00168854444969823));
#36445=CARTESIAN_POINT('Ctrl Pts',(-5.49893879582879,-1.98972409259997,
-0.462757055610613));
#36446=CARTESIAN_POINT('Ctrl Pts',(-5.42708911353091,-1.59690446533444,
-1.59562792885432));
#36447=CARTESIAN_POINT('Ctrl Pts',(-5.31299607171107,0.286994225274642,
-2.33836859757207));
#36448=CARTESIAN_POINT('Ctrl Pts',(-5.18626599314531,2.11794332300315,-1.03181852280261));
#36449=CARTESIAN_POINT('Ctrl Pts',(-5.05953591457952,2.01826542478903,1.21529340430752));
#36450=CARTESIAN_POINT('Ctrl Pts',(-4.93280583601374,0.0788226604640474,
2.35459558558354));
#36451=CARTESIAN_POINT('Ctrl Pts',(-4.82247557068882,-1.67219508841024,
1.47786799290997));
#36452=CARTESIAN_POINT('Ctrl Pts',(-4.75438866488583,-1.99007717672159,
0.404974706278286));
#36453=CARTESIAN_POINT('Ctrl Pts',(-4.72854511860476,-1.99216358252544,
-0.00112138763685429));
#36454=CARTESIAN_POINT('Ctrl Pts',(-5.37045488139522,-1.99229499213755,
-0.00121350091589837));
#36455=CARTESIAN_POINT('Ctrl Pts',(-5.35452435418437,-1.99369239809736,
-0.251498549257047));
#36456=CARTESIAN_POINT('Ctrl Pts',(-5.2963504674516,-1.83402193695601,-1.16375266509536));
#36457=CARTESIAN_POINT('Ctrl Pts',(-5.19593322119692,-0.468293640578219,
-2.30890316237654));
#36458=CARTESIAN_POINT('Ctrl Pts',(-5.06920314263113,1.68217981160309,-1.64942530248376));
#36459=CARTESIAN_POINT('Ctrl Pts',(-4.94247306406536,2.29924973922467,0.513598465451003));
#36460=CARTESIAN_POINT('Ctrl Pts',(-4.81574298549957,0.820421458075195,
2.20844773045863));
#36461=CARTESIAN_POINT('Ctrl Pts',(-4.69173692460954,-1.3584062128533,1.89701129862388));
#36462=CARTESIAN_POINT('Ctrl Pts',(-4.60997422324141,-1.99462724476305,
0.61587811228097));
#36463=CARTESIAN_POINT('Ctrl Pts',(-4.57045488139521,-1.99763259114031,
-0.000757564774075889));
#36464=CARTESIAN_POINT('Origin',(-13.1285451186048,0.,0.));
#36465=CARTESIAN_POINT('',(-6.32854511860476,-1.9979722269169,-0.000164116242219921));
#36466=CARTESIAN_POINT('',(-6.17045488139522,-1.99329205388752,0.00164168227339369));
#36467=CARTESIAN_POINT('',(-13.1285451186048,-1.99475,-1.92374832954336E-13));
#36468=CARTESIAN_POINT('Ctrl Pts',(-6.32854511860477,-1.9979722269169,-0.000164116242220302));
#36469=CARTESIAN_POINT('Ctrl Pts',(-6.32797564581561,-1.99798275077873,
-0.00904578607702301));
#36470=CARTESIAN_POINT('Ctrl Pts',(-6.28516281350453,-1.99391352194935,
-0.676757756073187));
#36471=CARTESIAN_POINT('Ctrl Pts',(-6.20010662167154,-1.25550409505514,
-1.9935001506777));
#36472=CARTESIAN_POINT('Ctrl Pts',(-6.07337654310573,0.989158387733211,
-2.13819995964578));
#36473=CARTESIAN_POINT('Ctrl Pts',(-5.94664646453999,2.33214618174238,-0.333807684807691));
#36474=CARTESIAN_POINT('Ctrl Pts',(-5.81991638597417,1.54924877001712,1.77486946901812));
#36475=CARTESIAN_POINT('Ctrl Pts',(-5.69318630740843,-0.645877886154986,
2.26565115135322));
#36476=CARTESIAN_POINT('Ctrl Pts',(-5.59606255161859,-1.87697369462381,
1.05898945087646));
#36477=CARTESIAN_POINT('Ctrl Pts',(-5.54118215535072,-1.9950923657192,0.199930526707089));
#36478=CARTESIAN_POINT('Ctrl Pts',(-5.52854511860476,-1.99348645498109,
0.00168854444969823));
#36479=CARTESIAN_POINT('Ctrl Pts',(-6.17045488139522,-1.99329205388752,
0.00164168227339381));
#36480=CARTESIAN_POINT('Ctrl Pts',(-6.14131784464926,-1.98971745724335,
-0.455554751072749));
#36481=CARTESIAN_POINT('Ctrl Pts',(-6.06993744838138,-1.60673514178807,
-1.58101374092423));
#36482=CARTESIAN_POINT('Ctrl Pts',(-5.95631369259159,0.261121169457012,
-2.34139883016539));
#36483=CARTESIAN_POINT('Ctrl Pts',(-5.8295836140258,2.10640484398777,-1.0551736256481));
#36484=CARTESIAN_POINT('Ctrl Pts',(-5.70285353546004,2.03157950898151,1.19290294899666));
#36485=CARTESIAN_POINT('Ctrl Pts',(-5.57612345689424,0.104852755347087,
2.35357996395588));
#36486=CARTESIAN_POINT('Ctrl Pts',(-5.46532390553932,-1.66324055776191,
1.49262058419748));
#36487=CARTESIAN_POINT('Ctrl Pts',(-5.3967677137063,-1.98998686333524,0.412188291743562));
#36488=CARTESIAN_POINT('Ctrl Pts',(-5.37045488139522,-1.99229499213755,
-0.00121350091589837));
#36489=CARTESIAN_POINT('Origin',(-13.1285451186048,0.,0.));
#36490=CARTESIAN_POINT('',(-7.12854511860477,-1.99302733218635,-0.00156197182782427));
#36491=CARTESIAN_POINT('',(-6.97045488139522,-1.99798886456863,-2.89228984749754E-5));
#36492=CARTESIAN_POINT('',(-13.1285451186048,-1.99475,-1.92374832954336E-13));
#36493=CARTESIAN_POINT('Ctrl Pts',(-7.12854511860477,-1.99302733218635,
-0.00156197182782411));
#36494=CARTESIAN_POINT('Ctrl Pts',(-7.11476913628051,-1.99462045073153,
-0.217796874425585));
#36495=CARTESIAN_POINT('Ctrl Pts',(-7.05874979443432,-1.86269372181647,
-1.09521440278052));
#36496=CARTESIAN_POINT('Ctrl Pts',(-6.96048709306619,-0.584852130314656,
-2.28216593812101));
#36497=CARTESIAN_POINT('Ctrl Pts',(-6.83375701450043,1.59631522845185,-1.73266011521722));
#36498=CARTESIAN_POINT('Ctrl Pts',(-6.70702693593464,2.32234956235835,0.396264928634968));
#36499=CARTESIAN_POINT('Ctrl Pts',(-6.58029685736886,0.931428871827763,
2.16397172813741));
#36500=CARTESIAN_POINT('Ctrl Pts',(-6.45413625159224,-1.29847722763132,
1.96001463265738));
#36501=CARTESIAN_POINT('Ctrl Pts',(-6.37021900533753,-1.99720209314702,
0.649794423907979));
#36502=CARTESIAN_POINT('Ctrl Pts',(-6.32854511860477,-1.9979722269169,-0.000164116242220302));
#36503=CARTESIAN_POINT('Ctrl Pts',(-6.97045488139522,-1.99798865963142,
-2.89210683962205E-5));
#36504=CARTESIAN_POINT('Ctrl Pts',(-6.97035469463609,-1.99798899549594,
-0.00159142903403707));
#36505=CARTESIAN_POINT('Ctrl Pts',(-6.92801114835502,-1.99728097638184,
-0.661979064342672));
#36506=CARTESIAN_POINT('Ctrl Pts',(-6.84342424255203,-1.27746953458014,
-1.97949598010661));
#36507=CARTESIAN_POINT('Ctrl Pts',(-6.71669416398625,0.965455645273396,
-2.1490063154975));
#36508=CARTESIAN_POINT('Ctrl Pts',(-6.58996408542047,2.32831254761179,-0.359573952994307));
#36509=CARTESIAN_POINT('Ctrl Pts',(-6.4632340068547,1.56877882193404,1.75763072199189));
#36510=CARTESIAN_POINT('Ctrl Pts',(-6.33650392828891,-0.620786912340788,
2.27265403361463));
#36511=CARTESIAN_POINT('Ctrl Pts',(-6.23891088646909,-1.87116208516676,
1.07391421228489));
#36512=CARTESIAN_POINT('Ctrl Pts',(-6.18356120417119,-1.99489996679304,
0.207296227027028));
#36513=CARTESIAN_POINT('Ctrl Pts',(-6.17045488139522,-1.99329205388752,
0.00164168227339381));
#36514=CARTESIAN_POINT('Origin',(-13.1285451186048,0.,0.));
#36515=CARTESIAN_POINT('',(-7.92854511860477,-1.99250106198237,0.0013356187689274));
#36516=CARTESIAN_POINT('',(-7.77045488139522,-1.99321120987985,-0.00161938525380073));
#36517=CARTESIAN_POINT('',(-13.1285451186048,-1.99475,-1.92374832954336E-13));
#36518=CARTESIAN_POINT('Ctrl Pts',(-7.92854511860477,-1.99250106198237,
0.00133561876892717));
#36519=CARTESIAN_POINT('Ctrl Pts',(-7.90156262674539,-1.9898790361083,-0.422477199748252));
#36520=CARTESIAN_POINT('Ctrl Pts',(-7.83233677536409,-1.65025022702601,
-1.51364290830163));
#36521=CARTESIAN_POINT('Ctrl Pts',(-7.72086756446086,0.141974088420104,
-2.35163278207385));
#36522=CARTESIAN_POINT('Ctrl Pts',(-7.5941374858951,2.05014815624844,-1.16070061638369));
#36523=CARTESIAN_POINT('Ctrl Pts',(-7.46740740732931,2.08949441685714,1.08827683305561));
#36524=CARTESIAN_POINT('Ctrl Pts',(-7.34067732876354,0.224146493614207,
2.3452274373418));
#36525=CARTESIAN_POINT('Ctrl Pts',(-7.22772323252202,-1.62054376456912,
1.56012082295419));
#36526=CARTESIAN_POINT('Ctrl Pts',(-7.15701249580243,-1.98973523253938,
0.445276619472374));
#36527=CARTESIAN_POINT('Ctrl Pts',(-7.12854511860477,-1.99302733218635,
-0.00156197182782411));
#36528=CARTESIAN_POINT('Ctrl Pts',(-7.77045488139522,-1.99321120987985,
-0.0016193852538011));
#36529=CARTESIAN_POINT('Ctrl Pts',(-7.75714818510097,-1.99481690227094,
-0.210439444705621));
#36530=CARTESIAN_POINT('Ctrl Pts',(-7.7015981292848,-1.86864990103976,-1.08028727279676));
#36531=CARTESIAN_POINT('Ctrl Pts',(-7.6038047139467,-0.610050402621316,
-2.27555954730001));
#36532=CARTESIAN_POINT('Ctrl Pts',(-7.47707463538092,1.57705941561997,-1.75020465850163));
#36533=CARTESIAN_POINT('Ctrl Pts',(-7.35034455681515,2.32658898847186,0.370562310224418));
#36534=CARTESIAN_POINT('Ctrl Pts',(-7.22361447824936,0.955299056467363,
2.15354044767035));
#36535=CARTESIAN_POINT('Ctrl Pts',(-7.09698458644272,-1.28502834164932,
1.97358514194292));
#36536=CARTESIAN_POINT('Ctrl Pts',(-7.01259805415801,-1.99784737952166,
0.657234011746362));
#36537=CARTESIAN_POINT('Ctrl Pts',(-6.97045488139522,-1.99798865963142,
-2.89210683962205E-5));
#36538=CARTESIAN_POINT('Origin',(-13.1285451186048,0.,0.));
#36539=CARTESIAN_POINT('',(-8.72854511860477,-1.99778044304682,0.000580414400251015));
#36540=CARTESIAN_POINT('',(-8.57045488139522,-1.99235441329993,0.00125123217891654));
#36541=CARTESIAN_POINT('',(-13.1285451186048,-1.99475,-1.92374832954336E-13));
#36542=CARTESIAN_POINT('Ctrl Pts',(-8.72854511860477,-1.99778044304682,
0.000580414400251001));
#36543=CARTESIAN_POINT('Ctrl Pts',(-8.68835611721029,-1.99536078015132,
-0.626380726430122));
#36544=CARTESIAN_POINT('Ctrl Pts',(-8.60592375629387,-1.34009769434388,
-1.91671199912222));
#36545=CARTESIAN_POINT('Ctrl Pts',(-8.48124803585554,0.85516388839699,-2.19522848691248));
#36546=CARTESIAN_POINT('Ctrl Pts',(-8.35451795728975,2.30706713390257,-0.47725739709158));
#36547=CARTESIAN_POINT('Ctrl Pts',(-8.22778787872399,1.65594616616223,1.67576122332812));
#36548=CARTESIAN_POINT('Ctrl Pts',(-8.10105780015819,-0.504664851331058,
2.30122723164079));
#36549=CARTESIAN_POINT('Ctrl Pts',(-8.0013102134518,-1.8431691324066,1.14245048428309));
#36550=CARTESIAN_POINT('Ctrl Pts',(-7.94380598626732,-1.99398403805739,
0.241037399123113));
#36551=CARTESIAN_POINT('Ctrl Pts',(-7.92854511860477,-1.99250106198237,
0.00133561876892717));
#36552=CARTESIAN_POINT('Ctrl Pts',(-8.57045488139522,-1.99235441329993,
0.0012512321789164));
#36553=CARTESIAN_POINT('Ctrl Pts',(-8.54394167556586,-1.98995194175533,
-0.415267451224239));
#36554=CARTESIAN_POINT('Ctrl Pts',(-8.47518511021458,-1.65937989506407,
-1.49891452050869));
#36555=CARTESIAN_POINT('Ctrl Pts',(-8.36418518534137,0.11596324319048,-2.35305870594664));
#36556=CARTESIAN_POINT('Ctrl Pts',(-8.2374551067756,2.0371887677672,-1.1832982174768));
#36557=CARTESIAN_POINT('Ctrl Pts',(-8.11072502820981,2.10139971207879,1.06510656604636));
#36558=CARTESIAN_POINT('Ctrl Pts',(-7.98399494964405,0.250064112115891,
2.34260553378614));
#36559=CARTESIAN_POINT('Ctrl Pts',(-7.8705715673725,-1.61089390858375,1.57476690963073));
#36560=CARTESIAN_POINT('Ctrl Pts',(-7.7993915446229,-1.98971948068271,0.452479483610746));
#36561=CARTESIAN_POINT('Ctrl Pts',(-7.77045488139522,-1.99321120987985,
-0.0016193852538011));
#36562=CARTESIAN_POINT('Origin',(-13.1285451186048,0.,0.));
#36563=CARTESIAN_POINT('',(-9.52854511860476,-1.99413929912365,-0.00178482837013569));
#36564=CARTESIAN_POINT('',(-9.37045488139522,-1.99768040091508,0.000705460530160528));
#36565=CARTESIAN_POINT('',(-13.1285451186048,-1.99475,-1.92374832954336E-13));
#36566=CARTESIAN_POINT('Ctrl Pts',(-9.52854511860476,-1.99413929912365,
-0.00178482837013546));
#36567=CARTESIAN_POINT('Ctrl Pts',(-9.5173929671971,-1.99567604089445,-0.176587503202193));
#36568=CARTESIAN_POINT('Ctrl Pts',(-9.46399745626751,-1.89470323252639,
-1.0117808002804));
#36569=CARTESIAN_POINT('Ctrl Pts',(-9.368358585816,-0.724734298212267,-2.24167199518702));
#36570=CARTESIAN_POINT('Ctrl Pts',(-9.2416285072502,1.48621635193257,-1.82797549873587));
#36571=CARTESIAN_POINT('Ctrl Pts',(-9.11489842868443,2.34239544440841,0.252025761717839));
#36572=CARTESIAN_POINT('Ctrl Pts',(-8.98816835011866,1.06334653056341,2.10229101340218));
#36573=CARTESIAN_POINT('Ctrl Pts',(-8.86143827155287,-1.18500382101302,
2.03619727482286));
#36574=CARTESIAN_POINT('Ctrl Pts',(-8.77489719438158,-1.98270767494886,
0.723567688852132));
#36575=CARTESIAN_POINT('Ctrl Pts',(-8.73059947673221,-1.99790412997515,
0.03262905135474));
#36576=CARTESIAN_POINT('Ctrl Pts',(-8.72854511860477,-1.99778044304682,
0.000580414400251001));
#36577=CARTESIAN_POINT('Ctrl Pts',(-9.37045488139522,-1.99768040091508,
0.000705460530160329));
#36578=CARTESIAN_POINT('Ctrl Pts',(-9.33073516603075,-1.99484052238671,
-0.619017268744858));
#36579=CARTESIAN_POINT('Ctrl Pts',(-9.24877209114436,-1.35295791994823,
-1.90291681631474));
#36580=CARTESIAN_POINT('Ctrl Pts',(-9.12456565673604,0.830838775459797,
-2.20454977051161));
#36581=CARTESIAN_POINT('Ctrl Pts',(-8.99783557817027,2.30164890208838,-0.502737585433884));
#36582=CARTESIAN_POINT('Ctrl Pts',(-8.87110549960448,1.67437384270186,1.65734877959569));
#36583=CARTESIAN_POINT('Ctrl Pts',(-8.74437542103871,-0.479189150904811,
2.30666653572304));
#36584=CARTESIAN_POINT('Ctrl Pts',(-8.64415854830229,-1.83678140535602,
1.15737884639853));
#36585=CARTESIAN_POINT('Ctrl Pts',(-8.58618503508779,-1.99377978776735,
0.248369703929462));
#36586=CARTESIAN_POINT('Ctrl Pts',(-8.57045488139522,-1.99235441329993,
0.0012512321789164));
#36587=CARTESIAN_POINT('Origin',(-13.1285451186048,0.,0.));
#36588=CARTESIAN_POINT('',(-10.3285451186048,-1.99182186837539,0.000801948237002644));
#36589=CARTESIAN_POINT('',(-10.1704548813952,-1.99435467562299,-0.00179807465759962));
#36590=CARTESIAN_POINT('',(-13.1285451186048,-1.99475,-1.92374832954336E-13));
#36591=CARTESIAN_POINT('Ctrl Pts',(-10.3285451186048,-1.99182186837539,
0.000801948237002768));
#36592=CARTESIAN_POINT('Ctrl Pts',(-10.304186457662,-1.99043382219268,-0.38212649427497));
#36593=CARTESIAN_POINT('Ctrl Pts',(-10.2375844371973,-1.69972871911625,
-1.43109111249991));
#36594=CARTESIAN_POINT('Ctrl Pts',(-10.1287390572107,-0.00358806096914,
-2.35590932209698));
#36595=CARTESIAN_POINT('Ctrl Pts',(-10.0020089786449,1.97451952674142,-1.2851492017786));
#36596=CARTESIAN_POINT('Ctrl Pts',(-9.8752789000791,2.15273996627044,0.957102848135853));
#36597=CARTESIAN_POINT('Ctrl Pts',(-9.74854882151332,0.368613841216539,
2.32689825630081));
#36598=CARTESIAN_POINT('Ctrl Pts',(-9.63297089435521,-1.56495415031113,
1.64170776389411));
#36599=CARTESIAN_POINT('Ctrl Pts',(-9.55963632671902,-1.9898549994879,0.485549511297817));
#36600=CARTESIAN_POINT('Ctrl Pts',(-9.52854511860476,-1.99413929912365,
-0.00178482837013546));
#36601=CARTESIAN_POINT('Ctrl Pts',(-10.1704548813952,-1.99435467562299,
-0.00179807465759959));
#36602=CARTESIAN_POINT('Ctrl Pts',(-10.1597720160176,-1.99585127079878,
-0.16919896214573));
#36603=CARTESIAN_POINT('Ctrl Pts',(-10.106845791118,-1.90010097116099,-0.996867385757571));
#36604=CARTESIAN_POINT('Ctrl Pts',(-10.0116762066965,-0.749476153859556,
-2.23352110175442));
#36605=CARTESIAN_POINT('Ctrl Pts',(-9.88494612813071,1.46591330801472,-1.84429699356347));
#36606=CARTESIAN_POINT('Ctrl Pts',(-9.75821604956493,2.34503881318019,0.22611040137808));
#36607=CARTESIAN_POINT('Ctrl Pts',(-9.63148597099915,1.08652661928962,2.09040484243106));
#36608=CARTESIAN_POINT('Ctrl Pts',(-9.50475589243338,-1.16241693685793,
2.04917537014711));
#36609=CARTESIAN_POINT('Ctrl Pts',(-9.41774552923206,-1.97898996654308,
0.738376615426936));
#36610=CARTESIAN_POINT('Ctrl Pts',(-9.37297852555267,-1.99786083631826,
0.0400803561110824));
#36611=CARTESIAN_POINT('Ctrl Pts',(-9.37045488139522,-1.99768040091508,
0.000705460530160329));
#36612=CARTESIAN_POINT('Origin',(-13.1285451186048,0.,0.));
#36613=CARTESIAN_POINT('',(-11.1285451186048,-1.99700380788516,0.00135048458759499));
#36614=CARTESIAN_POINT('',(-10.9704548813952,-1.99173416440345,0.000704422997178239));
#36615=CARTESIAN_POINT('',(-13.1285451186048,-1.99475,-1.92374832954336E-13));
#36616=CARTESIAN_POINT('Ctrl Pts',(-11.1285451186048,-1.99700380788516,
0.00135048458759495));
#36617=CARTESIAN_POINT('Ctrl Pts',(-11.0909799481269,-1.99278503355486,
-0.585230740927899));
#36618=CARTESIAN_POINT('Ctrl Pts',(-11.0111714181271,-1.41024709685789,
-1.8391755479592));
#36619=CARTESIAN_POINT('Ctrl Pts',(-10.8891195286053,0.717923294984202,
-2.24374937306581));
#36620=CARTESIAN_POINT('Ctrl Pts',(-10.7623894500395,2.27316203258867,-0.618946575035767));
#36621=CARTESIAN_POINT('Ctrl Pts',(-10.6356593714738,1.75632236943564,1.57028323687515));
#36622=CARTESIAN_POINT('Ctrl Pts',(-10.508929292908,-0.361526663326025,
2.32799343505198));
#36623=CARTESIAN_POINT('Ctrl Pts',(-10.406557875285,-1.80608791742609,1.22590108173666));
#36624=CARTESIAN_POINT('Ctrl Pts',(-10.3464298171839,-1.99284100434719,
0.281956966889221));
#36625=CARTESIAN_POINT('Ctrl Pts',(-10.3285451186048,-1.99182186837539,
0.000801948237002768));
#36626=CARTESIAN_POINT('Ctrl Pts',(-10.9704548813952,-1.99173416440345,
0.000704422997178135));
#36627=CARTESIAN_POINT('Ctrl Pts',(-10.9465655064825,-1.99056444425807,
-0.37489151711618));
#36628=CARTESIAN_POINT('Ctrl Pts',(-10.8804327720478,-1.70818809927551,
-1.41629846064639));
#36629=CARTESIAN_POINT('Ctrl Pts',(-10.7720566780912,-0.0296318476642994,
-2.35571138038688));
#36630=CARTESIAN_POINT('Ctrl Pts',(-10.6453265995254,1.96018587726147,-1.30691036088261));
#36631=CARTESIAN_POINT('Ctrl Pts',(-10.5185965209596,2.16319248849083,0.933245180944391));
#36632=CARTESIAN_POINT('Ctrl Pts',(-10.3918664423938,0.394319168136422,
2.32267805209636));
#36633=CARTESIAN_POINT('Ctrl Pts',(-10.2758192292057,-1.5545868425617,1.65621678803195));
#36634=CARTESIAN_POINT('Ctrl Pts',(-10.2020153755395,-1.98993326979109,
0.492756011961213));
#36635=CARTESIAN_POINT('Ctrl Pts',(-10.1704548813952,-1.99435467562299,
-0.00179807465759959));
#36636=CARTESIAN_POINT('Ctrl Pts',(-11.9126273851832,-0.875140871775474,
1.79252782880715));
#36637=CARTESIAN_POINT('Ctrl Pts',(-11.8703840256612,-1.46986319122015,
1.50217484195868));
#36638=CARTESIAN_POINT('Ctrl Pts',(-11.7858973066174,-2.33753098893177,
0.288226582968726));
#36639=CARTESIAN_POINT('Ctrl Pts',(-11.6591672280516,-1.51239476231416,
-1.80838669328082));
#36640=CARTESIAN_POINT('Ctrl Pts',(-11.5324371494858,0.693331691078553,
-2.2508689680574));
#36641=CARTESIAN_POINT('Ctrl Pts',(-11.4057070709201,2.2660422239822,-0.644398977329155));
#36642=CARTESIAN_POINT('Ctrl Pts',(-11.2789769923543,1.77364945549679,1.55095382729707));
#36643=CARTESIAN_POINT('Ctrl Pts',(-11.1522469137885,-0.335801440579385,
2.33175063016555));
#36644=CARTESIAN_POINT('Ctrl Pts',(-11.0255168352227,-2.13900593722502,
0.987427802354548));
#36645=CARTESIAN_POINT('Ctrl Pts',(-10.898786756657,-1.99245923770595,-1.25720460847756));
#36646=CARTESIAN_POINT('Ctrl Pts',(-10.7720566780912,-0.0296318476642994,
-2.35571138038688));
#36647=CARTESIAN_POINT('Ctrl Pts',(-10.6453265995254,1.96018587726147,-1.30691036088261));
#36648=CARTESIAN_POINT('Ctrl Pts',(-10.5185965209596,2.16319248849083,0.933245180944391));
#36649=CARTESIAN_POINT('Ctrl Pts',(-10.3918664423938,0.394319168136422,
2.32267805209636));
#36650=CARTESIAN_POINT('Ctrl Pts',(-10.265136363828,-1.73399572256841,1.59486489712634));
#36651=CARTESIAN_POINT('Ctrl Pts',(-10.1384062852623,-2.28167548395771,
-0.586763647263183));
#36652=CARTESIAN_POINT('Ctrl Pts',(-10.0116762066965,-0.749476153859556,
-2.23352110175442));
#36653=CARTESIAN_POINT('Ctrl Pts',(-9.88494612813071,1.46591330801472,-1.84429699356347));
#36654=CARTESIAN_POINT('Ctrl Pts',(-9.75821604956493,2.34503881318019,0.22611040137808));
#36655=CARTESIAN_POINT('Ctrl Pts',(-9.63148597099915,1.08652661928962,2.09040484243106));
#36656=CARTESIAN_POINT('Ctrl Pts',(-9.50475589243338,-1.16241693685793,
2.04917537014711));
#36657=CARTESIAN_POINT('Ctrl Pts',(-9.37802581386759,-2.35175071733265,
0.140004748881306));
#36658=CARTESIAN_POINT('Ctrl Pts',(-9.25129573530182,-1.39732861457205,
-1.89678819466818));
#36659=CARTESIAN_POINT('Ctrl Pts',(-9.12456565673604,0.830838775459797,
-2.20454977051161));
#36660=CARTESIAN_POINT('Ctrl Pts',(-8.99783557817027,2.30164890208838,-0.502737585433884));
#36661=CARTESIAN_POINT('Ctrl Pts',(-8.87110549960448,1.67437384270186,1.65734877959569));
#36662=CARTESIAN_POINT('Ctrl Pts',(-8.74437542103871,-0.479189150904811,
2.30666653572304));
#36663=CARTESIAN_POINT('Ctrl Pts',(-8.61764534247293,-2.195943708986,0.853325245121742));
#36664=CARTESIAN_POINT('Ctrl Pts',(-8.49091526390715,-1.91096943851369,
-1.37787102135406));
#36665=CARTESIAN_POINT('Ctrl Pts',(-8.36418518534137,0.11596324319048,-2.35305870594664));
#36666=CARTESIAN_POINT('Ctrl Pts',(-8.2374551067756,2.0371887677672,-1.1832982174768));
#36667=CARTESIAN_POINT('Ctrl Pts',(-8.11072502820981,2.10139971207879,1.06510656604636));
#36668=CARTESIAN_POINT('Ctrl Pts',(-7.98399494964405,0.250064112115891,
2.34260553378614));
#36669=CARTESIAN_POINT('Ctrl Pts',(-7.85726487107825,-1.82921929001621,
1.48468499556677));
#36670=CARTESIAN_POINT('Ctrl Pts',(-7.73053479251248,-2.24106423689609,
-0.726611198051787));
#36671=CARTESIAN_POINT('Ctrl Pts',(-7.6038047139467,-0.610050402621316,
-2.27555954730001));
#36672=CARTESIAN_POINT('Ctrl Pts',(-7.47707463538092,1.57705941561997,-1.75020465850163));
#36673=CARTESIAN_POINT('Ctrl Pts',(-7.35034455681515,2.32658898847186,0.370562310224418));
#36674=CARTESIAN_POINT('Ctrl Pts',(-7.22361447824936,0.955299056467363,
2.15354044767035));
#36675=CARTESIAN_POINT('Ctrl Pts',(-7.09688439968359,-1.28680083895008,
1.97344276530014));
#36676=CARTESIAN_POINT('Ctrl Pts',(-6.97015432111781,-2.35590785438983,
-0.005561354392871));
#36677=CARTESIAN_POINT('Ctrl Pts',(-6.84342424255203,-1.27746953458014,
-1.97949598010661));
#36678=CARTESIAN_POINT('Ctrl Pts',(-6.71669416398625,0.965455645273396,
-2.1490063154975));
#36679=CARTESIAN_POINT('Ctrl Pts',(-6.58996408542047,2.32831254761179,-0.359573952994307));
#36680=CARTESIAN_POINT('Ctrl Pts',(-6.4632340068547,1.56877882193404,1.75763072199189));
#36681=CARTESIAN_POINT('Ctrl Pts',(-6.33650392828891,-0.620786912340788,
2.27265403361463));
#36682=CARTESIAN_POINT('Ctrl Pts',(-6.20977384972314,-2.24446971732477,
0.716022649816709));
#36683=CARTESIAN_POINT('Ctrl Pts',(-6.08304377115735,-1.82218945012484,
-1.49330450842827));
#36684=CARTESIAN_POINT('Ctrl Pts',(-5.95631369259159,0.261121169457012,
-2.34139883016539));
#36685=CARTESIAN_POINT('Ctrl Pts',(-5.8295836140258,2.10640484398777,-1.0551736256481));
#36686=CARTESIAN_POINT('Ctrl Pts',(-5.70285353546004,2.03157950898151,1.19290294899666));
#36687=CARTESIAN_POINT('Ctrl Pts',(-5.57612345689424,0.104852755347087,
2.35357996395588));
#36688=CARTESIAN_POINT('Ctrl Pts',(-5.44939337832848,-1.91745330764535,
1.36883364951275));
#36689=CARTESIAN_POINT('Ctrl Pts',(-5.32266329976268,-2.19189054006374,
-0.863683163791881));
#36690=CARTESIAN_POINT('Ctrl Pts',(-5.19593322119692,-0.468293640578219,
-2.30890316237654));
#36691=CARTESIAN_POINT('Ctrl Pts',(-5.06920314263113,1.68217981160309,-1.64942530248376));
#36692=CARTESIAN_POINT('Ctrl Pts',(-4.94247306406536,2.29924973922467,0.513598465451003));
#36693=CARTESIAN_POINT('Ctrl Pts',(-4.81574298549957,0.820421458075195,
2.20844773045863));
#36694=CARTESIAN_POINT('Ctrl Pts',(-4.68901290693381,-1.40626810803312,
1.89017003345429));
#36695=CARTESIAN_POINT('Ctrl Pts',(-4.56228282836801,-2.35106351606113,
-0.151106222517994));
#36696=CARTESIAN_POINT('Ctrl Pts',(-4.43555274980225,-1.15272948149133,
-2.05464047695385));
#36697=CARTESIAN_POINT('Ctrl Pts',(-4.30882267123646,1.09638368952585,-2.08525191580977));
#36698=CARTESIAN_POINT('Ctrl Pts',(-4.18209259267069,2.34608015003573,-0.215036454205511));
#36699=CARTESIAN_POINT('Ctrl Pts',(-4.0553625141049,1.45718979233537,1.85119708733083));
#36700=CARTESIAN_POINT('Ctrl Pts',(-3.92863243553913,-0.760012763696535,
2.22995814895977));
#36701=CARTESIAN_POINT('Ctrl Pts',(-3.80190235697335,-2.28442002961604,
0.575984266494282));
#36702=CARTESIAN_POINT('Ctrl Pts',(-3.67517227840757,-1.72644721895094,
-1.60303235999064));
#36703=CARTESIAN_POINT('Ctrl Pts',(-3.5484421998418,0.405281400923077,-2.3207929105089));
#36704=CARTESIAN_POINT('Ctrl Pts',(-3.42171212127601,2.16757274388305,-0.923017413918032));
#36705=CARTESIAN_POINT('Ctrl Pts',(-3.29498204271024,1.95399702329888,1.3161414741343));
#36706=CARTESIAN_POINT('Ctrl Pts',(-3.16825196414445,-0.0407592243607493,
2.35556180878339));
#36707=CARTESIAN_POINT('Ctrl Pts',(-3.04152188557869,-1.99836109667082,
1.24775224690805));
#36708=CARTESIAN_POINT('Ctrl Pts',(-2.9147918070129,-2.13434204335348,-0.997455157020213));
#36709=CARTESIAN_POINT('Ctrl Pts',(-2.78806172844712,-0.324747614573964,
-2.33342489664845));
#36710=CARTESIAN_POINT('Ctrl Pts',(-2.66133164988135,1.78087291120639,-1.54234379652064));
#36711=CARTESIAN_POINT('Ctrl Pts',(-2.53460157131557,2.26312549748712,0.654672245331693));
#36712=CARTESIAN_POINT('Ctrl Pts',(-2.40787149274979,0.682409168923879,
2.25491697383304));
#36713=CARTESIAN_POINT('Ctrl Pts',(-2.28114141418401,-1.520362263158,1.79967527305601));
#36714=CARTESIAN_POINT('Ctrl Pts',(-2.15441133561823,-2.33723626077076,
-0.296073656834323));
#36715=CARTESIAN_POINT('Ctrl Pts',(-2.02768125705245,-1.02358496316198,
-2.12193474222715));
#36716=CARTESIAN_POINT('Ctrl Pts',(-1.90095117848668,1.22312246187489,-2.01352985089457));
#36717=CARTESIAN_POINT('Ctrl Pts',(-1.77422109992089,2.35488419618976,-0.0696779332279315));
#36718=CARTESIAN_POINT('Ctrl Pts',(-1.64749102135512,1.34003240157303,1.9376915050404));
#36719=CARTESIAN_POINT('Ctrl Pts',(-1.52076094278934,-0.896333389432558,
2.17873986401275));
#36720=CARTESIAN_POINT('Ctrl Pts',(-1.39403086422356,-2.31564459579178,
0.43374925475368));
#36721=CARTESIAN_POINT('Ctrl Pts',(-1.26730078565778,-1.6241036154426,-1.7066431411118));
#36722=CARTESIAN_POINT('Ctrl Pts',(-1.14057070709201,0.54788370586334,-2.29130478089007));
#36723=CARTESIAN_POINT('Ctrl Pts',(-1.01384062852623,2.22047671979483,-0.787362926702919));
#36724=CARTESIAN_POINT('Ctrl Pts',(-0.887110549960448,1.86891443749856,
1.43440541328318));
#36725=CARTESIAN_POINT('Ctrl Pts',(-0.760380471394668,-0.186150183504844,
2.34844027344827));
#36726=CARTESIAN_POINT('Ctrl Pts',(-0.633650392828891,-2.0717580026336,
1.12210023790887));
#36727=CARTESIAN_POINT('Ctrl Pts',(-0.506920314263113,-2.06840119353109,
-1.12779160550707));
#36728=CARTESIAN_POINT('Ctrl Pts',(-0.380190235697333,-0.180414554165581,
-2.34831227349832));
#36729=CARTESIAN_POINT('Ctrl Pts',(-0.253460157131555,1.87363647225322,
-1.43076438289222));
#36730=CARTESIAN_POINT('Ctrl Pts',(-0.126730078565778,2.21660082027165,
0.796119646106798));
#36731=CARTESIAN_POINT('Ctrl Pts',(-0.0422433595219261,1.10280973225228,
1.78908852524606));
#36732=CARTESIAN_POINT('Ctrl Pts',(0.,0.458732584425967,1.94128616604711));
#36733=CARTESIAN_POINT('Ctrl Pts',(-11.8249182567888,-0.94179006796741,
1.92904360906013));
#36734=CARTESIAN_POINT('Ctrl Pts',(-11.7826748972669,-1.58180539774536,
1.61657784721794));
#36735=CARTESIAN_POINT('Ctrl Pts',(-11.698188178223,-2.51555325541557,0.31017741476688));
#36736=CARTESIAN_POINT('Ctrl Pts',(-11.5714580996572,-1.62757609880992,
-1.94611025687904));
#36737=CARTESIAN_POINT('Ctrl Pts',(-11.4447280210914,0.746134618464435,
-2.42229120679946));
#36738=CARTESIAN_POINT('Ctrl Pts',(-11.3179979425257,2.43862003132311,-0.693475274930001));
#36739=CARTESIAN_POINT('Ctrl Pts',(-11.1912678639599,1.90872749189947,1.66907175465481));
#36740=CARTESIAN_POINT('Ctrl Pts',(-11.0645377853941,-0.36137549021701,
2.50933267464865));
#36741=CARTESIAN_POINT('Ctrl Pts',(-10.9378077068283,-2.30190888344055,
1.06262857453539));
#36742=CARTESIAN_POINT('Ctrl Pts',(-10.8110776282626,-2.14420144392804,
-1.35295110976236));
#36743=CARTESIAN_POINT('Ctrl Pts',(-10.6843475496968,-0.0318885572892489,
-2.53511823364523));
#36744=CARTESIAN_POINT('Ctrl Pts',(-10.557617471131,2.10947020087126,-1.40644236522273));
#36745=CARTESIAN_POINT('Ctrl Pts',(-10.4308873925652,2.32793744009374,1.00431949956666));
#36746=CARTESIAN_POINT('Ctrl Pts',(-10.3041573139994,0.424349825424849,
2.49956914492218));
#36747=CARTESIAN_POINT('Ctrl Pts',(-10.1774272354337,-1.86605380011539,
1.71632701466244));
#36748=CARTESIAN_POINT('Ctrl Pts',(-10.0506971568679,-2.4554438930004,-0.631450539060834));
#36749=CARTESIAN_POINT('Ctrl Pts',(-9.9239670783021,-0.806554945207108,
-2.40362215737953));
#36750=CARTESIAN_POINT('Ctrl Pts',(-9.79723699973633,1.57755469835229,-1.98475542274283));
#36751=CARTESIAN_POINT('Ctrl Pts',(-9.67050692117054,2.52363286241057,0.243330573568071));
#36752=CARTESIAN_POINT('Ctrl Pts',(-9.54377684260477,1.16927458382007,2.24960641438041));
#36753=CARTESIAN_POINT('Ctrl Pts',(-9.41704676403899,-1.25094457507039,
2.20523697769101));
#36754=CARTESIAN_POINT('Ctrl Pts',(-9.29031668547321,-2.53085593342896,
0.150667265370884));
#36755=CARTESIAN_POINT('Ctrl Pts',(-9.16358660690743,-1.50374671476695,
-2.04124426179772));
#36756=CARTESIAN_POINT('Ctrl Pts',(-9.03685652834166,0.894114001580982,
-2.37244442028571));
#36757=CARTESIAN_POINT('Ctrl Pts',(-8.91012644977588,2.47693845167718,-0.541025199514446));
#36758=CARTESIAN_POINT('Ctrl Pts',(-8.78339637121009,1.80189122229186,1.78356956019488));
#36759=CARTESIAN_POINT('Ctrl Pts',(-8.65666629264432,-0.515683357451122,
2.48233821950225));
#36760=CARTESIAN_POINT('Ctrl Pts',(-8.52993621407855,-2.36318293618579,
0.918313001392679));
#36761=CARTESIAN_POINT('Ctrl Pts',(-8.40320613551275,-2.05650552433943,
-1.48280726532483));
#36762=CARTESIAN_POINT('Ctrl Pts',(-8.27647605694698,0.124794800709627,
-2.53226353616516));
#36763=CARTESIAN_POINT('Ctrl Pts',(-8.14974597838121,2.19233749666553,-1.2734161374526));
#36764=CARTESIAN_POINT('Ctrl Pts',(-8.02301589981542,2.26143863404562,1.14622321683394));
#36765=CARTESIAN_POINT('Ctrl Pts',(-7.89628582124965,0.269108556966443,
2.52101426871917));
#36766=CARTESIAN_POINT('Ctrl Pts',(-7.76955574268387,-1.96852942769843,
1.59775600475416));
#36767=CARTESIAN_POINT('Ctrl Pts',(-7.64282566411809,-2.41173976448358,
-0.781948634407555));
#36768=CARTESIAN_POINT('Ctrl Pts',(-7.51609558555232,-0.656510772925826,
-2.44886217731746));
#36769=CARTESIAN_POINT('Ctrl Pts',(-7.38936550698653,1.69716549886662,-1.88349718022318));
#36770=CARTESIAN_POINT('Ctrl Pts',(-7.26263542842076,2.50377793136296,0.398783686818758));
#36771=CARTESIAN_POINT('Ctrl Pts',(-7.13590534985498,1.02805295962734,2.31755031674763));
#36772=CARTESIAN_POINT('Ctrl Pts',(-7.00917527128919,-1.38480133731686,
2.12373671028666));
#36773=CARTESIAN_POINT('Ctrl Pts',(-6.88244519272344,-2.53532967076417,
-0.00598489740401535));
#36774=CARTESIAN_POINT('Ctrl Pts',(-6.75571511415763,-1.37475937714771,
-2.130250927332));
#36775=CARTESIAN_POINT('Ctrl Pts',(-6.62898503559187,1.03898305644994,-2.31267087300897));
#36776=CARTESIAN_POINT('Ctrl Pts',(-6.50225495702608,2.50563275374858,-0.386958475545549));
#36777=CARTESIAN_POINT('Ctrl Pts',(-6.37552487846031,1.68825426966709,1.89148879970384));
#36778=CARTESIAN_POINT('Ctrl Pts',(-6.24879479989453,-0.668064956423038,
2.44573538479814));
#36779=CARTESIAN_POINT('Ctrl Pts',(-6.12206472132875,-2.4154046003378,0.770553680882268));
#36780=CARTESIAN_POINT('Ctrl Pts',(-5.99533464276297,-1.96096420751206,
-1.60703196462012));
#36781=CARTESIAN_POINT('Ctrl Pts',(-5.8686045641972,0.281007700430807,-2.51971566466393));
#36782=CARTESIAN_POINT('Ctrl Pts',(-5.74187448563141,2.26682494803545,-1.13553380109017));
#36783=CARTESIAN_POINT('Ctrl Pts',(-5.61514440706564,2.18630104655403,1.28375234850456));
#36784=CARTESIAN_POINT('Ctrl Pts',(-5.48841432849986,0.11283815756951,2.53282449227153));
#36785=CARTESIAN_POINT('Ctrl Pts',(-5.36168424993408,-2.06348319358917,
1.47308162307093));
#36786=CARTESIAN_POINT('Ctrl Pts',(-5.2349541713683,-2.35882108501659,-0.929459761009253));
#36787=CARTESIAN_POINT('Ctrl Pts',(-5.10822409280252,-0.503958064139003,
-2.48474518372476));
#36788=CARTESIAN_POINT('Ctrl Pts',(-4.98149401423675,1.81029168011427,-1.77504264494222));
#36789=CARTESIAN_POINT('Ctrl Pts',(-4.85476393567096,2.47435657277135,0.552713225133368));
#36790=CARTESIAN_POINT('Ctrl Pts',(-4.7280338571052,0.88290331954787,2.37663924203594));
#36791=CARTESIAN_POINT('Ctrl Pts',(-4.6013037785394,-1.51336702439457,2.03412207301595));
#36792=CARTESIAN_POINT('Ctrl Pts',(-4.47457369997363,-2.53011639611208,
-0.162614207798099));
#36793=CARTESIAN_POINT('Ctrl Pts',(-4.34784362140785,-1.24051934006839,
-2.21111829746129));
#36794=CARTESIAN_POINT('Ctrl Pts',(-4.22111354284208,1.17988235126313,-2.24406104989179));
#36795=CARTESIAN_POINT('Ctrl Pts',(-4.09438346427629,2.52475350565737,-0.231413253972277));
#36796=CARTESIAN_POINT('Ctrl Pts',(-3.96765338571052,1.56816681499601,1.99218101556761));
#36797=CARTESIAN_POINT('Ctrl Pts',(-3.84092330714474,-0.817894004796855,
2.39978785633972));
#36798=CARTESIAN_POINT('Ctrl Pts',(-3.71419322857896,-2.45839745844964,
0.619850219530145));
#36799=CARTESIAN_POINT('Ctrl Pts',(-3.58746315001318,-1.85793041568185,
-1.72511649719508));
#36800=CARTESIAN_POINT('Ctrl Pts',(-3.4607330714474,0.43614692266274,-2.4975404342528));
#36801=CARTESIAN_POINT('Ctrl Pts',(-3.33400299288163,2.33265128806564,-0.993312803715125));
#36802=CARTESIAN_POINT('Ctrl Pts',(-3.20727291431584,2.1028100146292,1.41637650389352));
#36803=CARTESIAN_POINT('Ctrl Pts',(-3.08054283575007,-0.0438633755078936,
2.53495727093036));
#36804=CARTESIAN_POINT('Ctrl Pts',(-2.95381275718429,-2.15055277813595,
1.34277887288933));
#36805=CARTESIAN_POINT('Ctrl Pts',(-2.82708267861851,-2.29688979557947,
-1.07341959497182));
#36806=CARTESIAN_POINT('Ctrl Pts',(-2.70035260005274,-0.349479824181215,
-2.5111344503348));
#36807=CARTESIAN_POINT('Ctrl Pts',(-2.57362252148695,1.91650107334572,-1.6598059990129));
#36808=CARTESIAN_POINT('Ctrl Pts',(-2.44689244292118,2.43548117204613,0.704530937032375));
#36809=CARTESIAN_POINT('Ctrl Pts',(-2.3201623643554,0.734380256150712,2.42664750160584));
#36810=CARTESIAN_POINT('Ctrl Pts',(-2.19343228578962,-1.63615039056481,
1.93673539014593));
#36811=CARTESIAN_POINT('Ctrl Pts',(-2.06670220722384,-2.51523608127396,
-0.31862210803575));
#36812=CARTESIAN_POINT('Ctrl Pts',(-1.93997212865807,-1.10153940138919,
-2.2835375761278));
#36813=CARTESIAN_POINT('Ctrl Pts',(-1.81324205009228,1.31627332656126,-2.1668767581169));
#36814=CARTESIAN_POINT('Ctrl Pts',(-1.68651197152651,2.53422805254828,-0.0749844825981518));
#36815=CARTESIAN_POINT('Ctrl Pts',(-1.55978189296073,1.4420869225267,2.08526269665541));
#36816=CARTESIAN_POINT('Ctrl Pts',(-1.43305181439495,-0.964596570655569,
2.34466887650786));
#36817=CARTESIAN_POINT('Ctrl Pts',(-1.30632173582917,-2.49200003290288,
0.466782838386398));
#36818=CARTESIAN_POINT('Ctrl Pts',(-1.17959165726339,-1.74779250256096,
-1.83661809395662));
#36819=CARTESIAN_POINT('Ctrl Pts',(-1.05286157869762,0.58960956941301,-2.46580654032369));
#36820=CARTESIAN_POINT('Ctrl Pts',(-0.926131500131837,2.38958433813404,
-0.847327108320492));
#36821=CARTESIAN_POINT('Ctrl Pts',(-0.799401421566058,2.01124768809639,
1.54364721753663));
#36822=CARTESIAN_POINT('Ctrl Pts',(-0.672671343000278,-0.200327055482492,
2.52729337193581));
#36823=CARTESIAN_POINT('Ctrl Pts',(-0.5459412644345,-2.22953946391951,1.20755742693457));
#36824=CARTESIAN_POINT('Ctrl Pts',(-0.419211185868724,-2.22592700611442,
-1.21368223912194));
#36825=CARTESIAN_POINT('Ctrl Pts',(-0.292481107302943,-0.194154610657383,
-2.52715562373383));
#36826=CARTESIAN_POINT('Ctrl Pts',(-0.165751028737165,2.01632934474841,
-1.53972889264753));
#36827=CARTESIAN_POINT('Ctrl Pts',(-0.0390209501713877,2.38541325689092,
0.856750724138811));
#36828=CARTESIAN_POINT('Ctrl Pts',(0.0454657688724642,1.18679779014993,
1.92534237416295));
#36829=CARTESIAN_POINT('Ctrl Pts',(0.0877091283943902,0.493668854694124,
2.08913112074919));
#36830=CARTESIAN_POINT('Ctrl Pts',(-11.7372091283944,-1.00843926415935,
2.06555938931311));
#36831=CARTESIAN_POINT('Ctrl Pts',(-11.6949657688725,-1.69374760427058,
1.73098085247721));
#36832=CARTESIAN_POINT('Ctrl Pts',(-11.6104790498286,-2.69357552189936,
0.332128246565033));
#36833=CARTESIAN_POINT('Ctrl Pts',(-11.4837489712628,-1.74275743530568,
-2.08383382047727));
#36834=CARTESIAN_POINT('Ctrl Pts',(-11.3570188926971,0.798937545850312,
-2.59371344554152));
#36835=CARTESIAN_POINT('Ctrl Pts',(-11.2302888141313,2.61119783866403,-0.742551572530846));
#36836=CARTESIAN_POINT('Ctrl Pts',(-11.1035587355655,2.04380552830215,1.78718968201255));
#36837=CARTESIAN_POINT('Ctrl Pts',(-10.9768286569997,-0.386949539854633,
2.68691471913174));
#36838=CARTESIAN_POINT('Ctrl Pts',(-10.850098578434,-2.46481182965607,1.13782934671622));
#36839=CARTESIAN_POINT('Ctrl Pts',(-10.7233684998681,-2.29594365015013,
-1.44869761104716));
#36840=CARTESIAN_POINT('Ctrl Pts',(-10.5966384213024,-0.0341452669142003,
-2.71452508690359));
#36841=CARTESIAN_POINT('Ctrl Pts',(-10.4699083427366,2.25875452448105,-1.50597436956284));
#36842=CARTESIAN_POINT('Ctrl Pts',(-10.3431782641708,2.49268239169665,1.07539381818893));
#36843=CARTESIAN_POINT('Ctrl Pts',(-10.216448185605,0.454380482713277,2.676460237748));
#36844=CARTESIAN_POINT('Ctrl Pts',(-10.0897181070393,-1.99811187766236,
1.83778913219854));
#36845=CARTESIAN_POINT('Ctrl Pts',(-9.96298802847347,-2.6292123020431,-0.676137430858485));
#36846=CARTESIAN_POINT('Ctrl Pts',(-9.83625794990772,-0.863633736554661,
-2.57372321300464));
#36847=CARTESIAN_POINT('Ctrl Pts',(-9.70952787134193,1.68919608868986,-2.1252138519222));
#36848=CARTESIAN_POINT('Ctrl Pts',(-9.58279779277616,2.70222691164095,0.260550745758062));
#36849=CARTESIAN_POINT('Ctrl Pts',(-9.45606771421037,1.25202254835052,2.40880798632976));
#36850=CARTESIAN_POINT('Ctrl Pts',(-9.3293376356446,-1.33947221328284,2.36129858523491));
#36851=CARTESIAN_POINT('Ctrl Pts',(-9.20260755707882,-2.70996114952527,
0.161329781860462));
#36852=CARTESIAN_POINT('Ctrl Pts',(-9.07587747851304,-1.61016481496184,
-2.18570032892727));
#36853=CARTESIAN_POINT('Ctrl Pts',(-8.94914739994727,0.957389227702167,
-2.54033907005982));
#36854=CARTESIAN_POINT('Ctrl Pts',(-8.82241732138147,2.65222800126598,-0.579312813595004));
#36855=CARTESIAN_POINT('Ctrl Pts',(-8.69568724281571,1.92940860188185,1.90979034079406));
#36856=CARTESIAN_POINT('Ctrl Pts',(-8.56895716424992,-0.552177563997433,
2.65800990328147));
#36857=CARTESIAN_POINT('Ctrl Pts',(-8.44222708568415,-2.53042216338558,
0.98330075766361));
#36858=CARTESIAN_POINT('Ctrl Pts',(-8.31549700711837,-2.20204161016517,
-1.58774350929558));
#36859=CARTESIAN_POINT('Ctrl Pts',(-8.18876692855259,0.133626358228775,
-2.71146836638369));
#36860=CARTESIAN_POINT('Ctrl Pts',(-8.06203684998682,2.34748622556386,-1.36353405742839));
#36861=CARTESIAN_POINT('Ctrl Pts',(-7.93530677142103,2.42147755601244,1.22733986762151));
#36862=CARTESIAN_POINT('Ctrl Pts',(-7.80857669285527,0.288153001816996,
2.69942300365221));
#36863=CARTESIAN_POINT('Ctrl Pts',(-7.68184661428947,-2.10783956538065,
1.71082701394155));
#36864=CARTESIAN_POINT('Ctrl Pts',(-7.5551165357237,-2.58241529207107,-0.837286070763322));
#36865=CARTESIAN_POINT('Ctrl Pts',(-7.42838645715792,-0.702971143230335,
-2.62216480733491));
#36866=CARTESIAN_POINT('Ctrl Pts',(-7.30165637859214,1.81727158211326,-2.01678970194473));
#36867=CARTESIAN_POINT('Ctrl Pts',(-7.17492630002637,2.68096687425406,0.427005063413098));
#36868=CARTESIAN_POINT('Ctrl Pts',(-7.04819622146058,1.10080686278732,2.48156018582491));
#36869=CARTESIAN_POINT('Ctrl Pts',(-6.92146614289481,-1.48280183568364,
2.27403065527319));
#36870=CARTESIAN_POINT('Ctrl Pts',(-6.79473606432903,-2.71475148713851,
-0.0064084404151617));
#36871=CARTESIAN_POINT('Ctrl Pts',(-6.66800598576325,-1.47204921971528,
-2.28100587455739));
#36872=CARTESIAN_POINT('Ctrl Pts',(-6.54127590719748,1.11251046762649,-2.47633543052044));
#36873=CARTESIAN_POINT('Ctrl Pts',(-6.41454582863169,2.68295295988536,-0.414342998096788));
#36874=CARTESIAN_POINT('Ctrl Pts',(-6.28781575006593,1.80772971740014,2.02534687741579));
#36875=CARTESIAN_POINT('Ctrl Pts',(-6.16108567150013,-0.715343000505289,
2.61881673598164));
#36876=CARTESIAN_POINT('Ctrl Pts',(-6.03435559293437,-2.58633948335083,
0.825084711947826));
#36877=CARTESIAN_POINT('Ctrl Pts',(-5.90762551436857,-2.09973896489927,
-1.72075942081198));
#36878=CARTESIAN_POINT('Ctrl Pts',(-5.78089543580281,0.3008942314046,-2.69803249916247));
#36879=CARTESIAN_POINT('Ctrl Pts',(-5.65416535723702,2.42724505208314,-1.21589397653224));
#36880=CARTESIAN_POINT('Ctrl Pts',(-5.52743527867125,2.34102258412655,1.37460174801246));
#36881=CARTESIAN_POINT('Ctrl Pts',(-5.40070520010546,0.120823559791933,
2.71206902058717));
#36882=CARTESIAN_POINT('Ctrl Pts',(-5.27397512153969,-2.20951307953299,
1.5773295966291));
#36883=CARTESIAN_POINT('Ctrl Pts',(-5.14724504297391,-2.52575162996943,
-0.995236358226622));
#36884=CARTESIAN_POINT('Ctrl Pts',(-5.02051496440813,-0.539622487699786,
-2.66058720507298));
#36885=CARTESIAN_POINT('Ctrl Pts',(-4.89378488584236,1.93840354862544,-1.90065998740068));
#36886=CARTESIAN_POINT('Ctrl Pts',(-4.76705480727657,2.64946340631802,0.591827984815734));
#36887=CARTESIAN_POINT('Ctrl Pts',(-4.64032472871081,0.945385181020546,
2.54483075361324));
#36888=CARTESIAN_POINT('Ctrl Pts',(-4.51359465014501,-1.62046594075601,
2.17807411257761));
#36889=CARTESIAN_POINT('Ctrl Pts',(-4.38686457157924,-2.70916927616302,
-0.174122193078205));
#36890=CARTESIAN_POINT('Ctrl Pts',(-4.26013449301346,-1.32830919864544,
-2.36759611796874));
#36891=CARTESIAN_POINT('Ctrl Pts',(-4.13340441444769,1.26338101300041,-2.40287018397382));
#36892=CARTESIAN_POINT('Ctrl Pts',(-4.00667433588191,2.70342686127901,-0.247790053739041));
#36893=CARTESIAN_POINT('Ctrl Pts',(-3.87994425731612,1.67914383765664,2.13316494380439));
#36894=CARTESIAN_POINT('Ctrl Pts',(-3.75321417875035,-0.875775245897177,
2.56961756371967));
#36895=CARTESIAN_POINT('Ctrl Pts',(-3.62648410018457,-2.63237488728325,
0.663716172566008));
#36896=CARTESIAN_POINT('Ctrl Pts',(-3.49975402161879,-1.98941361241277,
-1.84720063439951));
#36897=CARTESIAN_POINT('Ctrl Pts',(-3.37302394305301,0.467012444402406,
-2.6742879579967));
#36898=CARTESIAN_POINT('Ctrl Pts',(-3.24629386448724,2.49772983224823,-1.06360819351221));
#36899=CARTESIAN_POINT('Ctrl Pts',(-3.11956378592145,2.25162300595954,1.51661153365274));
#36900=CARTESIAN_POINT('Ctrl Pts',(-2.99283370735568,-0.0469675266550418,
2.71435273307734));
#36901=CARTESIAN_POINT('Ctrl Pts',(-2.8661036287899,-2.30274445960107,1.4378054988706));
#36902=CARTESIAN_POINT('Ctrl Pts',(-2.73937355022412,-2.45943754780547,
-1.14938403292342));
#36903=CARTESIAN_POINT('Ctrl Pts',(-2.61264347165834,-0.374212033788463,
-2.68884400402115));
#36904=CARTESIAN_POINT('Ctrl Pts',(-2.48591339309257,2.05212923548504,-1.77726820150518));
#36905=CARTESIAN_POINT('Ctrl Pts',(-2.35918331452679,2.60783684660515,0.754389628733061));
#36906=CARTESIAN_POINT('Ctrl Pts',(-2.23245323596101,0.786351343377539,
2.59837802937863));
#36907=CARTESIAN_POINT('Ctrl Pts',(-2.10572315739523,-1.75193851797162,
2.07379550723585));
#36908=CARTESIAN_POINT('Ctrl Pts',(-1.97899307882945,-2.69323590177716,
-0.341170559237177));
#36909=CARTESIAN_POINT('Ctrl Pts',(-1.85226300026368,-1.17949383961639,
-2.44514041002845));
#36910=CARTESIAN_POINT('Ctrl Pts',(-1.72553292169789,1.40942419124763,-2.32022366533924));
#36911=CARTESIAN_POINT('Ctrl Pts',(-1.59880284313212,2.7135719089068,-0.0802910319683703));
#36912=CARTESIAN_POINT('Ctrl Pts',(-1.47207276456634,1.54414144348037,2.23283388827042));
#36913=CARTESIAN_POINT('Ctrl Pts',(-1.34534268600056,-1.03285975187858,
2.51059788900296));
#36914=CARTESIAN_POINT('Ctrl Pts',(-1.21861260743478,-2.66835547001398,
0.499816422019115));
#36915=CARTESIAN_POINT('Ctrl Pts',(-1.091882528869,-1.87148138967931,-1.96659304680144));
#36916=CARTESIAN_POINT('Ctrl Pts',(-0.965152450303224,0.631335432962678,
-2.64030829975732));
#36917=CARTESIAN_POINT('Ctrl Pts',(-0.83842237173745,2.55869195647326,-0.907291289938061));
#36918=CARTESIAN_POINT('Ctrl Pts',(-0.711692293171666,2.15358093869421,
1.65288902179009));
#36919=CARTESIAN_POINT('Ctrl Pts',(-0.584962214605889,-0.214503927460137,
2.70614647042334));
#36920=CARTESIAN_POINT('Ctrl Pts',(-0.45823213604011,-2.38732092520542,
1.29301461596027));
#36921=CARTESIAN_POINT('Ctrl Pts',(-0.331502057474334,-2.38345281869776,
-1.2995728727368));
#36922=CARTESIAN_POINT('Ctrl Pts',(-0.204771978908552,-0.207894667149185,
-2.70599897396934));
#36923=CARTESIAN_POINT('Ctrl Pts',(-0.0780419003427751,2.1590222172436,
-1.64869340240284));
#36924=CARTESIAN_POINT('Ctrl Pts',(0.0486881782230028,2.55422569351019,
0.917381802170824));
#36925=CARTESIAN_POINT('Ctrl Pts',(0.133174897266854,1.27078584804759,2.06159622307983));
#36926=CARTESIAN_POINT('Ctrl Pts',(0.17541825678878,0.528605124962282,2.23697607545127));
#36927=CARTESIAN_POINT('Ctrl Pts',(-11.6495,-1.07508846035128,2.20207516956609));
#36928=CARTESIAN_POINT('Ctrl Pts',(-11.6072566404781,-1.8056898107958,1.84538385773647));
#36929=CARTESIAN_POINT('Ctrl Pts',(-11.5227699214342,-2.87159778838315,
0.354079078363186));
#36930=CARTESIAN_POINT('Ctrl Pts',(-11.3960398428684,-1.85793877180144,
-2.22155738407549));
#36931=CARTESIAN_POINT('Ctrl Pts',(-11.2693097643027,0.851740473236193,
-2.76513568428359));
#36932=CARTESIAN_POINT('Ctrl Pts',(-11.1425796857369,2.78377564600494,-0.791627870131692));
#36933=CARTESIAN_POINT('Ctrl Pts',(-11.0158496071711,2.17888356470483,1.90530760937029));
#36934=CARTESIAN_POINT('Ctrl Pts',(-10.8891195286053,-0.412523589492258,
2.86449676361484));
#36935=CARTESIAN_POINT('Ctrl Pts',(-10.7623894500395,-2.6277147758716,1.21303011889706));
#36936=CARTESIAN_POINT('Ctrl Pts',(-10.6356593714738,-2.44768585637222,
-1.54444411233196));
#36937=CARTESIAN_POINT('Ctrl Pts',(-10.508929292908,-0.036401976539149,
-2.89393194016194));
#36938=CARTESIAN_POINT('Ctrl Pts',(-10.3821992143422,2.40803884809083,-1.60550637390296));
#36939=CARTESIAN_POINT('Ctrl Pts',(-10.2554691357764,2.65742734329957,1.1464681368112));
#36940=CARTESIAN_POINT('Ctrl Pts',(-10.1287390572106,0.484411140001705,
2.85335133057382));
#36941=CARTESIAN_POINT('Ctrl Pts',(-10.0020089786449,-2.13016995520933,
1.95925124973464));
#36942=CARTESIAN_POINT('Ctrl Pts',(-9.87527890007908,-2.80298071108579,
-0.720824322656137));
#36943=CARTESIAN_POINT('Ctrl Pts',(-9.74854882151334,-0.920712527902214,
-2.74382426862974));
#36944=CARTESIAN_POINT('Ctrl Pts',(-9.62181874294753,1.80083747902744,-2.26567228110156));
#36945=CARTESIAN_POINT('Ctrl Pts',(-9.49508866438176,2.88082096087132,0.277770917948053));
#36946=CARTESIAN_POINT('Ctrl Pts',(-9.36835858581599,1.33477051288097,2.56800955827911));
#36947=CARTESIAN_POINT('Ctrl Pts',(-9.24162850725019,-1.4279998514953,2.51736019277881));
#36948=CARTESIAN_POINT('Ctrl Pts',(-9.11489842868444,-2.88906636562158,
0.171992298350041));
#36949=CARTESIAN_POINT('Ctrl Pts',(-8.98816835011864,-1.71658291515674,
-2.33015639605681));
#36950=CARTESIAN_POINT('Ctrl Pts',(-8.86143827155288,1.02066445382335,-2.70823371983393));
#36951=CARTESIAN_POINT('Ctrl Pts',(-8.73470819298709,2.82751755085477,-0.617600427675567));
#36952=CARTESIAN_POINT('Ctrl Pts',(-8.60797811442131,2.05692598147186,2.03601112139324));
#36953=CARTESIAN_POINT('Ctrl Pts',(-8.48124803585554,-0.588671770543746,
2.83368158706069));
#36954=CARTESIAN_POINT('Ctrl Pts',(-8.35451795728976,-2.69766139058536,
1.04828851393454));
#36955=CARTESIAN_POINT('Ctrl Pts',(-8.22778787872398,-2.34757769599091,
-1.69267975326635));
#36956=CARTESIAN_POINT('Ctrl Pts',(-8.1010578001582,0.142457915747924,-2.8906731966022));
#36957=CARTESIAN_POINT('Ctrl Pts',(-7.97432772159243,2.50263495446219,-1.45365197740418));
#36958=CARTESIAN_POINT('Ctrl Pts',(-7.84759764302664,2.58151647797926,1.30845651840909));
#36959=CARTESIAN_POINT('Ctrl Pts',(-7.72086756446088,0.307197446667551,
2.87783173858525));
#36960=CARTESIAN_POINT('Ctrl Pts',(-7.59413748589508,-2.24714970306288,
1.82389802312894));
#36961=CARTESIAN_POINT('Ctrl Pts',(-7.46740740732932,-2.75309081965856,
-0.892623507119088));
#36962=CARTESIAN_POINT('Ctrl Pts',(-7.34067732876353,-0.749431513534847,
-2.79546743735237));
#36963=CARTESIAN_POINT('Ctrl Pts',(-7.21394725019776,1.9373776653599,-2.15008222366628));
#36964=CARTESIAN_POINT('Ctrl Pts',(-7.08721717163197,2.85815581714516,0.455226440007436));
#36965=CARTESIAN_POINT('Ctrl Pts',(-6.9604870930662,1.1735607659473,2.6455700549022));
#36966=CARTESIAN_POINT('Ctrl Pts',(-6.83375701450042,-1.58080233405042,
2.42432460025971));
#36967=CARTESIAN_POINT('Ctrl Pts',(-6.70702693593464,-2.89417330351285,
-0.00683198342630554));
#36968=CARTESIAN_POINT('Ctrl Pts',(-6.58029685736886,-1.56933906228285,
-2.43176082178278));
#36969=CARTESIAN_POINT('Ctrl Pts',(-6.45356677880308,1.18603787880304,-2.63999998803191));
#36970=CARTESIAN_POINT('Ctrl Pts',(-6.32683670023731,2.86027316602215,-0.441727520648026));
#36971=CARTESIAN_POINT('Ctrl Pts',(-6.20010662167153,1.9272051651332,2.15920495512774));
#36972=CARTESIAN_POINT('Ctrl Pts',(-6.07337654310574,-0.762621044587542,
2.79189808716515));
#36973=CARTESIAN_POINT('Ctrl Pts',(-5.94664646453997,-2.75727436636386,
0.87961574301338));
#36974=CARTESIAN_POINT('Ctrl Pts',(-5.81991638597419,-2.23851372228649,
-1.83448687700383));
#36975=CARTESIAN_POINT('Ctrl Pts',(-5.69318630740841,0.320780762378395,
-2.87634933366101));
#36976=CARTESIAN_POINT('Ctrl Pts',(-5.56645622884264,2.58766515613083,-1.29625415197431));
#36977=CARTESIAN_POINT('Ctrl Pts',(-5.43972615027686,2.49574412169908,1.46545114752035));
#36978=CARTESIAN_POINT('Ctrl Pts',(-5.31299607171107,0.128808962014357,
2.89131354890282));
#36979=CARTESIAN_POINT('Ctrl Pts',(-5.18626599314531,-2.35554296547681,
1.68157757018728));
#36980=CARTESIAN_POINT('Ctrl Pts',(-5.05953591457952,-2.69268217492228,
-1.06101295544399));
#36981=CARTESIAN_POINT('Ctrl Pts',(-4.93280583601374,-0.575286911260571,
-2.8364292264212));
#36982=CARTESIAN_POINT('Ctrl Pts',(-4.80607575744797,2.06651541713663,-2.02627732985914));
#36983=CARTESIAN_POINT('Ctrl Pts',(-4.67934567888219,2.82457023986469,0.630942744498098));
#36984=CARTESIAN_POINT('Ctrl Pts',(-4.55261560031641,1.00786704249322,2.71302226519054));
#36985=CARTESIAN_POINT('Ctrl Pts',(-4.42588552175063,-1.72756485711747,
2.32202615213927));
#36986=CARTESIAN_POINT('Ctrl Pts',(-4.29915544318485,-2.88822215621396,
-0.18563017835831));
#36987=CARTESIAN_POINT('Ctrl Pts',(-4.17242536461907,-1.41609905722251,
-2.52407393847618));
#36988=CARTESIAN_POINT('Ctrl Pts',(-4.04569528605329,1.34687967473769,-2.56167931805584));
#36989=CARTESIAN_POINT('Ctrl Pts',(-3.91896520748752,2.88210021690064,-0.264166853505807));
#36990=CARTESIAN_POINT('Ctrl Pts',(-3.79223512892173,1.79012086031728,2.27414887204118));
#36991=CARTESIAN_POINT('Ctrl Pts',(-3.66550505035596,-0.933656486997501,
2.73944727109961));
#36992=CARTESIAN_POINT('Ctrl Pts',(-3.53877497179018,-2.80635231611685,
0.707582125601873));
#36993=CARTESIAN_POINT('Ctrl Pts',(-3.4120448932244,-2.12089680914368,-1.96928477160395));
#36994=CARTESIAN_POINT('Ctrl Pts',(-3.28531481465862,0.49787796614207,-2.85103548174061));
#36995=CARTESIAN_POINT('Ctrl Pts',(-3.15858473609284,2.66280837643082,-1.1339035833093));
#36996=CARTESIAN_POINT('Ctrl Pts',(-3.03185465752707,2.40043599728986,1.61684656341196));
#36997=CARTESIAN_POINT('Ctrl Pts',(-2.90512457896129,-0.0500716778021863,
2.89374819522431));
#36998=CARTESIAN_POINT('Ctrl Pts',(-2.77839450039551,-2.4549361410662,1.53283212485187));
#36999=CARTESIAN_POINT('Ctrl Pts',(-2.65166442182973,-2.62198530003146,
-1.22534847087502));
#37000=CARTESIAN_POINT('Ctrl Pts',(-2.52493434326395,-0.398944243395714,
-2.86655355770749));
#37001=CARTESIAN_POINT('Ctrl Pts',(-2.39820426469817,2.18775739762436,-1.89473040399744));
#37002=CARTESIAN_POINT('Ctrl Pts',(-2.2714741861324,2.78019252116416,0.804248320433746));
#37003=CARTESIAN_POINT('Ctrl Pts',(-2.14474410756662,0.838322430604369,
2.77010855715143));
#37004=CARTESIAN_POINT('Ctrl Pts',(-2.01801402900084,-1.86772664537843,
2.21085562432577));
#37005=CARTESIAN_POINT('Ctrl Pts',(-1.89128395043506,-2.87123572228036,
-0.363719010438602));
#37006=CARTESIAN_POINT('Ctrl Pts',(-1.76455387186928,-1.2574482778436,-2.60674324392911));
#37007=CARTESIAN_POINT('Ctrl Pts',(-1.6378237933035,1.50257505593399,-2.47357057256157));
#37008=CARTESIAN_POINT('Ctrl Pts',(-1.51109371473772,2.89291576526532,-0.0855975813385903));
#37009=CARTESIAN_POINT('Ctrl Pts',(-1.38436363617195,1.64619596443404,2.38040507988543));
#37010=CARTESIAN_POINT('Ctrl Pts',(-1.25763355760617,-1.10112293310158,
2.67652690149807));
#37011=CARTESIAN_POINT('Ctrl Pts',(-1.13090347904039,-2.84471090712508,
0.532850005651832));
#37012=CARTESIAN_POINT('Ctrl Pts',(-1.00417340047461,-1.99517027679767,
-2.09656799964626));
#37013=CARTESIAN_POINT('Ctrl Pts',(-0.877443321908835,0.673061296512348,
-2.81481005919094));
#37014=CARTESIAN_POINT('Ctrl Pts',(-0.750713243343059,2.72779957481248,
-0.967255471555635));
#37015=CARTESIAN_POINT('Ctrl Pts',(-0.623983164777276,2.29591418929203,
1.76213082604354));
#37016=CARTESIAN_POINT('Ctrl Pts',(-0.497253086211499,-0.228680799437782,
2.88499956891088));
#37017=CARTESIAN_POINT('Ctrl Pts',(-0.370523007645719,-2.54510238649133,
1.37847180498597));
#37018=CARTESIAN_POINT('Ctrl Pts',(-0.243792929079943,-2.5409786312811,
-1.38546350635167));
#37019=CARTESIAN_POINT('Ctrl Pts',(-0.117062850514162,-0.221634723640988,
-2.88484232420485));
#37020=CARTESIAN_POINT('Ctrl Pts',(0.0096672280516153,2.30171508973879,
-1.75765791215815));
#37021=CARTESIAN_POINT('Ctrl Pts',(0.136397306617393,2.72303813012945,0.978012880202838));
#37022=CARTESIAN_POINT('Ctrl Pts',(0.220884025661244,1.35477390594525,2.19785007199671));
#37023=CARTESIAN_POINT('Ctrl Pts',(0.263127385183171,0.563541395230439,
2.38482103015336));
#37024=CARTESIAN_POINT('',(0.,1.82956213026058,-1.63023086141699));
#37025=CARTESIAN_POINT('Ctrl Pts',(1.11022302462516E-16,1.83311928606617,
-1.63215490580859));
#37026=CARTESIAN_POINT('Ctrl Pts',(3.35691596827958E-16,1.87020221509191,
-1.58263650689979));
#37027=CARTESIAN_POINT('Ctrl Pts',(1.7799849765391E-15,1.90522161173578,
-1.53170199440537));
#37028=CARTESIAN_POINT('Ctrl Pts',(8.88178419700125E-16,1.93804364176405,
-1.47939865304506));
#37029=CARTESIAN_POINT('Ctrl Pts',(-1.77793102530655E-16,1.98336980933887,
-1.40716942124011));
#37030=CARTESIAN_POINT('Ctrl Pts',(5.39107183348623E-16,2.02450743199428,
-1.33232980239994));
#37031=CARTESIAN_POINT('Ctrl Pts',(-5.27355936696949E-16,2.06143695913673,
-1.25527886014649));
#37032=CARTESIAN_POINT('Ctrl Pts',(-1.06429201921402E-15,2.08003000305954,
-1.21648574080632));
#37033=CARTESIAN_POINT('Ctrl Pts',(2.02892540791524E-15,2.09755555354514,
-1.17713185376445));
#37034=CARTESIAN_POINT('Ctrl Pts',(1.97064586870965E-15,2.11400625054454,
-1.13726744031613));
#37035=CARTESIAN_POINT('Ctrl Pts',(1.9422168992414E-15,2.12203095988682,
-1.11782143562494));
#37036=CARTESIAN_POINT('Ctrl Pts',(4.11823233707136E-15,2.12979985614877,
-1.09825394858399));
#37037=CARTESIAN_POINT('Ctrl Pts',(4.27435864480685E-15,2.13731180430856,
-1.07857082222221));
#37038=CARTESIAN_POINT('Ctrl Pts',(4.40132187367308E-15,2.14342058384275,
-1.06256433802797));
#37039=CARTESIAN_POINT('Ctrl Pts',(-1.81383465133899E-15,2.14935611980056,
-1.04648998991835));
#37040=CARTESIAN_POINT('Ctrl Pts',(-1.52655665885959E-15,2.15511691042516,
-1.03035523241857));
#37041=CARTESIAN_POINT('Ctrl Pts',(-1.0238845684058E-16,2.18367578037281,
-0.950367871116878));
#37042=CARTESIAN_POINT('Ctrl Pts',(5.79434641801055E-15,2.20795681184397,
-0.868863550066977));
#37043=CARTESIAN_POINT('Ctrl Pts',(4.57966997657877E-15,2.22793924709077,
-0.786237832279718));
#37044=CARTESIAN_POINT('Ctrl Pts',(3.64166789715849E-15,2.24337015953301,
-0.72243228501259));
#37045=CARTESIAN_POINT('Ctrl Pts',(-2.13542367938229E-16,2.25623663051347,
-0.657957590807845));
#37046=CARTESIAN_POINT('Ctrl Pts',(-9.99200722162641E-16,2.26650784188907,
-0.592996429696028));
#37047=CARTESIAN_POINT('Ctrl Pts',(-1.39260515725901E-15,2.27165096814395,
-0.56046828466583));
#37048=CARTESIAN_POINT('Ctrl Pts',(-2.30199172467359E-16,2.276143089034,
-0.527818207731014));
#37049=CARTESIAN_POINT('Ctrl Pts',(-3.88578058618805E-16,2.27997860287735,
-0.49506956990305));
#37050=CARTESIAN_POINT('Ctrl Pts',(-4.77966372939306E-16,2.28214334923554,
-0.476586389456036));
#37051=CARTESIAN_POINT('Ctrl Pts',(1.21427467872323E-15,2.28409919911833,
-0.458067593765231));
#37052=CARTESIAN_POINT('Ctrl Pts',(1.22124532708767E-15,2.28584270747282,
-0.439545337752037));
#37053=CARTESIAN_POINT('Ctrl Pts',(1.2524054674238E-15,2.29363652551706,
-0.356747287048907));
#37054=CARTESIAN_POINT('Ctrl Pts',(2.98674777348732E-15,2.29720513916532,
-0.273778886552983));
#37055=CARTESIAN_POINT('Ctrl Pts',(2.33146835171283E-15,2.29652846067949,
-0.19100810983232));
#37056=CARTESIAN_POINT('Ctrl Pts',(1.68915238065727E-15,2.29586516898396,
-0.109874794703355));
#37057=CARTESIAN_POINT('Ctrl Pts',(3.98927178069262E-15,2.29112266840023,
-0.0289304327025789));
#37058=CARTESIAN_POINT('Ctrl Pts',(4.63518112781003E-15,2.28223399867317,
0.0514685248767753));
#37059=CARTESIAN_POINT('Ctrl Pts',(5.26622813180739E-15,2.27354985681052,
0.130017506295588));
#37060=CARTESIAN_POINT('Ctrl Pts',(-5.74427027136191E-16,2.26090793882628,
0.208046647240463));
#37061=CARTESIAN_POINT('Ctrl Pts',(-3.33066907387547E-16,2.24420274952171,
0.285201797779823));
#37062=CARTESIAN_POINT('Ctrl Pts',(-2.43223168602901E-16,2.23798442038849,
0.313921982366105));
#37063=CARTESIAN_POINT('Ctrl Pts',(1.74108706017718E-15,2.2312026560155,
0.342520788687836));
#37064=CARTESIAN_POINT('Ctrl Pts',(1.74860126378462E-15,2.22385052915109,
0.370978839784131));
#37065=CARTESIAN_POINT('Ctrl Pts',(1.75230874467845E-15,2.22022301633633,
0.385019939310695));
#37066=CARTESIAN_POINT('Ctrl Pts',(-1.10164963276453E-15,2.21645664217309,
0.399026762935435));
#37067=CARTESIAN_POINT('Ctrl Pts',(-1.08246744900953E-15,2.21255050287209,
0.412996918792799));
#37068=CARTESIAN_POINT('Ctrl Pts',(-1.06630207080745E-15,2.20925868688716,
0.424769971113676));
#37069=CARTESIAN_POINT('Ctrl Pts',(3.14036835259962E-15,2.20587022064258,
0.436507639975992));
#37070=CARTESIAN_POINT('Ctrl Pts',(3.08086889333481E-15,2.20238504581408,
0.448208492551131));
#37071=CARTESIAN_POINT('Ctrl Pts',(2.70032584026761E-15,2.18009477484193,
0.523044099755827));
#37072=CARTESIAN_POINT('Ctrl Pts',(1.67653588062007E-15,2.15385146753471,
0.596378577822135));
#37073=CARTESIAN_POINT('Ctrl Pts',(1.72084568816899E-15,2.12359651477114,
0.667885141097565));
#37074=CARTESIAN_POINT('Ctrl Pts',(1.73741029882426E-15,2.11228611780386,
0.694616883921002));
#37075=CARTESIAN_POINT('Ctrl Pts',(-1.7751156820648E-15,2.10041461978735,
0.721092938851344));
#37076=CARTESIAN_POINT('Ctrl Pts',(-1.66533453693773E-15,2.08797732702981,
0.747295272013091));
#37077=CARTESIAN_POINT('Ctrl Pts',(-1.36557198820265E-15,2.05401671774622,
0.818841967598024));
#37078=CARTESIAN_POINT('Ctrl Pts',(2.10526653845581E-15,2.01584013144301,
0.888350571890128));
#37079=CARTESIAN_POINT('Ctrl Pts',(2.37310171513627E-15,1.97374114073884,
0.955596271977286));
#37080=CARTESIAN_POINT('Ctrl Pts',(2.63446996854363E-15,1.9326586369134,
1.02121831385681));
#37081=CARTESIAN_POINT('Ctrl Pts',(5.41294650752726E-16,1.88783990086501,
1.08468576120073));
#37082=CARTESIAN_POINT('Ctrl Pts',(5.68989300120393E-16,1.83953150843297,
1.14575058726299));
#37083=CARTESIAN_POINT('Ctrl Pts',(5.7480995700391E-16,1.82937840726139,
1.15858474145074));
#37084=CARTESIAN_POINT('Ctrl Pts',(2.09061406733528E-15,1.81906844436066,
1.17131562858466));
#37085=CARTESIAN_POINT('Ctrl Pts',(2.13717932240343E-15,1.80862151941036,
1.18391988280963));
#37086=CARTESIAN_POINT('Ctrl Pts',(2.358433526946E-15,1.75898309122153,
1.24380883302188));
#37087=CARTESIAN_POINT('Ctrl Pts',(3.18887734197556E-15,1.70618592804151,
1.30093322236681));
#37088=CARTESIAN_POINT('Ctrl Pts',(1.85962356624714E-15,1.65052993023653,
1.35510174998724));
#37089=CARTESIAN_POINT('Ctrl Pts',(5.3128362391325E-16,1.59491219473355,
1.40923303790945));
#37090=CARTESIAN_POINT('Ctrl Pts',(-1.69124579543603E-15,1.53643861743996,
1.46041303633541));
#37091=CARTESIAN_POINT('Ctrl Pts',(-2.27595720048157E-15,1.47538001259375,
1.50840761508891));
#37092=CARTESIAN_POINT('Ctrl Pts',(-2.85094123198906E-15,1.41533719066528,
1.55560374662331));
#37093=CARTESIAN_POINT('Ctrl Pts',(-1.60428500839505E-16,1.35279374628381,
1.59971990299823));
#37094=CARTESIAN_POINT('Ctrl Pts',(-8.11850586757146E-16,1.28799325731152,
1.64048554490097));
#37095=CARTESIAN_POINT('Ctrl Pts',(-1.06202854919824E-15,1.26310669812549,
1.65614154651545));
#37096=CARTESIAN_POINT('Ctrl Pts',(-6.10864375227674E-16,1.2378871606073,
1.671302834036));
#37097=CARTESIAN_POINT('Ctrl Pts',(-7.56339435525888E-16,1.21234829708237,
1.68595199882551));
#37098=CARTESIAN_POINT('Ctrl Pts',(-8.17640432114187E-16,1.20158660512911,
1.69212493595262));
#37099=CARTESIAN_POINT('Ctrl Pts',(1.56771109887162E-15,1.19076801370443,
1.69820693920532));
#37100=CARTESIAN_POINT('Ctrl Pts',(1.56125112837913E-15,1.17990651797273,
1.70418977564566));
#37101=CARTESIAN_POINT('Ctrl Pts',(1.52217870306378E-15,1.11421194842586,
1.74037630780726));
#37102=CARTESIAN_POINT('Ctrl Pts',(-3.32055172913184E-16,1.04683370283974,
1.77300608886991));
#37103=CARTESIAN_POINT('Ctrl Pts',(-4.85722573273506E-17,0.97802182017074,
1.80187351209679));
#37104=CARTESIAN_POINT('Ctrl Pts',(2.3032739167331E-16,0.910322467340964,
1.83027421550035));
#37105=CARTESIAN_POINT('Ctrl Pts',(-3.29174076884851E-16,0.841234638235302,
1.85503349815338));
#37106=CARTESIAN_POINT('Ctrl Pts',(-1.21430643318376E-16,0.770987551814153,
1.87590662840547));
#37107=CARTESIAN_POINT('Ctrl Pts',(7.96662066757932E-17,0.702987964255391,
1.8961119396933));
#37108=CARTESIAN_POINT('Ctrl Pts',(1.21052487671592E-16,0.633901450878722,
1.91267585920164));
#37109=CARTESIAN_POINT('Ctrl Pts',(-1.55257751099924E-16,0.563938259187892,
1.92532798546484));
#37110=CARTESIAN_POINT('Ctrl Pts',(-2.92932647256323E-16,0.529078258365518,
1.93163205938258));
#37111=CARTESIAN_POINT('Ctrl Pts',(6.23284630163641E-17,0.494000706321858,
1.93696420018631));
#37112=CARTESIAN_POINT('Ctrl Pts',(0.,0.458732584425967,1.94128616604711));
#37113=CARTESIAN_POINT('Ctrl Pts',(-0.307327496212056,-2.44646461313235,
-7.12799915801969E-5));
#37114=CARTESIAN_POINT('Ctrl Pts',(-0.286149307168018,-2.44640487853515,
-0.409278547049527));
#37115=CARTESIAN_POINT('Ctrl Pts',(-0.264971118123981,-2.34924893135542,
-0.818477401716759));
#37116=CARTESIAN_POINT('Ctrl Pts',(-0.243792929079942,-2.15510860587612,
-1.17470409077093));
#37117=CARTESIAN_POINT('Ctrl Pts',(-0.201549569558017,-1.76786399540107,
-1.88525644563605));
#37118=CARTESIAN_POINT('Ctrl Pts',(-0.15930621003609,-0.994749359521043,
-2.38504938492044));
#37119=CARTESIAN_POINT('Ctrl Pts',(-0.117062850514165,-0.187633739351079,
-2.4470817858882));
#37120=CARTESIAN_POINT('Ctrl Pts',(-0.0780419003427761,0.557913460342055,
-2.50438222919026));
#37121=CARTESIAN_POINT('Ctrl Pts',(-0.0390209501713872,1.33247216588429,
-2.18816135588657));
#37122=CARTESIAN_POINT('Ctrl Pts',(1.2490009027033E-15,1.8331192860662,
-1.63215490580856));
#37123=CARTESIAN_POINT('',(-11.6495,-1.16034898466906,-1.62253437445174));
#37124=CARTESIAN_POINT('Ctrl Pts',(-11.6495,-1.16282838272805,-1.62470001792843));
#37125=CARTESIAN_POINT('Ctrl Pts',(-11.6495,-1.20737062417396,-1.60007728866689));
#37126=CARTESIAN_POINT('Ctrl Pts',(-11.6495,-1.25082068484827,-1.57369074934353));
#37127=CARTESIAN_POINT('Ctrl Pts',(-11.6495,-1.2930601147943,-1.54556381430646));
#37128=CARTESIAN_POINT('Ctrl Pts',(-11.6495,-1.35275072455609,-1.50581626313832));
#37129=CARTESIAN_POINT('Ctrl Pts',(-11.6495,-1.4100250943243,-1.4625955098447));
#37130=CARTESIAN_POINT('Ctrl Pts',(-11.6495,-1.46480184196881,-1.41624486913394));
#37131=CARTESIAN_POINT('Ctrl Pts',(-11.6495,-1.49642999741264,-1.3894819572715));
#37132=CARTESIAN_POINT('Ctrl Pts',(-11.6495,-1.52722514655207,-1.36167461307911));
#37133=CARTESIAN_POINT('Ctrl Pts',(-11.6495,-1.55716837922547,-1.3328819584687));
#37134=CARTESIAN_POINT('Ctrl Pts',(-11.6495,-1.56777135753634,-1.3226864029094));
#37135=CARTESIAN_POINT('Ctrl Pts',(-11.6495,-1.57826909663807,-1.31236563771069));
#37136=CARTESIAN_POINT('Ctrl Pts',(-11.6495,-1.58865543938623,-1.30192742989216));
#37137=CARTESIAN_POINT('Ctrl Pts',(-11.6495,-1.64145689071544,-1.24886231010381));
#37138=CARTESIAN_POINT('Ctrl Pts',(-11.6495,-1.69128391428968,-1.19286573360743));
#37139=CARTESIAN_POINT('Ctrl Pts',(-11.6495,-1.73804986103682,-1.13431476634906));
#37140=CARTESIAN_POINT('Ctrl Pts',(-11.6495,-1.77743172266821,-1.08500867396049));
#37141=CARTESIAN_POINT('Ctrl Pts',(-11.6495,-1.81464268770884,-1.0338899671485));
#37142=CARTESIAN_POINT('Ctrl Pts',(-11.6495,-1.84961682596229,-0.981158846144615));
#37143=CARTESIAN_POINT('Ctrl Pts',(-11.6495,-1.86647192782428,-0.95574611375999));
#37144=CARTESIAN_POINT('Ctrl Pts',(-11.6495,-1.88280729537051,-0.929958580884817));
#37145=CARTESIAN_POINT('Ctrl Pts',(-11.6495,-1.89861422754426,-0.903817116040125));
#37146=CARTESIAN_POINT('Ctrl Pts',(-11.6495,-1.9058390612283,-0.891868704186114));
#37147=CARTESIAN_POINT('Ctrl Pts',(-11.6495,-1.91295470835595,-0.879844221187209));
#37148=CARTESIAN_POINT('Ctrl Pts',(-11.6495,-1.91995627982203,-0.86775251788438));
#37149=CARTESIAN_POINT('Ctrl Pts',(-11.6495,-1.95884003755814,-0.800600327248006));
#37150=CARTESIAN_POINT('Ctrl Pts',(-11.6495,-1.9941235221355,-0.731526978428571));
#37151=CARTESIAN_POINT('Ctrl Pts',(-11.6495,-2.02571637553995,-0.660913112382761));
#37152=CARTESIAN_POINT('Ctrl Pts',(-11.6495,-2.0584793484816,-0.587683886996029));
#37153=CARTESIAN_POINT('Ctrl Pts',(-11.6495,-2.08727405704258,-0.512797249958379));
#37154=CARTESIAN_POINT('Ctrl Pts',(-11.6495,-2.11196354206791,-0.436633606374266));
#37155=CARTESIAN_POINT('Ctrl Pts',(-11.6495,-2.13048065583691,-0.379510873686182));
#37156=CARTESIAN_POINT('Ctrl Pts',(-11.6495,-2.14668789055987,-0.32166880515796));
#37157=CARTESIAN_POINT('Ctrl Pts',(-11.6495,-2.1605106338825,-0.263256315368801));
#37158=CARTESIAN_POINT('Ctrl Pts',(-11.6495,-2.17087769137447,-0.219446948026931));
#37159=CARTESIAN_POINT('Ctrl Pts',(-11.6495,-2.17990318743524,-0.175316499307717));
#37160=CARTESIAN_POINT('Ctrl Pts',(-11.6495,-2.18754943061712,-0.130925494906403));
#37161=CARTESIAN_POINT('Ctrl Pts',(-11.6495,-2.18995384688195,-0.116966423705573));
#37162=CARTESIAN_POINT('Ctrl Pts',(-11.6495,-2.19222183574009,-0.102981577419542));
#37163=CARTESIAN_POINT('Ctrl Pts',(-11.6495,-2.19435210579768,-0.0889728138154531));
#37164=CARTESIAN_POINT('Ctrl Pts',(-11.6495,-2.19617602412986,-0.0769786346466959));
#37165=CARTESIAN_POINT('Ctrl Pts',(-11.6495,-2.19789753243822,-0.0649764515061904));
#37166=CARTESIAN_POINT('Ctrl Pts',(-11.6495,-2.19951620912844,-0.052968022700671));
#37167=CARTESIAN_POINT('Ctrl Pts',(-11.6495,-2.21033880808821,0.0273212715633298));
#37168=CARTESIAN_POINT('Ctrl Pts',(-11.6495,-2.21656893840084,0.10789384853219));
#37169=CARTESIAN_POINT('Ctrl Pts',(-11.6495,-2.21807674608418,0.188374054145962));
#37170=CARTESIAN_POINT('Ctrl Pts',(-11.6495,-2.21859286329889,0.215922142685333));
#37171=CARTESIAN_POINT('Ctrl Pts',(-11.6495,-2.21855530302174,0.243459652058912));
#37172=CARTESIAN_POINT('Ctrl Pts',(-11.6495,-2.21795761289143,0.270972168827435));
#37173=CARTESIAN_POINT('Ctrl Pts',(-11.6495,-2.21627102067576,0.348608379068655));
#37174=CARTESIAN_POINT('Ctrl Pts',(-11.6495,-2.2101281442622,0.426045052693772));
#37175=CARTESIAN_POINT('Ctrl Pts',(-11.6495,-2.1997617102457,0.503031799881565));
#37176=CARTESIAN_POINT('Ctrl Pts',(-11.6495,-2.18918095360188,0.58161022284716));
#37177=CARTESIAN_POINT('Ctrl Pts',(-11.6495,-2.17420007249142,0.659720697636032));
#37178=CARTESIAN_POINT('Ctrl Pts',(-11.6495,-2.15501262324688,0.737098841831874));
#37179=CARTESIAN_POINT('Ctrl Pts',(-11.6495,-2.15035875822838,0.755866705860072));
#37180=CARTESIAN_POINT('Ctrl Pts',(-11.6495,-2.14545522714254,0.774598052202702));
#37181=CARTESIAN_POINT('Ctrl Pts',(-11.6495,-2.14031447676813,0.793253811565047));
#37182=CARTESIAN_POINT('Ctrl Pts',(-11.6495,-2.11881533699752,0.871274090482765));
#37183=CARTESIAN_POINT('Ctrl Pts',(-11.6495,-2.09315279746427,0.948060275340426));
#37184=CARTESIAN_POINT('Ctrl Pts',(-11.6495,-2.06360314980312,1.02334283907926));
#37185=CARTESIAN_POINT('Ctrl Pts',(-11.6495,-2.03346473222344,1.10012539054816));
#37186=CARTESIAN_POINT('Ctrl Pts',(-11.6495,-1.99928257575015,1.17534462999745));
#37187=CARTESIAN_POINT('Ctrl Pts',(-11.6495,-1.9612944536973,1.24871635014604));
#37188=CARTESIAN_POINT('Ctrl Pts',(-11.6495,-1.92301128002754,1.3226579443367));
#37189=CARTESIAN_POINT('Ctrl Pts',(-11.6495,-1.88086246501352,1.39472412259045));
#37190=CARTESIAN_POINT('Ctrl Pts',(-11.6495,-1.83503975229434,1.46461255055414));
#37191=CARTESIAN_POINT('Ctrl Pts',(-11.6495,-1.81559616867206,1.49426774582094));
#37192=CARTESIAN_POINT('Ctrl Pts',(-11.6495,-1.79549050001335,1.52353061819257));
#37193=CARTESIAN_POINT('Ctrl Pts',(-11.6495,-1.77473484362459,1.5523768230785));
#37194=CARTESIAN_POINT('Ctrl Pts',(-11.6495,-1.76427959115328,1.56690752975781));
#37195=CARTESIAN_POINT('Ctrl Pts',(-11.6495,-1.75365636602808,1.58133631474072));
#37196=CARTESIAN_POINT('Ctrl Pts',(-11.6495,-1.74288499727145,1.59563608488518));
#37197=CARTESIAN_POINT('Ctrl Pts',(-11.6495,-1.69122789171288,1.66421462420599));
#37198=CARTESIAN_POINT('Ctrl Pts',(-11.6495,-1.63610074686772,1.72992393044111));
#37199=CARTESIAN_POINT('Ctrl Pts',(-11.6495,-1.5777607315452,1.79246828497059));
#37200=CARTESIAN_POINT('Ctrl Pts',(-11.6495,-1.51932500291965,1.85511525049058));
#37201=CARTESIAN_POINT('Ctrl Pts',(-11.6495,-1.45766541888288,1.91458780561411));
#37202=CARTESIAN_POINT('Ctrl Pts',(-11.6495,-1.39299120107362,1.97057137326597));
#37203=CARTESIAN_POINT('Ctrl Pts',(-11.6495,-1.32967814016095,2.02537669057656));
#37204=CARTESIAN_POINT('Ctrl Pts',(-11.6495,-1.26347544514419,2.07683912052618));
#37205=CARTESIAN_POINT('Ctrl Pts',(-11.6495,-1.19453988778704,2.12463431235531));
#37206=CARTESIAN_POINT('Ctrl Pts',(-11.6495,-1.15558812056379,2.15164079867228));
#37207=CARTESIAN_POINT('Ctrl Pts',(-11.6495,-1.11576313904794,2.17747582457847));
#37208=CARTESIAN_POINT('Ctrl Pts',(-11.6495,-1.07508846035129,2.20207516956608));
#37209=CARTESIAN_POINT('Ctrl Pts',(-11.6495,-1.16282838272804,-1.62470001792844));
#37210=CARTESIAN_POINT('Ctrl Pts',(-11.6104790498286,-0.66559499343731,
-1.97639595858999));
#37211=CARTESIAN_POINT('Ctrl Pts',(-11.5292147401353,0.733321543403064,
-2.21002070237282));
#37212=CARTESIAN_POINT('Ctrl Pts',(-11.4057070709201,2.2660422239822,-0.644398977329155));
#37213=CARTESIAN_POINT('Ctrl Pts',(-11.2789769923543,1.77364945549679,1.55095382729707));
#37214=CARTESIAN_POINT('Ctrl Pts',(-11.1522469137885,-0.335801440579385,
2.33175063016555));
#37215=CARTESIAN_POINT('Ctrl Pts',(-11.0494062101355,-1.79909114547032,
1.24084066535289));
#37216=CARTESIAN_POINT('Ctrl Pts',(-10.9888088660044,-1.99263284951445,
0.289271291292402));
#37217=CARTESIAN_POINT('Ctrl Pts',(-10.9704548813952,-1.99173416440345,
0.000704422997178135));
#37218=CARTESIAN_POINT('Origin',(-11.6495,-5.69858952725515E-16,8.58067791224701E-17));
#37219=CARTESIAN_POINT('',(-11.6495,-2.4505,-3.00099698131059E-16));
#37220=CARTESIAN_POINT('Origin',(-11.6495,0.,0.));
#37221=CARTESIAN_POINT('Origin',(-11.6495,0.,0.));
#37222=CARTESIAN_POINT('',(-11.6495,1.16034898466908,-1.62253437445172));
#37223=CARTESIAN_POINT('Ctrl Pts',(-11.6495,1.07765118568552,2.20520362934387));
#37224=CARTESIAN_POINT('Ctrl Pts',(-11.6495,1.13073687254156,2.17343691132479));
#37225=CARTESIAN_POINT('Ctrl Pts',(-11.6495,1.18244979581025,2.13957757514889));
#37226=CARTESIAN_POINT('Ctrl Pts',(-11.6495,1.23264818481424,2.10361864746718));
#37227=CARTESIAN_POINT('Ctrl Pts',(-11.6495,1.30197054661187,2.05396052408779));
#37228=CARTESIAN_POINT('Ctrl Pts',(-11.6495,1.36840639937506,2.00029914630137));
#37229=CARTESIAN_POINT('Ctrl Pts',(-11.6495,1.43178638700421,1.9429963843878));
#37230=CARTESIAN_POINT('Ctrl Pts',(-11.6495,1.46369654011807,1.9141459542298));
#37231=CARTESIAN_POINT('Ctrl Pts',(-11.6495,1.49483142030138,1.88437196977866));
#37232=CARTESIAN_POINT('Ctrl Pts',(-11.6495,1.52516517286246,1.85371813290651));
#37233=CARTESIAN_POINT('Ctrl Pts',(-11.6495,1.5399621404638,1.83876502645716));
#37234=CARTESIAN_POINT('Ctrl Pts',(-11.6495,1.55456843151077,1.82360253561288));
#37235=CARTESIAN_POINT('Ctrl Pts',(-11.6495,1.56898078085552,1.80823563715035));
#37236=CARTESIAN_POINT('Ctrl Pts',(-11.6495,1.58070094654556,1.79573922925633));
#37237=CARTESIAN_POINT('Ctrl Pts',(-11.6495,1.59228652143182,1.78311435458078));
#37238=CARTESIAN_POINT('Ctrl Pts',(-11.6495,1.60373329040506,1.77036734183654));
#37239=CARTESIAN_POINT('Ctrl Pts',(-11.6495,1.66048032516668,1.70717438520439));
#37240=CARTESIAN_POINT('Ctrl Pts',(-11.6495,1.71384375789451,1.64095615253125));
#37241=CARTESIAN_POINT('Ctrl Pts',(-11.6495,1.76365444232725,1.57207081711976));
#37242=CARTESIAN_POINT('Ctrl Pts',(-11.6495,1.80211943702331,1.51887592346563));
#37243=CARTESIAN_POINT('Ctrl Pts',(-11.6495,1.83846500194502,1.46408976223796));
#37244=CARTESIAN_POINT('Ctrl Pts',(-11.6495,1.87259337417673,1.40786969807678));
#37245=CARTESIAN_POINT('Ctrl Pts',(-11.6495,1.88968256071726,1.3797184825061));
#37246=CARTESIAN_POINT('Ctrl Pts',(-11.6495,1.90621554079354,1.35120766875282));
#37247=CARTESIAN_POINT('Ctrl Pts',(-11.6495,1.9221782719748,1.32235676032253));
#37248=CARTESIAN_POINT('Ctrl Pts',(-11.6495,1.93118753982307,1.3060734840609));
#37249=CARTESIAN_POINT('Ctrl Pts',(-11.6495,1.9400170008051,1.28967806812594));
#37250=CARTESIAN_POINT('Ctrl Pts',(-11.6495,1.94865127865783,1.27319896184839));
#37251=CARTESIAN_POINT('Ctrl Pts',(-11.6495,1.98724824363966,1.19953403019175));
#37252=CARTESIAN_POINT('Ctrl Pts',(-11.6495,2.02199988085258,1.12410988628387));
#37253=CARTESIAN_POINT('Ctrl Pts',(-11.6495,2.05274812180369,1.04725942698306));
#37254=CARTESIAN_POINT('Ctrl Pts',(-11.6495,2.08288806559826,0.971929312080035));
#37255=CARTESIAN_POINT('Ctrl Pts',(-11.6495,2.10918158952032,0.895227812752492));
#37256=CARTESIAN_POINT('Ctrl Pts',(-11.6495,2.13143161793832,0.817459396317668));
#37257=CARTESIAN_POINT('Ctrl Pts',(-11.6495,2.15316968868661,0.741480377024631));
#37258=CARTESIAN_POINT('Ctrl Pts',(-11.6495,2.17104828296331,0.66448219410781));
#37259=CARTESIAN_POINT('Ctrl Pts',(-11.6495,2.18483553769043,0.58675257912323));
#37260=CARTESIAN_POINT('Ctrl Pts',(-11.6495,2.18996770971013,0.557818482885722));
#37261=CARTESIAN_POINT('Ctrl Pts',(-11.6495,2.19453248101047,0.528783133929868));
#37262=CARTESIAN_POINT('Ctrl Pts',(-11.6495,2.19851609634267,0.499661837442922));
#37263=CARTESIAN_POINT('Ctrl Pts',(-11.6495,2.20048159642361,0.485293504702629));
#37264=CARTESIAN_POINT('Ctrl Pts',(-11.6495,2.20230560473944,0.470904253929722));
#37265=CARTESIAN_POINT('Ctrl Pts',(-11.6495,2.20398637829912,0.456495955912551));
#37266=CARTESIAN_POINT('Ctrl Pts',(-11.6495,2.20540279415176,0.444353843369362));
#37267=CARTESIAN_POINT('Ctrl Pts',(-11.6495,2.20671636256573,0.43220783876865));
#37268=CARTESIAN_POINT('Ctrl Pts',(-11.6495,2.2079264865813,0.420059244968361));
#37269=CARTESIAN_POINT('Ctrl Pts',(-11.6495,2.21566622029946,0.342359042464759));
#37270=CARTESIAN_POINT('Ctrl Pts',(-11.6495,2.21917890730586,0.264549530424612));
#37271=CARTESIAN_POINT('Ctrl Pts',(-11.6495,2.21828644435235,0.186910890393313));
#37272=CARTESIAN_POINT('Ctrl Pts',(-11.6495,2.21795281039612,0.157886843481426));
#37273=CARTESIAN_POINT('Ctrl Pts',(-11.6495,2.21700303246508,0.128886715398128));
#37274=CARTESIAN_POINT('Ctrl Pts',(-11.6495,2.21542593150821,0.0999254148515203));
#37275=CARTESIAN_POINT('Ctrl Pts',(-11.6495,2.21111957118993,0.0208450015803043));
#37276=CARTESIAN_POINT('Ctrl Pts',(-11.6495,2.20213931188017,-0.0579475015914385));
#37277=CARTESIAN_POINT('Ctrl Pts',(-11.6495,2.18867160105417,-0.136132775928427));
#37278=CARTESIAN_POINT('Ctrl Pts',(-11.6495,2.1755290745819,-0.212430229221862));
#37279=CARTESIAN_POINT('Ctrl Pts',(-11.6495,2.15811243339091,-0.288150111668693));
#37280=CARTESIAN_POINT('Ctrl Pts',(-11.6495,2.13655583598888,-0.362969437792645));
#37281=CARTESIAN_POINT('Ctrl Pts',(-11.6495,2.13202523535206,-0.378694391052281));
#37282=CARTESIAN_POINT('Ctrl Pts',(-11.6495,2.12731033581924,-0.394383242756282));
#37283=CARTESIAN_POINT('Ctrl Pts',(-11.6495,2.1224206951262,-0.410006827745426));
#37284=CARTESIAN_POINT('Ctrl Pts',(-11.6495,2.09918759635712,-0.484242199210638));
#37285=CARTESIAN_POINT('Ctrl Pts',(-11.6495,2.07198357162087,-0.557116646646277));
#37286=CARTESIAN_POINT('Ctrl Pts',(-11.6495,2.04101362673087,-0.628339464180321));
#37287=CARTESIAN_POINT('Ctrl Pts',(-11.6495,2.01006498584023,-0.699513288057304));
#37288=CARTESIAN_POINT('Ctrl Pts',(-11.6495,1.97535493052193,-0.769038579984836));
#37289=CARTESIAN_POINT('Ctrl Pts',(-11.6495,1.93704531624577,-0.83659602647624));
#37290=CARTESIAN_POINT('Ctrl Pts',(-11.6495,1.89937304271498,-0.903029548487702));
#37291=CARTESIAN_POINT('Ctrl Pts',(-11.6495,1.85821928820994,-0.967560808242973));
#37292=CARTESIAN_POINT('Ctrl Pts',(-11.6495,1.81370690330138,-1.02984712465529));
#37293=CARTESIAN_POINT('Ctrl Pts',(-11.6495,1.79661192966788,-1.05376817357198));
#37294=CARTESIAN_POINT('Ctrl Pts',(-11.6495,1.7790213017759,-1.07735764126509));
#37295=CARTESIAN_POINT('Ctrl Pts',(-11.6495,1.76094105430332,-1.10059424300847));
#37296=CARTESIAN_POINT('Ctrl Pts',(-11.6495,1.753322321499,-1.11038578265591));
#37297=CARTESIAN_POINT('Ctrl Pts',(-11.6495,1.74561646654128,-1.12011474214072));
#37298=CARTESIAN_POINT('Ctrl Pts',(-11.6495,1.73783331949158,-1.12976819796877));
#37299=CARTESIAN_POINT('Ctrl Pts',(-11.6495,1.69075783958123,-1.18815602785256));
#37300=CARTESIAN_POINT('Ctrl Pts',(-11.6495,1.64077613345497,-1.2438907292167));
#37301=CARTESIAN_POINT('Ctrl Pts',(-11.6495,1.58804164355534,-1.29668725875532));
#37302=CARTESIAN_POINT('Ctrl Pts',(-11.6495,1.53615976281906,-1.34863017607615));
#37303=CARTESIAN_POINT('Ctrl Pts',(-11.6495,1.48161273193739,-1.39772971703901));
#37304=CARTESIAN_POINT('Ctrl Pts',(-11.6495,1.42451989663264,-1.44367252532997));
#37305=CARTESIAN_POINT('Ctrl Pts',(-11.6495,1.36925371315748,-1.48814542037571));
#37306=CARTESIAN_POINT('Ctrl Pts',(-11.6495,1.31160143729427,-1.52966066226345));
#37307=CARTESIAN_POINT('Ctrl Pts',(-11.6495,1.25165512889375,-1.56788833203711));
#37308=CARTESIAN_POINT('Ctrl Pts',(-11.6495,1.2217859935916,-1.58693583423069));
#37309=CARTESIAN_POINT('Ctrl Pts',(-11.6495,1.19134712145188,-1.60516638714514));
#37310=CARTESIAN_POINT('Ctrl Pts',(-11.6495,1.16034898466911,-1.6225343744517));
#37311=CARTESIAN_POINT('Origin',(-11.6495,0.,0.));
#37312=CARTESIAN_POINT('Origin',(-13.1285451186048,0.,0.));
#37313=CARTESIAN_POINT('Ctrl Pts',(-11.6495,1.16034898466908,-1.62253437445172));
#37314=CARTESIAN_POINT('Ctrl Pts',(-11.6072566404781,1.69867111894511,-1.23755544779991));
#37315=CARTESIAN_POINT('Ctrl Pts',(-11.5227699214342,2.35295738103105,0.103500486870383));
#37316=CARTESIAN_POINT('Ctrl Pts',(-11.3960398428684,1.19148277972948,2.03419922420614));
#37317=CARTESIAN_POINT('Ctrl Pts',(-11.2693097643027,-1.05708502050599,
2.10468425318621));
#37318=CARTESIAN_POINT('Ctrl Pts',(-11.1801448562148,-1.96080296173452,
0.806515742280787));
#37319=CARTESIAN_POINT('Ctrl Pts',(-11.1332233076488,-1.99752919412992,
0.0744005420673237));
#37320=CARTESIAN_POINT('Ctrl Pts',(-11.1285451186048,-1.99700380788516,
0.00135048458759495));
#37321=CARTESIAN_POINT('Ctrl Pts',(-11.9126273851832,1.42545942445495,-1.99324250386965));
#37322=CARTESIAN_POINT('Ctrl Pts',(-11.8703840256612,2.08677457173828,-1.52030561465535));
#37323=CARTESIAN_POINT('Ctrl Pts',(-11.7858973066174,2.89054872150224,0.12714773434053));
#37324=CARTESIAN_POINT('Ctrl Pts',(-11.6591672280516,1.46370650544038,2.49896237569475));
#37325=CARTESIAN_POINT('Ctrl Pts',(-11.5324371494858,-1.29860225228717,
2.58555145378261));
#37326=CARTESIAN_POINT('Ctrl Pts',(-11.4057070709201,-2.87652186863451,
0.318908881767984));
#37327=CARTESIAN_POINT('Ctrl Pts',(-11.2789769923543,-1.83266175101893,
-2.24033061384541));
#37328=CARTESIAN_POINT('Ctrl Pts',(-11.1522469137885,0.881950637603053,
-2.75638944163318));
#37329=CARTESIAN_POINT('Ctrl Pts',(-11.0255168352227,2.79252215107582,-0.760360236683921));
#37330=CARTESIAN_POINT('Ctrl Pts',(-10.898786756657,2.15759767705332,1.9290533008961));
#37331=CARTESIAN_POINT('Ctrl Pts',(-10.7720566780912,-0.4441263759771,2.85988114430123));
#37332=CARTESIAN_POINT('Ctrl Pts',(-10.6453265995254,-2.64099042545161,
1.18383794202982));
#37333=CARTESIAN_POINT('Ctrl Pts',(-10.5185965209596,-2.43044697619487,
-1.57138082209723));
#37334=CARTESIAN_POINT('Ctrl Pts',(-10.3918664423938,-0.00440784228849815,
-2.89417510655402));
#37335=CARTESIAN_POINT('Ctrl Pts',(-10.2651363638281,2.42564737449796,-1.57877333949545));
#37336=CARTESIAN_POINT('Ctrl Pts',(-10.1384062852623,2.64458668371764,1.17577667845936));
#37337=CARTESIAN_POINT('Ctrl Pts',(-10.0116762066965,0.452832795037591,
2.85853574486283));
#37338=CARTESIAN_POINT('Ctrl Pts',(-9.88494612813071,-2.15170392079859,
1.93557684058089));
#37339=CARTESIAN_POINT('Ctrl Pts',(-9.75821604956493,-2.79483906169062,
-0.75177235279057));
#37340=CARTESIAN_POINT('Ctrl Pts',(-9.63148597099916,-0.890317783065174,
-2.75383743537073));
#37341=CARTESIAN_POINT('Ctrl Pts',(-9.50475589243338,1.82577925575169,-2.24562173688547));
#37342=CARTESIAN_POINT('Ctrl Pts',(-9.3780258138676,2.87757364909028,0.309607283664348));
#37343=CARTESIAN_POINT('Ctrl Pts',(-9.25129573530183,1.30629435926593,2.58261141914626));
#37344=CARTESIAN_POINT('Ctrl Pts',(-9.12456565673605,-1.45574726827538,
2.50141693041908));
#37345=CARTESIAN_POINT('Ctrl Pts',(-8.99783557817026,-2.89079164405769,
0.140037208434977));
#37346=CARTESIAN_POINT('Ctrl Pts',(-8.8711054996045,-1.69071338440342,-2.34899446401371));
#37347=CARTESIAN_POINT('Ctrl Pts',(-8.7443754210387,1.05054724076537,-2.69678275833015));
#37348=CARTESIAN_POINT('Ctrl Pts',(-8.61764534247293,2.8341737118076,-0.586298659768404));
#37349=CARTESIAN_POINT('Ctrl Pts',(-8.49091526390716,2.03428804621161,2.05863034353453));
#37350=CARTESIAN_POINT('Ctrl Pts',(-8.36418518534136,-0.619968025159372,
2.8269995393587));
#37351=CARTESIAN_POINT('Ctrl Pts',(-8.23745510677561,-2.709087630006,1.01839626869896));
#37352=CARTESIAN_POINT('Ctrl Pts',(-8.11072502820981,-2.32871824705604,
-1.71853369851118));
#37353=CARTESIAN_POINT('Ctrl Pts',(-7.98399494964404,0.174411582240062,
-2.88892148513446));
#37354=CARTESIAN_POINT('Ctrl Pts',(-7.85726487107826,2.51855523593771,-1.42589139513639));
#37355=CARTESIAN_POINT('Ctrl Pts',(-7.73053479251247,2.5668911234533,1.33692060629286));
#37356=CARTESIAN_POINT('Ctrl Pts',(-7.60380471394671,0.275358306856354,
2.88105268089038));
#37357=CARTESIAN_POINT('Ctrl Pts',(-7.47707463538091,-2.26717942332955,
1.79893974597155));
#37358=CARTESIAN_POINT('Ctrl Pts',(-7.35034455681516,-2.74305287983666,
-0.92301010050071));
#37359=CARTESIAN_POINT('Ctrl Pts',(-7.22361447824936,-0.718476072358019,
-2.80358322163957));
#37360=CARTESIAN_POINT('Ctrl Pts',(-7.0968843996836,1.96103294514159,-2.12852919530761));
#37361=CARTESIAN_POINT('Ctrl Pts',(-6.97015432111781,2.85294778922629,0.486801457636237));
#37362=CARTESIAN_POINT('Ctrl Pts',(-6.84342424255203,1.14423684693021,2.6583846195266));
#37363=CARTESIAN_POINT('Ctrl Pts',(-6.71669416398626,-1.60751170758271,
2.40669750014258));
#37364=CARTESIAN_POINT('Ctrl Pts',(-6.58996408542048,-2.89392100336966,
-0.0388326340083757));
#37365=CARTESIAN_POINT('Ctrl Pts',(-6.4632340068547,-1.54235507453701,-2.44896459167096));
#37366=CARTESIAN_POINT('Ctrl Pts',(-6.33650392828892,1.21515609933081,-2.62672465276953));
#37367=CARTESIAN_POINT('Ctrl Pts',(-6.20977384972314,2.86498268873778,-0.410074310876727));
#37368=CARTESIAN_POINT('Ctrl Pts',(-6.08304377115736,1.90321298956112,2.18038232050574));
#37369=CARTESIAN_POINT('Ctrl Pts',(-5.95631369259159,-0.793444672276071,
2.78329522315633));
#37370=CARTESIAN_POINT('Ctrl Pts',(-5.8295836140258,-2.7668319389872,0.849074654319879));
#37371=CARTESIAN_POINT('Ctrl Pts',(-5.70285353546003,-2.21809296340086,
-1.85912623372372));
#37372=CARTESIAN_POINT('Ctrl Pts',(-5.57612345689425,0.352565158057603,
-2.87262676944498));
#37373=CARTESIAN_POINT('Ctrl Pts',(-5.44939337832847,2.6018398862109,-1.26756299793353));
#37374=CARTESIAN_POINT('Ctrl Pts',(-5.3226632997627,2.47938810549972,1.49295725642586));
#37375=CARTESIAN_POINT('Ctrl Pts',(-5.19593322119691,0.0968316478091236,
2.89256121442409));
#37376=CARTESIAN_POINT('Ctrl Pts',(-5.06920314263115,-2.37399241897732,
1.65542947353446));
#37377=CARTESIAN_POINT('Ctrl Pts',(-4.94247306406535,-2.68078603109511,
-1.09072132219616));
#37378=CARTESIAN_POINT('Ctrl Pts',(-4.81574298549958,-0.543889188532094,
-2.84261698049623));
#37379=CARTESIAN_POINT('Ctrl Pts',(-4.6890129069338,2.08879389097954,-2.00330397798648));
#37380=CARTESIAN_POINT('Ctrl Pts',(-4.56228282836802,2.8174213562132,0.662135672472256));
#37381=CARTESIAN_POINT('Ctrl Pts',(-4.43555274980224,0.977807419436725,
2.7240006236599));
#37382=CARTESIAN_POINT('Ctrl Pts',(-4.30882267123646,-1.75313414650703,
2.30278253675232));
#37383=CARTESIAN_POINT('Ctrl Pts',(-4.18209259267069,-2.88599323592512,
-0.217554106806299));
#37384=CARTESIAN_POINT('Ctrl Pts',(-4.05536251410491,-1.38810371613861,
-2.53957768544997));
#37385=CARTESIAN_POINT('Ctrl Pts',(-3.92863243553913,1.37512207515111,-2.54663032765321));
#37386=CARTESIAN_POINT('Ctrl Pts',(-3.80190235697336,2.8848451063612,-0.232283144877331));
#37387=CARTESIAN_POINT('Ctrl Pts',(-3.67517227840757,1.76486611447052,2.29380346698343));
#37388=CARTESIAN_POINT('Ctrl Pts',(-3.5484421998418,-0.963889716762702,
2.72895646020112));
#37389=CARTESIAN_POINT('Ctrl Pts',(-3.42171212127602,-2.81400470402705,
0.676508885377088));
#37390=CARTESIAN_POINT('Ctrl Pts',(-3.29498204271024,-2.09899276446139,
-1.99261539738261));
#37391=CARTESIAN_POINT('Ctrl Pts',(-3.16825196414446,0.529371649267236,
-2.84535628835101));
#37392=CARTESIAN_POINT('Ctrl Pts',(-3.04152188557868,2.67518339532782,-1.10439148019637));
#37393=CARTESIAN_POINT('Ctrl Pts',(-2.91479180701291,2.38241181420258,1.64328959609923));
#37394=CARTESIAN_POINT('Ctrl Pts',(-2.78806172844712,-0.0820649900061464,
2.89301781990601));
#37395=CARTESIAN_POINT('Ctrl Pts',(-2.66133164988135,-2.47173483038822,
1.50559410984514));
#37396=CARTESIAN_POINT('Ctrl Pts',(-2.53460157131557,-2.60827641565575,
-1.25426508983179));
#37397=CARTESIAN_POINT('Ctrl Pts',(-2.40787149274979,-0.367224183821934,
-2.87078966048055));
#37398=CARTESIAN_POINT('Ctrl Pts',(-2.28114141418401,2.20857390538749,-1.87042446512356));
#37399=CARTESIAN_POINT('Ctrl Pts',(-2.15441133561824,2.77113016932584,0.83493989952818));
#37400=CARTESIAN_POINT('Ctrl Pts',(-2.02768125705246,0.807641816455084,
2.77920890990336));
#37401=CARTESIAN_POINT('Ctrl Pts',(-1.90095117848668,-1.89205788973094,
2.19006874020588));
#37402=CARTESIAN_POINT('Ctrl Pts',(-1.7742210999209,-2.86703920430662,-0.395443708098236));
#37403=CARTESIAN_POINT('Ctrl Pts',(-1.64749102135512,-1.22854758315733,
-2.62048874808283));
#37404=CARTESIAN_POINT('Ctrl Pts',(-1.52076094278934,1.52983188688595,-2.45680348712256));
#37405=CARTESIAN_POINT('Ctrl Pts',(-1.39403086422356,2.893689043194,-0.0536088933736343));
#37406=CARTESIAN_POINT('Ctrl Pts',(-1.26730078565778,1.61976845006142,2.39846885918956));
#37407=CARTESIAN_POINT('Ctrl Pts',(-1.140570707092,-1.13063748919579,2.66417478131471));
#37408=CARTESIAN_POINT('Ctrl Pts',(-1.01384062852623,-2.85045320367203,
0.501388978139588));
#37409=CARTESIAN_POINT('Ctrl Pts',(-0.887110549960449,-1.97182024087482,
-2.11854964337763));
#37410=CARTESIAN_POINT('Ctrl Pts',(-0.760380471394671,0.704055462274761,
-2.80710270335027));
#37411=CARTESIAN_POINT('Ctrl Pts',(-0.633650392828892,2.73849632864145,
-0.937213001936086));
#37412=CARTESIAN_POINT('Ctrl Pts',(-0.506920314263115,2.27596874940147,
1.7877491958748));
#37413=CARTESIAN_POINT('Ctrl Pts',(-0.380190235697335,-0.259952027690717,
2.88164346738145));
#37414=CARTESIAN_POINT('Ctrl Pts',(-0.253460157131559,-2.56137725938084,
1.35151626861576));
#37415=CARTESIAN_POINT('Ctrl Pts',(-0.126730078565777,-2.5230909281715,
-1.41613933844973));
#37416=CARTESIAN_POINT('Ctrl Pts',(-0.0422433595219261,-0.971443343070606,
-2.3921235558411));
#37417=CARTESIAN_POINT('Ctrl Pts',(0.,-0.160158266245241,-2.44526063636442));
#37418=CARTESIAN_POINT('Ctrl Pts',(-11.8249182567888,1.33708927785966,-1.86967312739701));
#37419=CARTESIAN_POINT('Ctrl Pts',(-11.7826748972669,1.95740675414056,-1.42605555903687));
#37420=CARTESIAN_POINT('Ctrl Pts',(-11.698188178223,2.71135160801184,0.119265318517148));
#37421=CARTESIAN_POINT('Ctrl Pts',(-11.5714580996572,1.37296526353675,2.34404132519854));
#37422=CARTESIAN_POINT('Ctrl Pts',(-11.4447280210914,-1.21809650836011,
2.42526238691714));
#37423=CARTESIAN_POINT('Ctrl Pts',(-11.3179979425257,-2.69819433797679,
0.299138396443103));
#37424=CARTESIAN_POINT('Ctrl Pts',(-11.1912678639599,-1.71904744196269,
-2.10144321980882));
#37425=CARTESIAN_POINT('Ctrl Pts',(-11.0645377853941,0.827274856730104,
-2.58550941877739));
#37426=CARTESIAN_POINT('Ctrl Pts',(-10.9378077068283,2.6194021115801,-0.713222349467867));
#37427=CARTESIAN_POINT('Ctrl Pts',(-10.8110776282626,2.02383924118076,1.80946327955578));
#37428=CARTESIAN_POINT('Ctrl Pts',(-10.6843475496968,-0.416593138426741,
2.68258524121815));
#37429=CARTESIAN_POINT('Ctrl Pts',(-10.557617471131,-2.47726446661335,1.11044691406543));
#37430=CARTESIAN_POINT('Ctrl Pts',(-10.4308873925652,-2.27977347971104,
-1.47396440236374));
#37431=CARTESIAN_POINT('Ctrl Pts',(-10.3041573139994,-0.00413458184871249,
-2.71475317840167));
#37432=CARTESIAN_POINT('Ctrl Pts',(-10.1774272354337,2.27527142524578,-1.48089862692316));
#37433=CARTESIAN_POINT('Ctrl Pts',(-10.0506971568679,2.4806377779019,1.10288540168486));
#37434=CARTESIAN_POINT('Ctrl Pts',(-9.9239670783021,0.424759810430573,2.68132324867549));
#37435=CARTESIAN_POINT('Ctrl Pts',(-9.79723699973633,-2.0183108633404,1.81558239793723));
#37436=CARTESIAN_POINT('Ctrl Pts',(-9.67050692117055,-2.62157538728873,
-0.705166864144143));
#37437=CARTESIAN_POINT('Ctrl Pts',(-9.54377684260478,-0.835123288114206,
-2.58311562197616));
#37438=CARTESIAN_POINT('Ctrl Pts',(-9.41704676403898,1.71259162114532,-2.10640632416894));
#37439=CARTESIAN_POINT('Ctrl Pts',(-9.29031668547322,2.69918091419632,0.290413443015511));
#37440=CARTESIAN_POINT('Ctrl Pts',(-9.16358660690742,1.22531174969842,2.42250461723157));
#37441=CARTESIAN_POINT('Ctrl Pts',(-9.03685652834166,-1.36549945252126,
2.346343711887));
#37442=CARTESIAN_POINT('Ctrl Pts',(-8.91012644977587,-2.71157947078975,
0.131355720610133));
#37443=CARTESIAN_POINT('Ctrl Pts',(-8.7833963712101,-1.58589904380056,-2.20337054685746));
#37444=CARTESIAN_POINT('Ctrl Pts',(-8.65666629264431,0.985419456642577,
-2.52959800119093));
#37445=CARTESIAN_POINT('Ctrl Pts',(-8.52993621407854,2.65847151917259,-0.549951572209463));
#37446=CARTESIAN_POINT('Ctrl Pts',(-8.40320613551276,1.90817408619515,1.93100730346573));
#37447=CARTESIAN_POINT('Ctrl Pts',(-8.276476056947,-0.581533633883264,2.65174210345273));
#37448=CARTESIAN_POINT('Ctrl Pts',(-8.14974597838119,-2.54114004279588,
0.955261656788515));
#37449=CARTESIAN_POINT('Ctrl Pts',(-8.02301589981544,-2.18435133675258,
-1.61199466115875));
#37450=CARTESIAN_POINT('Ctrl Pts',(-7.89628582124963,0.163599084300075,
-2.70982525078093));
#37451=CARTESIAN_POINT('Ctrl Pts',(-7.76955574268389,2.36241954270795,-1.33749446888549));
#37452=CARTESIAN_POINT('Ctrl Pts',(-7.64282566411808,2.40775888792125,1.25403934854711));
#37453=CARTESIAN_POINT('Ctrl Pts',(-7.51609558555232,0.258287702442303,
2.70244426637418));
#37454=CARTESIAN_POINT('Ctrl Pts',(-7.38936550698653,-2.12662756014756,
1.6874160039833));
#37455=CARTESIAN_POINT('Ctrl Pts',(-7.26263542842076,-2.57299964580475,
-0.86578887309092));
#37456=CARTESIAN_POINT('Ctrl Pts',(-7.13590534985498,-0.673934758343563,
-2.62977746046671));
#37457=CARTESIAN_POINT('Ctrl Pts',(-7.0091752712892,1.83946037291168,-1.99657283527748));
#37458=CARTESIAN_POINT('Ctrl Pts',(-6.88244519272341,2.67608171360365,0.456622614635815));
#37459=CARTESIAN_POINT('Ctrl Pts',(-6.75571511415765,1.07330085522939,2.49358032239687));
#37460=CARTESIAN_POINT('Ctrl Pts',(-6.62898503559186,-1.50785538428396,
2.25749633225983));
#37461=CARTESIAN_POINT('Ctrl Pts',(-6.50225495702609,-2.71451482812846,
-0.0364252378376332));
#37462=CARTESIAN_POINT('Ctrl Pts',(-6.3755248784603,-1.44673808137638,-2.29714311133987));
#37463=CARTESIAN_POINT('Ctrl Pts',(-6.24879479989453,1.13982352879828,-2.46388308839495));
#37464=CARTESIAN_POINT('Ctrl Pts',(-6.12206472132875,2.68737051973931,-0.38465210218705));
#37465=CARTESIAN_POINT('Ctrl Pts',(-5.99533464276298,1.78522491637979,2.04521137000987));
#37466=CARTESIAN_POINT('Ctrl Pts',(-5.8686045641972,-0.744255743569043,
2.61074719922196));
#37467=CARTESIAN_POINT('Ctrl Pts',(-5.74187448563141,-2.59530454237517,
0.796436992114019));
#37468=CARTESIAN_POINT('Ctrl Pts',(-5.61514440706564,-2.08058417362054,
-1.74387128153443));
#37469=CARTESIAN_POINT('Ctrl Pts',(-5.48841432849986,0.330708180463282,
-2.69454071215402));
#37470=CARTESIAN_POINT('Ctrl Pts',(-5.36168424993407,2.44054103180832,-1.18898150622322));
#37471=CARTESIAN_POINT('Ctrl Pts',(-5.23495417136831,2.32568054526282,1.40040263905308));
#37472=CARTESIAN_POINT('Ctrl Pts',(-5.10822409280252,0.0908286520274319,
2.71323933814391));
#37473=CARTESIAN_POINT('Ctrl Pts',(-4.98149401423675,-2.22681877483003,
1.55280252902471));
#37474=CARTESIAN_POINT('Ctrl Pts',(-4.85476393567096,-2.51459297747725,
-1.02310298000874));
#37475=CARTESIAN_POINT('Ctrl Pts',(-4.72803385710519,-0.510171240130598,
-2.66639135458844));
#37476=CARTESIAN_POINT('Ctrl Pts',(-4.60130377853941,1.95930088740016,-1.87911084896963));
#37477=CARTESIAN_POINT('Ctrl Pts',(-4.47457369997363,2.64275771163805,0.621087133707496));
#37478=CARTESIAN_POINT('Ctrl Pts',(-4.34784362140786,0.917189078770414,
2.55512851807153));
#37479=CARTESIAN_POINT('Ctrl Pts',(-4.22111354284207,-1.64445008376195,
2.16002348878593));
#37480=CARTESIAN_POINT('Ctrl Pts',(-4.0943834642763,-2.7070785358948,-0.20406702469015));
#37481=CARTESIAN_POINT('Ctrl Pts',(-3.96765338571052,-1.3020494049599,-2.38213872331384));
#37482=CARTESIAN_POINT('Ctrl Pts',(-3.84092330714474,1.28987254978213,-2.3887541429524));
#37483=CARTESIAN_POINT('Ctrl Pts',(-3.71419322857896,2.70600158364826,-0.21788294855305));
#37484=CARTESIAN_POINT('Ctrl Pts',(-3.58746315001318,1.65545473833367,2.15160106882283));
#37485=CARTESIAN_POINT('Ctrl Pts',(-3.4607330714474,-0.904134192255527,
2.55977712173459));
#37486=CARTESIAN_POINT('Ctrl Pts',(-3.33400299288163,-2.63955287190295,
0.634569291483229));
#37487=CARTESIAN_POINT('Ctrl Pts',(-3.20727291431585,-1.96886749038081,
-1.86908489784414));
#37488=CARTESIAN_POINT('Ctrl Pts',(-3.08054283575007,0.496553703384974,
-2.66896084137883));
#37489=CARTESIAN_POINT('Ctrl Pts',(-2.95381275718429,2.50933767235691,-1.03592566817167));
#37490=CARTESIAN_POINT('Ctrl Pts',(-2.82708267861852,2.23471621679757,1.54141525298257));
#37491=CARTESIAN_POINT('Ctrl Pts',(-2.70035260005273,-0.0769774406359214,
2.7136676367567));
#37492=CARTESIAN_POINT('Ctrl Pts',(-2.57362252148696,-2.31850172844312,
1.41225608147515));
#37493=CARTESIAN_POINT('Ctrl Pts',(-2.44689244292118,-2.44657853407578,
-1.17650799064241));
#37494=CARTESIAN_POINT('Ctrl Pts',(-2.3201623643554,-0.344458432372982,
-2.69281749319986));
#37495=CARTESIAN_POINT('Ctrl Pts',(-2.19343228578962,2.07165524152565,-1.75446908867248));
#37496=CARTESIAN_POINT('Ctrl Pts',(-2.06670220722384,2.59933630757378,0.783178509443182));
#37497=CARTESIAN_POINT('Ctrl Pts',(-1.93997212865807,0.757572747850102,
2.60691421348924));
#37498=CARTESIAN_POINT('Ctrl Pts',(-1.81324205009229,-1.77476136749129,
2.05429728834587));
#37499=CARTESIAN_POINT('Ctrl Pts',(-1.68651197152651,-2.68929954337174,
-0.370928511204314));
#37500=CARTESIAN_POINT('Ctrl Pts',(-1.55978189296073,-1.15238481895627,
-2.45803377332412));
#37501=CARTESIAN_POINT('Ctrl Pts',(-1.43305181439495,1.43499125810976,-2.30449604112431));
#37502=CARTESIAN_POINT('Ctrl Pts',(-1.30632173582917,2.71429724812692,-0.0502854555507226));
#37503=CARTESIAN_POINT('Ctrl Pts',(-1.17959165726339,1.51935228042046,2.24977781891539));
#37504=CARTESIAN_POINT('Ctrl Pts',(-1.05286157869761,-1.0605445781299,2.49901152802161));
#37505=CARTESIAN_POINT('Ctrl Pts',(-0.926131500131838,-2.67374177776255,
0.470305794192473));
#37506=CARTESIAN_POINT('Ctrl Pts',(-0.799401421566061,-1.8495789194059,
-1.98721195719532));
#37507=CARTESIAN_POINT('Ctrl Pts',(-0.67267134300028,0.660408141737237,
-2.63307875489731));
#37508=CARTESIAN_POINT('Ctrl Pts',(-0.545941264434503,2.56872557413171,
-0.879111277712124));
#37509=CARTESIAN_POINT('Ctrl Pts',(-0.419211185868724,2.13487199941306,
1.67691920253741));
#37510=CARTESIAN_POINT('Ctrl Pts',(-0.292481107302946,-0.243836522471383,
2.70299842755841));
#37511=CARTESIAN_POINT('Ctrl Pts',(-0.165751028737168,-2.4025868511699,
1.26773016517814));
#37512=CARTESIAN_POINT('Ctrl Pts',(-0.0390209501713873,-2.36667404855317,
-1.32834698267222));
#37513=CARTESIAN_POINT('Ctrl Pts',(0.0454657688724642,-0.91121953791458,
-2.24382588725992));
#37514=CARTESIAN_POINT('Ctrl Pts',(0.0877091283943902,-0.150229390527176,
-2.29366877959735));
#37515=CARTESIAN_POINT('Ctrl Pts',(-11.7372091283944,1.24871913126437,-1.74610375092436));
#37516=CARTESIAN_POINT('Ctrl Pts',(-11.6949657688725,1.82803893654284,-1.33180550341839));
#37517=CARTESIAN_POINT('Ctrl Pts',(-11.6104790498286,2.53215449452145,0.111382902693765));
#37518=CARTESIAN_POINT('Ctrl Pts',(-11.4837489712628,1.28222402163311,2.18912027470234));
#37519=CARTESIAN_POINT('Ctrl Pts',(-11.3570188926971,-1.13759076443305,
2.26497332005167));
#37520=CARTESIAN_POINT('Ctrl Pts',(-11.2302888141313,-2.51986680731908,
0.279367911118224));
#37521=CARTESIAN_POINT('Ctrl Pts',(-11.1035587355655,-1.60543313290645,
-1.96255582577224));
#37522=CARTESIAN_POINT('Ctrl Pts',(-10.9768286569997,0.772599075857153,
-2.41462939592159));
#37523=CARTESIAN_POINT('Ctrl Pts',(-10.850098578434,2.44628207208438,-0.666084462251818));
#37524=CARTESIAN_POINT('Ctrl Pts',(-10.7233684998682,1.8900808053082,1.68987325821547));
#37525=CARTESIAN_POINT('Ctrl Pts',(-10.5966384213024,-0.389059900876383,
2.50528933813506));
#37526=CARTESIAN_POINT('Ctrl Pts',(-10.4699083427366,-2.31353850777508,
1.03705588610104));
#37527=CARTESIAN_POINT('Ctrl Pts',(-10.3431782641708,-2.12909998322721,
-1.37654798263025));
#37528=CARTESIAN_POINT('Ctrl Pts',(-10.2164481856051,-0.00386132140892683,
-2.53533125024933));
#37529=CARTESIAN_POINT('Ctrl Pts',(-10.0897181070393,2.1248954759936,-1.38302391435088));
#37530=CARTESIAN_POINT('Ctrl Pts',(-9.96298802847351,2.31668887208617,1.02999412491035));
#37531=CARTESIAN_POINT('Ctrl Pts',(-9.8362579499077,0.396686825823557,2.50411075248815));
#37532=CARTESIAN_POINT('Ctrl Pts',(-9.70952787134194,-1.88491780588221,
1.69558795529358));
#37533=CARTESIAN_POINT('Ctrl Pts',(-9.58279779277616,-2.44831171288684,
-0.658561375497717));
#37534=CARTESIAN_POINT('Ctrl Pts',(-9.45606771421038,-0.779928793163236,
-2.41239380858159));
#37535=CARTESIAN_POINT('Ctrl Pts',(-9.32933763564459,1.59940398653894,-1.9671909114524));
#37536=CARTESIAN_POINT('Ctrl Pts',(-9.20260755707883,2.52078817930237,0.271219602366674));
#37537=CARTESIAN_POINT('Ctrl Pts',(-9.07587747851304,1.14432914013092,2.26239781531688));
#37538=CARTESIAN_POINT('Ctrl Pts',(-8.94914739994727,-1.27525163676714,
2.19127049335493));
#37539=CARTESIAN_POINT('Ctrl Pts',(-8.82241732138148,-2.5323672975218,0.122674232785287));
#37540=CARTESIAN_POINT('Ctrl Pts',(-8.69568724281572,-1.4810847031977,-2.05774662970121));
#37541=CARTESIAN_POINT('Ctrl Pts',(-8.56895716424991,0.920291672519785,
-2.36241324405171));
#37542=CARTESIAN_POINT('Ctrl Pts',(-8.44222708568416,2.48276932653758,-0.513604484650522));
#37543=CARTESIAN_POINT('Ctrl Pts',(-8.31549700711837,1.78206012617869,1.80338426339693));
#37544=CARTESIAN_POINT('Ctrl Pts',(-8.18876692855259,-0.543099242607164,
2.47648466754675));
#37545=CARTESIAN_POINT('Ctrl Pts',(-8.06203684998681,-2.37319245558576,
0.892127044878068));
#37546=CARTESIAN_POINT('Ctrl Pts',(-7.93530677142103,-2.03998442644912,
-1.50545562380632));
#37547=CARTESIAN_POINT('Ctrl Pts',(-7.80857669285526,0.152786586360089,
-2.53072901642739));
#37548=CARTESIAN_POINT('Ctrl Pts',(-7.68184661428948,2.20628384947819,-1.24909754263459));
#37549=CARTESIAN_POINT('Ctrl Pts',(-7.55511653572371,2.2486266523892,1.17115809080136));
#37550=CARTESIAN_POINT('Ctrl Pts',(-7.42838645715792,0.241217098028255,
2.52383585185799));
#37551=CARTESIAN_POINT('Ctrl Pts',(-7.30165637859215,-1.98607569696558,
1.57589226199505));
#37552=CARTESIAN_POINT('Ctrl Pts',(-7.17492630002637,-2.40294641177284,
-0.808567645681122));
#37553=CARTESIAN_POINT('Ctrl Pts',(-7.04819622146058,-0.629393444329111,
-2.45597169929387));
#37554=CARTESIAN_POINT('Ctrl Pts',(-6.92146614289482,1.71788780068177,-1.86461647524734));
#37555=CARTESIAN_POINT('Ctrl Pts',(-6.79473606432902,2.49921563798099,0.426443771635388));
#37556=CARTESIAN_POINT('Ctrl Pts',(-6.66800598576326,1.00236486352858,2.32877602526715));
#37557=CARTESIAN_POINT('Ctrl Pts',(-6.54127590719748,-1.40819906098522,
2.10829516437708));
#37558=CARTESIAN_POINT('Ctrl Pts',(-6.41454582863168,-2.53510865288725,
-0.0340178416668884));
#37559=CARTESIAN_POINT('Ctrl Pts',(-6.28781575006593,-1.35112108821576,
-2.14532163100879));
#37560=CARTESIAN_POINT('Ctrl Pts',(-6.16108567150013,1.06449095826574,-2.30104152402036));
#37561=CARTESIAN_POINT('Ctrl Pts',(-6.03435559293437,2.50975835074084,-0.359229893497372));
#37562=CARTESIAN_POINT('Ctrl Pts',(-5.90762551436857,1.66723684319845,1.910040419514));
#37563=CARTESIAN_POINT('Ctrl Pts',(-5.78089543580281,-0.695066814862014,
2.43819917528759));
#37564=CARTESIAN_POINT('Ctrl Pts',(-5.65416535723702,-2.42377714576313,
0.743799329908159));
#37565=CARTESIAN_POINT('Ctrl Pts',(-5.52743527867125,-1.94307538384022,
-1.62861632934515));
#37566=CARTESIAN_POINT('Ctrl Pts',(-5.40070520010547,0.308851202868963,
-2.51645465486305));
#37567=CARTESIAN_POINT('Ctrl Pts',(-5.27397512153969,2.27924217740573,-1.11040001451292));
#37568=CARTESIAN_POINT('Ctrl Pts',(-5.14724504297392,2.17197298502593,1.3078480216803));
#37569=CARTESIAN_POINT('Ctrl Pts',(-5.02051496440813,0.0848256562457381,
2.53391746186373));
#37570=CARTESIAN_POINT('Ctrl Pts',(-4.89378488584236,-2.07964513068273,
1.45017558451496));
#37571=CARTESIAN_POINT('Ctrl Pts',(-4.76705480727658,-2.3483999238594,-0.955484637821318));
#37572=CARTESIAN_POINT('Ctrl Pts',(-4.6403247287108,-0.476453291729102,
-2.49016572868064));
#37573=CARTESIAN_POINT('Ctrl Pts',(-4.51359465014502,1.82980788382077,-1.75491771995277));
#37574=CARTESIAN_POINT('Ctrl Pts',(-4.38686457157924,2.46809406706291,0.58003859494274));
#37575=CARTESIAN_POINT('Ctrl Pts',(-4.26013449301346,0.856570738104105,
2.38625641248314));
#37576=CARTESIAN_POINT('Ctrl Pts',(-4.13340441444769,-1.53576602101686,
2.01726444081954));
#37577=CARTESIAN_POINT('Ctrl Pts',(-4.0066743358819,-2.52816383586448,-0.190579942574003));
#37578=CARTESIAN_POINT('Ctrl Pts',(-3.87994425731613,-1.2159950937812,-2.22469976117771));
#37579=CARTESIAN_POINT('Ctrl Pts',(-3.75321417875035,1.20462302441316,-2.23087795825159));
#37580=CARTESIAN_POINT('Ctrl Pts',(-3.62648410018457,2.52715806093534,-0.203482752228769));
#37581=CARTESIAN_POINT('Ctrl Pts',(-3.49975402161879,1.54604336219683,2.00939867066223));
#37582=CARTESIAN_POINT('Ctrl Pts',(-3.37302394305301,-0.84437866774835,
2.39059778326806));
#37583=CARTESIAN_POINT('Ctrl Pts',(-3.24629386448724,-2.46510103977886,
0.592629697589368));
#37584=CARTESIAN_POINT('Ctrl Pts',(-3.11956378592146,-1.83874221630024,
-1.74555439830567));
#37585=CARTESIAN_POINT('Ctrl Pts',(-2.99283370735568,0.463735757502715,
-2.49256539440665));
#37586=CARTESIAN_POINT('Ctrl Pts',(-2.8661036287899,2.343491949386,-0.967459856146969));
#37587=CARTESIAN_POINT('Ctrl Pts',(-2.73937355022413,2.08702061939257,1.43954090986591));
#37588=CARTESIAN_POINT('Ctrl Pts',(-2.61264347165834,-0.0718898912657027,
2.53431745360739));
#37589=CARTESIAN_POINT('Ctrl Pts',(-2.48591339309257,-2.16526862649802,
1.31891805310516));
#37590=CARTESIAN_POINT('Ctrl Pts',(-2.35918331452679,-2.28488065249581,
-1.09875089145302));
#37591=CARTESIAN_POINT('Ctrl Pts',(-2.23245323596101,-0.321692680924034,
-2.51484532591917));
#37592=CARTESIAN_POINT('Ctrl Pts',(-2.10572315739523,1.93473657766382,-1.63851371222139));
#37593=CARTESIAN_POINT('Ctrl Pts',(-1.97899307882946,2.42754244582172,0.731417119358184));
#37594=CARTESIAN_POINT('Ctrl Pts',(-1.85226300026367,0.707503679245126,
2.43461951707511));
#37595=CARTESIAN_POINT('Ctrl Pts',(-1.7255329216979,-1.65746484525164,1.91852583648585));
#37596=CARTESIAN_POINT('Ctrl Pts',(-1.59880284313211,-2.51155988243686,
-0.346413314310394));
#37597=CARTESIAN_POINT('Ctrl Pts',(-1.47207276456634,-1.07622205475522,
-2.2955787985654));
#37598=CARTESIAN_POINT('Ctrl Pts',(-1.34534268600056,1.34015062933357,-2.15218859512606));
#37599=CARTESIAN_POINT('Ctrl Pts',(-1.21861260743479,2.53490545305983,-0.0469620177278084));
#37600=CARTESIAN_POINT('Ctrl Pts',(-1.091882528869,1.41893611077949,2.10108677864122));
#37601=CARTESIAN_POINT('Ctrl Pts',(-0.965152450303225,-0.99045166706401,
2.33384827472851));
#37602=CARTESIAN_POINT('Ctrl Pts',(-0.838422371737447,-2.49703035185308,
0.439222610245357));
#37603=CARTESIAN_POINT('Ctrl Pts',(-0.711692293171671,-1.72733759793698,
-1.855874271013));
#37604=CARTESIAN_POINT('Ctrl Pts',(-0.58496221460589,0.61676082119971,-2.45905480644435));
#37605=CARTESIAN_POINT('Ctrl Pts',(-0.458232136040112,2.39895481962198,
-0.821009553488159));
#37606=CARTESIAN_POINT('Ctrl Pts',(-0.331502057474334,1.99377524942465,
1.56608920920002));
#37607=CARTESIAN_POINT('Ctrl Pts',(-0.204771978908555,-0.227721017252045,
2.52435338773536));
#37608=CARTESIAN_POINT('Ctrl Pts',(-0.0780419003427782,-2.24379644295895,
1.18394406174051));
#37609=CARTESIAN_POINT('Ctrl Pts',(0.048688178223003,-2.21025716893482,
-1.24055462689471));
#37610=CARTESIAN_POINT('Ctrl Pts',(0.133174897266854,-0.850995732758557,
-2.09552821867874));
#37611=CARTESIAN_POINT('Ctrl Pts',(0.17541825678878,-0.140300514809111,
-2.14207692283029));
#37612=CARTESIAN_POINT('Ctrl Pts',(-11.6495,1.16034898466908,-1.62253437445172));
#37613=CARTESIAN_POINT('Ctrl Pts',(-11.6072566404781,1.69867111894511,-1.23755544779991));
#37614=CARTESIAN_POINT('Ctrl Pts',(-11.5227699214342,2.35295738103105,0.103500486870383));
#37615=CARTESIAN_POINT('Ctrl Pts',(-11.3960398428684,1.19148277972948,2.03419922420614));
#37616=CARTESIAN_POINT('Ctrl Pts',(-11.2693097643027,-1.05708502050599,
2.10468425318621));
#37617=CARTESIAN_POINT('Ctrl Pts',(-11.1425796857369,-2.34153927666138,
0.259597425793341));
#37618=CARTESIAN_POINT('Ctrl Pts',(-11.0158496071711,-1.49181882385021,
-1.82366843173565));
#37619=CARTESIAN_POINT('Ctrl Pts',(-10.8891195286053,0.717923294984202,
-2.24374937306581));
#37620=CARTESIAN_POINT('Ctrl Pts',(-10.7623894500395,2.27316203258867,-0.618946575035767));
#37621=CARTESIAN_POINT('Ctrl Pts',(-10.6356593714738,1.75632236943564,1.57028323687515));
#37622=CARTESIAN_POINT('Ctrl Pts',(-10.508929292908,-0.361526663326025,
2.32799343505198));
#37623=CARTESIAN_POINT('Ctrl Pts',(-10.3821992143422,-2.14981254893681,
0.963664858136657));
#37624=CARTESIAN_POINT('Ctrl Pts',(-10.2554691357764,-1.97842648674338,
-1.27913156289677));
#37625=CARTESIAN_POINT('Ctrl Pts',(-10.1287390572107,-0.00358806096914,
-2.35590932209698));
#37626=CARTESIAN_POINT('Ctrl Pts',(-10.0020089786449,1.97451952674142,-1.2851492017786));
#37627=CARTESIAN_POINT('Ctrl Pts',(-9.8752789000791,2.15273996627044,0.957102848135853));
#37628=CARTESIAN_POINT('Ctrl Pts',(-9.74854882151332,0.368613841216539,
2.32689825630081));
#37629=CARTESIAN_POINT('Ctrl Pts',(-9.62181874294755,-1.75152474842402,
1.57559351264993));
#37630=CARTESIAN_POINT('Ctrl Pts',(-9.49508866438176,-2.27504803848494,
-0.611955886851293));
#37631=CARTESIAN_POINT('Ctrl Pts',(-9.368358585816,-0.724734298212267,-2.24167199518702));
#37632=CARTESIAN_POINT('Ctrl Pts',(-9.2416285072502,1.48621635193257,-1.82797549873587));
#37633=CARTESIAN_POINT('Ctrl Pts',(-9.11489842868443,2.34239544440841,0.252025761717839));
#37634=CARTESIAN_POINT('Ctrl Pts',(-8.98816835011866,1.06334653056341,2.10229101340218));
#37635=CARTESIAN_POINT('Ctrl Pts',(-8.86143827155287,-1.18500382101302,
2.03619727482286));
#37636=CARTESIAN_POINT('Ctrl Pts',(-8.7347081929871,-2.35315512425386,0.113992744960442));
#37637=CARTESIAN_POINT('Ctrl Pts',(-8.60797811442132,-1.37627036259484,
-1.91212271254496));
#37638=CARTESIAN_POINT('Ctrl Pts',(-8.48124803585554,0.85516388839699,-2.19522848691248));
#37639=CARTESIAN_POINT('Ctrl Pts',(-8.35451795728975,2.30706713390257,-0.47725739709158));
#37640=CARTESIAN_POINT('Ctrl Pts',(-8.22778787872399,1.65594616616223,1.67576122332812));
#37641=CARTESIAN_POINT('Ctrl Pts',(-8.10105780015819,-0.504664851331058,
2.30122723164079));
#37642=CARTESIAN_POINT('Ctrl Pts',(-7.97432772159243,-2.20524486837564,
0.828992432967621));
#37643=CARTESIAN_POINT('Ctrl Pts',(-7.84759764302665,-1.89561751614567,
-1.39891658645389));
#37644=CARTESIAN_POINT('Ctrl Pts',(-7.72086756446086,0.141974088420104,
-2.35163278207385));
#37645=CARTESIAN_POINT('Ctrl Pts',(-7.5941374858951,2.05014815624844,-1.16070061638369));
#37646=CARTESIAN_POINT('Ctrl Pts',(-7.46740740732931,2.08949441685714,1.08827683305561));
#37647=CARTESIAN_POINT('Ctrl Pts',(-7.34067732876354,0.224146493614207,
2.3452274373418));
#37648=CARTESIAN_POINT('Ctrl Pts',(-7.21394725019775,-1.84552383378359,
1.4643685200068));
#37649=CARTESIAN_POINT('Ctrl Pts',(-7.08721717163198,-2.23289317774092,
-0.75134641827133));
#37650=CARTESIAN_POINT('Ctrl Pts',(-6.96048709306619,-0.584852130314656,
-2.28216593812101));
#37651=CARTESIAN_POINT('Ctrl Pts',(-6.83375701450043,1.59631522845185,-1.73266011521722));
#37652=CARTESIAN_POINT('Ctrl Pts',(-6.70702693593464,2.32234956235835,0.396264928634968));
#37653=CARTESIAN_POINT('Ctrl Pts',(-6.58029685736886,0.931428871827763,
2.16397172813741));
#37654=CARTESIAN_POINT('Ctrl Pts',(-6.45356677880309,-1.30854273768647,
1.95909399649433));
#37655=CARTESIAN_POINT('Ctrl Pts',(-6.3268367002373,-2.35570247764605,-0.03161044549615));
#37656=CARTESIAN_POINT('Ctrl Pts',(-6.20010662167154,-1.25550409505514,
-1.9935001506777));
#37657=CARTESIAN_POINT('Ctrl Pts',(-6.07337654310573,0.989158387733211,
-2.13819995964578));
#37658=CARTESIAN_POINT('Ctrl Pts',(-5.94664646453999,2.33214618174238,-0.333807684807691));
#37659=CARTESIAN_POINT('Ctrl Pts',(-5.81991638597417,1.54924877001712,1.77486946901812));
#37660=CARTESIAN_POINT('Ctrl Pts',(-5.69318630740843,-0.645877886154986,
2.26565115135322));
#37661=CARTESIAN_POINT('Ctrl Pts',(-5.56645622884262,-2.25224974915109,
0.691161667702299));
#37662=CARTESIAN_POINT('Ctrl Pts',(-5.43972615027687,-1.8055665940599,-1.51336137715587));
#37663=CARTESIAN_POINT('Ctrl Pts',(-5.31299607171107,0.286994225274642,
-2.33836859757207));
#37664=CARTESIAN_POINT('Ctrl Pts',(-5.18626599314531,2.11794332300315,-1.03181852280261));
#37665=CARTESIAN_POINT('Ctrl Pts',(-5.05953591457952,2.01826542478903,1.21529340430752));
#37666=CARTESIAN_POINT('Ctrl Pts',(-4.93280583601374,0.0788226604640474,
2.35459558558354));
#37667=CARTESIAN_POINT('Ctrl Pts',(-4.80607575744796,-1.93247148653543,
1.34754864000521));
#37668=CARTESIAN_POINT('Ctrl Pts',(-4.67934567888219,-2.18220687024155,
-0.887866295633901));
#37669=CARTESIAN_POINT('Ctrl Pts',(-4.55261560031641,-0.442735343327605,
-2.31394010277285));
#37670=CARTESIAN_POINT('Ctrl Pts',(-4.42588552175063,1.70031488024139,-1.63072459093592));
#37671=CARTESIAN_POINT('Ctrl Pts',(-4.29915544318485,2.29343042248776,0.538990056177979));
#37672=CARTESIAN_POINT('Ctrl Pts',(-4.17242536461907,0.795952397437793,
2.21738430689477));
#37673=CARTESIAN_POINT('Ctrl Pts',(-4.0456952860533,-1.42708195827177,1.87450539285314));
#37674=CARTESIAN_POINT('Ctrl Pts',(-3.91896520748751,-2.34924913583417,
-0.177092860457853));
#37675=CARTESIAN_POINT('Ctrl Pts',(-3.79223512892175,-1.12994078260249,
-2.06726079904157));
#37676=CARTESIAN_POINT('Ctrl Pts',(-3.66550505035595,1.11937349904418,-2.07300177355078));
#37677=CARTESIAN_POINT('Ctrl Pts',(-3.53877497179019,2.34831453822241,-0.189082555904491));
#37678=CARTESIAN_POINT('Ctrl Pts',(-3.4120448932244,1.43663198605998,1.86719627250164));
#37679=CARTESIAN_POINT('Ctrl Pts',(-3.28531481465863,-0.784623143241175,
2.22141844480153));
#37680=CARTESIAN_POINT('Ctrl Pts',(-3.15858473609284,-2.29064920765476,
0.55069010369551));
#37681=CARTESIAN_POINT('Ctrl Pts',(-3.03185465752707,-1.70861694221966,
-1.6220238987672));
#37682=CARTESIAN_POINT('Ctrl Pts',(-2.90512457896129,0.430917811620456,
-2.31616994743447));
#37683=CARTESIAN_POINT('Ctrl Pts',(-2.77839450039551,2.1776462264151,-0.898994044122268));
#37684=CARTESIAN_POINT('Ctrl Pts',(-2.65166442182973,1.93932502198757,1.33766656674925));
#37685=CARTESIAN_POINT('Ctrl Pts',(-2.52493434326395,-0.066802341895476,
2.35496727045807));
#37686=CARTESIAN_POINT('Ctrl Pts',(-2.39820426469818,-2.01203552455293,
1.22558002473516));
#37687=CARTESIAN_POINT('Ctrl Pts',(-2.2714741861324,-2.12318277091584,-1.02099379226364));
#37688=CARTESIAN_POINT('Ctrl Pts',(-2.14474410756662,-0.298926929475087,
-2.33687315863848));
#37689=CARTESIAN_POINT('Ctrl Pts',(-2.01801402900084,1.79781791380199,-1.52255833577031));
#37690=CARTESIAN_POINT('Ctrl Pts',(-1.89128395043506,2.25574858406966,0.679655729273182));
#37691=CARTESIAN_POINT('Ctrl Pts',(-1.76455387186929,0.657434610640146,
2.26232482066099));
#37692=CARTESIAN_POINT('Ctrl Pts',(-1.6378237933035,-1.54016832301198,1.78275438462583));
#37693=CARTESIAN_POINT('Ctrl Pts',(-1.51109371473773,-2.33382022150199,
-0.321898117416469));
#37694=CARTESIAN_POINT('Ctrl Pts',(-1.38436363617195,-1.00005929055416,
-2.13312382380668));
#37695=CARTESIAN_POINT('Ctrl Pts',(-1.25763355760617,1.24531000055737,-1.9998811491278));
#37696=CARTESIAN_POINT('Ctrl Pts',(-1.13090347904039,2.35551365799275,-0.0436385799048972));
#37697=CARTESIAN_POINT('Ctrl Pts',(-1.00417340047461,1.31851994113852,1.95239573836704));
#37698=CARTESIAN_POINT('Ctrl Pts',(-0.877443321908835,-0.920358755998121,
2.16868502143541));
#37699=CARTESIAN_POINT('Ctrl Pts',(-0.750713243343058,-2.32031892594361,
0.408139426298241));
#37700=CARTESIAN_POINT('Ctrl Pts',(-0.62398316477728,-1.60509627646806,
-1.72453658483069));
#37701=CARTESIAN_POINT('Ctrl Pts',(-0.497253086211501,0.573113500662185,
-2.2850308579914));
#37702=CARTESIAN_POINT('Ctrl Pts',(-0.370523007645721,2.22918406511225,
-0.762907829264197));
#37703=CARTESIAN_POINT('Ctrl Pts',(-0.243792929079945,1.85267849943624,
1.45525921586262));
#37704=CARTESIAN_POINT('Ctrl Pts',(-0.117062850514165,-0.211605512032712,
2.34570834791232));
#37705=CARTESIAN_POINT('Ctrl Pts',(0.0096672280516118,-2.085006034748,1.10015795830288));
#37706=CARTESIAN_POINT('Ctrl Pts',(0.136397306617393,-2.05384028931649,
-1.1527622711172));
#37707=CARTESIAN_POINT('Ctrl Pts',(0.220884025661244,-0.790771927602532,
-1.94723055009756));
#37708=CARTESIAN_POINT('Ctrl Pts',(0.263127385183171,-0.130371639091046,
-1.99048506606322));
#37709=CARTESIAN_POINT('',(0.,-0.160158266245241,-2.44526063636442));
#37710=CARTESIAN_POINT('Ctrl Pts',(-7.21644966006352E-16,-1.69189910824764,
1.06268379792867));
#37711=CARTESIAN_POINT('Ctrl Pts',(-7.21076027123798E-16,-1.72378408803524,
1.02301469480698));
#37712=CARTESIAN_POINT('Ctrl Pts',(-9.55233987476986E-16,-1.7539898143595,
0.98212740444666));
#37713=CARTESIAN_POINT('Ctrl Pts',(-7.7715611723761E-16,-1.78241555186685,
0.940088493339687));
#37714=CARTESIAN_POINT('Ctrl Pts',(-5.26309397071712E-16,-1.82258537863282,
0.880681212309237));
#37715=CARTESIAN_POINT('Ctrl Pts',(-3.25548323645293E-15,-1.8592027471497,
0.818975806660995));
#37716=CARTESIAN_POINT('Ctrl Pts',(-3.94129173741931E-15,-1.89232248273639,
0.755320817406468));
#37717=CARTESIAN_POINT('Ctrl Pts',(-4.33727841913663E-15,-1.91144585927058,
0.718566347413557));
#37718=CARTESIAN_POINT('Ctrl Pts',(-2.02180909249841E-15,-1.92940249600458,
0.681161140715259));
#37719=CARTESIAN_POINT('Ctrl Pts',(-1.94289029309402E-15,-1.94619730424733,
0.643167074871445));
#37720=CARTESIAN_POINT('Ctrl Pts',(-1.91494498717367E-15,-1.95214437969399,
0.629713299583723));
#37721=CARTESIAN_POINT('Ctrl Pts',(-2.14700471816057E-15,-1.95794660868843,
0.61618355001508));
#37722=CARTESIAN_POINT('Ctrl Pts',(-1.99840144432528E-15,-1.96360123760218,
0.60258734758215));
#37723=CARTESIAN_POINT('Ctrl Pts',(-1.24294016579427E-15,-1.99234793394707,
0.533467709716482));
#37724=CARTESIAN_POINT('Ctrl Pts',(-2.63660178728452E-15,-2.01723098981382,
0.46276284494659));
#37725=CARTESIAN_POINT('Ctrl Pts',(-2.60902410786912E-15,-2.03831315006211,
0.390854522909893));
#37726=CARTESIAN_POINT('Ctrl Pts',(-2.58580080554436E-15,-2.05606654307716,
0.330300163815003));
#37727=CARTESIAN_POINT('Ctrl Pts',(-2.83510209010142E-15,-2.07112396733743,
0.268891343741576));
#37728=CARTESIAN_POINT('Ctrl Pts',(-3.88578058618805E-15,-2.08350029900009,
0.206838312286158));
#37729=CARTESIAN_POINT('Ctrl Pts',(-4.39213530033574E-15,-2.08946483896602,
0.176933022398113));
#37730=CARTESIAN_POINT('Ctrl Pts',(2.96323789960187E-15,-2.0948063589925,
0.146877908022072));
#37731=CARTESIAN_POINT('Ctrl Pts',(3.05311331771918E-15,-2.09952471759412,
0.116695578438766));
#37732=CARTESIAN_POINT('Ctrl Pts',(3.09419245965773E-15,-2.10168132645084,
0.102900213399458));
#37733=CARTESIAN_POINT('Ctrl Pts',(-1.34143688527772E-15,-2.10370806138866,
0.0890758412722826));
#37734=CARTESIAN_POINT('Ctrl Pts',(-1.41553435639707E-15,-2.10560375301678,
0.0752325061236768));
#37735=CARTESIAN_POINT('Ctrl Pts',(-1.82703970662702E-15,-2.11613160552745,
-0.00164739804338759));
#37736=CARTESIAN_POINT('Ctrl Pts',(7.37197929993521E-17,-2.12259963218265,
-0.0789404011946104));
#37737=CARTESIAN_POINT('Ctrl Pts',(-3.88578058618805E-16,-2.12506850073416,
-0.156260019712051));
#37738=CARTESIAN_POINT('Ctrl Pts',(-8.67997835351761E-16,-2.12762880769991,
-0.236443291420884));
#37739=CARTESIAN_POINT('Ctrl Pts',(-6.93190692512345E-16,-2.12588873988702,
-0.316656112225985));
#37740=CARTESIAN_POINT('Ctrl Pts',(-1.38777878078145E-16,-2.1198657520015,
-0.396494553741407));
#37741=CARTESIAN_POINT('Ctrl Pts',(2.77031732747506E-16,-2.11534851108737,
-0.456373384877974));
#37742=CARTESIAN_POINT('Ctrl Pts',(6.39606772428307E-16,-2.10842110187479,
-0.51604230937309));
#37743=CARTESIAN_POINT('Ctrl Pts',(4.44089209850063E-16,-2.09907092634396,
-0.575335244944601));
#37744=CARTESIAN_POINT('Ctrl Pts',(2.97451037916379E-16,-2.09205829469584,
-0.619804946623235));
#37745=CARTESIAN_POINT('Ctrl Pts',(-8.03907321812597E-16,-2.08368251007437,
-0.664063249538941));
#37746=CARTESIAN_POINT('Ctrl Pts',(-8.04911692853238E-16,-2.07393163616088,
-0.708039858350645));
#37747=CARTESIAN_POINT('Ctrl Pts',(-8.05227535616264E-16,-2.07086529629828,
-0.721869103792363));
#37748=CARTESIAN_POINT('Ctrl Pts',(-1.27292777763199E-15,-2.06766293040564,
-0.735670486093707));
#37749=CARTESIAN_POINT('Ctrl Pts',(-1.30451205393456E-15,-2.06432404759794,
-0.749441796406119));
#37750=CARTESIAN_POINT('Ctrl Pts',(-1.33155230346768E-15,-2.06146552953607,
-0.761231829639062));
#37751=CARTESIAN_POINT('Ctrl Pts',(-1.31834190104063E-15,-2.05850921748488,
-0.772990451522471));
#37752=CARTESIAN_POINT('Ctrl Pts',(-1.33226762955019E-15,-2.05545538714023,
-0.784715877967114));
#37753=CARTESIAN_POINT('Ctrl Pts',(-1.42537956622108E-15,-2.03503648715523,
-0.863115881514751));
#37754=CARTESIAN_POINT('Ctrl Pts',(-1.25530095348547E-15,-2.0102604516796,
-0.940037252301371));
#37755=CARTESIAN_POINT('Ctrl Pts',(-9.71445146547012E-16,-1.98114950952945,
-1.0150831509489));
#37756=CARTESIAN_POINT('Ctrl Pts',(-8.74282698905283E-16,-1.97118497710373,
-1.04077099322598));
#37757=CARTESIAN_POINT('Ctrl Pts',(-7.76969050075519E-16,-1.96071209936315,
-1.06623917638337));
#37758=CARTESIAN_POINT('Ctrl Pts',(-8.32667268468867E-16,-1.94973036890473,
-1.09147191710966));
#37759=CARTESIAN_POINT('Ctrl Pts',(-1.01672237405949E-15,-1.91874143595192,
-1.16267524098863));
#37760=CARTESIAN_POINT('Ctrl Pts',(3.52175838536202E-15,-1.88370440096443,
-1.23200476678311));
#37761=CARTESIAN_POINT('Ctrl Pts',(4.91273688396632E-15,-1.84492953449254,
-1.29931700254966));
#37762=CARTESIAN_POINT('Ctrl Pts',(6.33247345622073E-15,-1.80535300899651,
-1.3680208991044));
#37763=CARTESIAN_POINT('Ctrl Pts',(2.18326834371925E-15,-1.76188209226263,
-1.43462390096206));
#37764=CARTESIAN_POINT('Ctrl Pts',(3.24740234702858E-15,-1.71479611157841,
-1.49895472013064));
#37765=CARTESIAN_POINT('Ctrl Pts',(3.50550449537181E-15,-1.7033755642285,
-1.51455794545795));
#37766=CARTESIAN_POINT('Ctrl Pts',(9.82688432106508E-17,-1.69173782534689,
-1.53003274288333));
#37767=CARTESIAN_POINT('Ctrl Pts',(4.16333634234434E-17,-1.67990922204288,
-1.54534767673703));
#37768=CARTESIAN_POINT('Ctrl Pts',(-1.9522263401941E-16,-1.63044066197322,
-1.60939646642361));
#37769=CARTESIAN_POINT('Ctrl Pts',(4.54908001959739E-16,-1.57758717960021,
-1.67072511626626));
#37770=CARTESIAN_POINT('Ctrl Pts',(6.80011602582908E-16,-1.52170661356515,
-1.72918893837752));
#37771=CARTESIAN_POINT('Ctrl Pts',(9.09600338458483E-16,-1.46471264065452,
-1.78881763812208));
#37772=CARTESIAN_POINT('Ctrl Pts',(6.75097762342671E-16,-1.40456926783563,
-1.84546690259517));
#37773=CARTESIAN_POINT('Ctrl Pts',(3.19189119579733E-16,-1.34160425438441,
-1.89896385868516));
#37774=CARTESIAN_POINT('Ctrl Pts',(-3.94837766702072E-17,-1.27815020740864,
-1.95287631226424));
#37775=CARTESIAN_POINT('Ctrl Pts',(-7.23779732573461E-16,-1.21182987269852,
-2.00358802360937));
#37776=CARTESIAN_POINT('Ctrl Pts',(-4.44089209850063E-16,-1.14293528572537,
-2.05089189769593));
#37777=CARTESIAN_POINT('Ctrl Pts',(-3.25410331228778E-16,-1.11370178776685,
-2.07096397835269));
#37778=CARTESIAN_POINT('Ctrl Pts',(1.70065938854078E-15,-1.08400432332864,
-2.09042204748417));
#37779=CARTESIAN_POINT('Ctrl Pts',(1.70696790036118E-15,-1.05386331486469,
-2.1092481624567));
#37780=CARTESIAN_POINT('Ctrl Pts',(1.7101456789279E-15,-1.03868042333605,
-2.11873141720165));
#37781=CARTESIAN_POINT('Ctrl Pts',(-3.82184296166841E-15,-1.02338072840275,
-2.12805668641633));
#37782=CARTESIAN_POINT('Ctrl Pts',(-3.65679708735911E-15,-1.0079928489119,
-2.13720641506556));
#37783=CARTESIAN_POINT('Ctrl Pts',(-2.86527130671852E-15,-0.934195770509449,
-2.18108661590086));
#37784=CARTESIAN_POINT('Ctrl Pts',(2.35760061415838E-15,-0.858275193167998,
-2.22099636818658));
#37785=CARTESIAN_POINT('Ctrl Pts',(2.26901830657766E-15,-0.780581187603902,
-2.25675949833411));
#37786=CARTESIAN_POINT('Ctrl Pts',(2.18029069254155E-15,-0.702759736268041,
-2.29258129272077));
#37787=CARTESIAN_POINT('Ctrl Pts',(9.81873011222773E-16,-0.623158277772009,
-2.32424355037343));
#37788=CARTESIAN_POINT('Ctrl Pts',(1.47798440153224E-15,-0.542089661797717,
-2.35153447222983));
#37789=CARTESIAN_POINT('Ctrl Pts',(1.96365420303237E-15,-0.46272728593377,
-2.37825100577382));
#37790=CARTESIAN_POINT('Ctrl Pts',(-4.5803513406731E-15,-0.381958046000184,
-2.40077878705499));
#37791=CARTESIAN_POINT('Ctrl Pts',(-5.32473370951081E-15,-0.300049960212024,
-2.41887709197029));
#37792=CARTESIAN_POINT('Ctrl Pts',(-5.74534480860178E-15,-0.253768033839171,
-2.42910348668461));
#37793=CARTESIAN_POINT('Ctrl Pts',(-1.31935727443843E-16,-0.20712210076169,
-2.43791483968498));
#37794=CARTESIAN_POINT('Ctrl Pts',(0.,-0.160158266245241,-2.44526063636442));
#37795=CARTESIAN_POINT('Ctrl Pts',(0.,-0.160158266245241,-2.44526063636442));
#37796=CARTESIAN_POINT('Ctrl Pts',(-0.0422433595219261,-0.971443343070605,
-2.3921235558411));
#37797=CARTESIAN_POINT('Ctrl Pts',(-0.0844867190438518,-1.74726713562105,
-1.90413144714542));
#37798=CARTESIAN_POINT('Ctrl Pts',(-0.126730078565778,-2.14156008709783,
-1.19885945828666));
#37799=CARTESIAN_POINT('Ctrl Pts',(-0.148377553639829,-2.34361425455905,
-0.83744507335068));
#37800=CARTESIAN_POINT('Ctrl Pts',(-0.17002502871388,-2.44547775967852,
-0.418972614037773));
#37801=CARTESIAN_POINT('Ctrl Pts',(-0.191672503787931,-2.44601738174545,
-0.0004368899209653));
#37802=CARTESIAN_POINT('Origin',(0.6,4.98642551413971,-0.829870828464581));
#37803=CARTESIAN_POINT('',(7.6,4.69510848352227,-0.997976115925247));
#37804=CARTESIAN_POINT('',(7.4,4.92450311121048,-0.865603320048102));
#37805=CARTESIAN_POINT('Ctrl Pts',(7.6,4.69510848352227,-0.997976115925247));
#37806=CARTESIAN_POINT('Ctrl Pts',(7.50357879858669,4.80746503585943,-0.9331404608017));
#37807=CARTESIAN_POINT('Ctrl Pts',(7.4,4.92450311121048,-0.8656033200481));
#37808=CARTESIAN_POINT('',(0.6,4.69510848352227,-0.997976115925247));
#37809=CARTESIAN_POINT('',(0.6,4.69510848352227,-0.997976115925247));
#37810=CARTESIAN_POINT('',(0.6,4.92450311121048,-0.865603320048101));
#37811=CARTESIAN_POINT('',(0.6,4.98642551413971,-0.829870828464581));
#37812=CARTESIAN_POINT('',(3.95,4.92450311121048,-0.865603320048102));
#37813=CARTESIAN_POINT('Origin',(0.6,4.81737693361399,-1.02396507727747));
#37814=CARTESIAN_POINT('',(0.6,4.85083003702482,-1.21220788311979));
#37815=CARTESIAN_POINT('Origin',(0.6,0.,0.));
#37816=CARTESIAN_POINT('',(0.6,4.69510848352227,-0.997976115925247));
#37817=CARTESIAN_POINT('Origin',(0.6,4.69510848352227,-0.997976115925247));
#37818=CARTESIAN_POINT('',(7.4,4.85083003702482,-1.21220788311979));
#37819=CARTESIAN_POINT('Ctrl Pts',(7.4,4.85083003702482,-1.21220788311979));
#37820=CARTESIAN_POINT('Ctrl Pts',(7.50357879858673,4.77138026482966,-1.10290596108179));
#37821=CARTESIAN_POINT('Ctrl Pts',(7.6,4.69510848352227,-0.997976115925248));
#37822=CARTESIAN_POINT('',(3.95,4.85083003702482,-1.21220788311979));
#37823=CARTESIAN_POINT('Origin',(3.95,0.,0.));
#37824=CARTESIAN_POINT('',(7.4,4.63692185318803,-1.87054957898135));
#37825=CARTESIAN_POINT('Origin',(7.4,0.,0.));
#37826=CARTESIAN_POINT('',(0.6,4.63692185318803,-1.87054957898136));
#37827=CARTESIAN_POINT('',(3.95,4.63692185318803,-1.87054957898135));
#37828=CARTESIAN_POINT('',(0.6,4.49279557168125,-2.19426250733164));
#37829=CARTESIAN_POINT('Origin',(0.6,0.,0.));
#37830=CARTESIAN_POINT('',(7.4,4.49279557168125,-2.19426250733164));
#37831=CARTESIAN_POINT('',(3.95,4.49279557168125,-2.19426250733164));
#37832=CARTESIAN_POINT('',(7.4,4.14668485976156,-2.79374384542038));
#37833=CARTESIAN_POINT('Origin',(7.4,0.,0.));
#37834=CARTESIAN_POINT('',(0.6,4.14668485976156,-2.79374384542038));
#37835=CARTESIAN_POINT('',(3.95,4.14668485976156,-2.79374384542038));
#37836=CARTESIAN_POINT('',(0.6,3.93840438103015,-3.08041733073337));
#37837=CARTESIAN_POINT('Origin',(0.6,0.,0.));
#37838=CARTESIAN_POINT('',(7.4,3.93840438103015,-3.08041733073337));
#37839=CARTESIAN_POINT('',(3.95,3.93840438103015,-3.08041733073337));
#37840=CARTESIAN_POINT('',(7.4,3.4752178399619,-3.59483809994421));
#37841=CARTESIAN_POINT('Origin',(7.4,0.,0.));
#37842=CARTESIAN_POINT('',(0.6,3.4752178399619,-3.59483809994421));
#37843=CARTESIAN_POINT('',(3.95,3.4752178399619,-3.59483809994421));
#37844=CARTESIAN_POINT('',(0.6,3.21188602036704,-3.83194313529973));
#37845=CARTESIAN_POINT('Origin',(0.6,0.,0.));
#37846=CARTESIAN_POINT('',(7.4,3.21188602036704,-3.83194313529973));
#37847=CARTESIAN_POINT('',(3.95,3.21188602036704,-3.83194313529973));
#37848=CARTESIAN_POINT('',(7.4,2.65186712461055,-4.23882067955343));
#37849=CARTESIAN_POINT('Origin',(7.4,0.,0.));
#37850=CARTESIAN_POINT('',(0.6,2.65186712461055,-4.23882067955343));
#37851=CARTESIAN_POINT('',(3.95,2.65186712461055,-4.23882067955343));
#37852=CARTESIAN_POINT('',(0.6,2.3449928282748,-4.41599463715025));
#37853=CARTESIAN_POINT('Origin',(0.6,0.,0.));
#37854=CARTESIAN_POINT('',(7.4,2.3449928282748,-4.41599463715025));
#37855=CARTESIAN_POINT('',(3.95,2.3449928282748,-4.41599463715025));
#37856=CARTESIAN_POINT('',(7.4,1.71261709084344,-4.69754645534783));
#37857=CARTESIAN_POINT('Origin',(7.4,0.,0.));
#37858=CARTESIAN_POINT('',(0.6,1.71261709084344,-4.69754645534783));
#37859=CARTESIAN_POINT('',(3.95,1.71261709084344,-4.69754645534783));
#37860=CARTESIAN_POINT('',(0.6,1.37561219706291,-4.807045983064));
#37861=CARTESIAN_POINT('Origin',(0.6,0.,0.));
#37862=CARTESIAN_POINT('',(7.4,1.37561219706291,-4.807045983064));
#37863=CARTESIAN_POINT('',(3.95,1.37561219706291,-4.807045983064));
#37864=CARTESIAN_POINT('',(7.4,0.698517472157875,-4.95096690971472));
#37865=CARTESIAN_POINT('Origin',(7.4,0.,0.));
#37866=CARTESIAN_POINT('',(0.6,0.698517472157875,-4.95096690971472));
#37867=CARTESIAN_POINT('',(3.95,0.698517472157875,-4.95096690971472));
#37868=CARTESIAN_POINT('',(0.6,0.346110711919692,-4.98800635275201));
#37869=CARTESIAN_POINT('Origin',(0.6,0.,0.));
#37870=CARTESIAN_POINT('',(7.4,0.346110711919692,-4.98800635275201));
#37871=CARTESIAN_POINT('',(3.95,0.346110711919692,-4.98800635275201));
#37872=CARTESIAN_POINT('',(7.4,-0.3461107119197,-4.98800635275201));
#37873=CARTESIAN_POINT('Origin',(7.4,0.,0.));
#37874=CARTESIAN_POINT('',(0.6,-0.3461107119197,-4.98800635275201));
#37875=CARTESIAN_POINT('',(3.95,-0.3461107119197,-4.98800635275201));
#37876=CARTESIAN_POINT('',(0.6,-0.698517472157882,-4.95096690971472));
#37877=CARTESIAN_POINT('Origin',(0.6,0.,0.));
#37878=CARTESIAN_POINT('',(7.4,-0.698517472157882,-4.95096690971472));
#37879=CARTESIAN_POINT('',(3.95,-0.698517472157882,-4.95096690971472));
#37880=CARTESIAN_POINT('',(7.4,-1.37561219706292,-4.807045983064));
#37881=CARTESIAN_POINT('Origin',(7.4,0.,0.));
#37882=CARTESIAN_POINT('',(0.6,-1.37561219706292,-4.807045983064));
#37883=CARTESIAN_POINT('',(3.95,-1.37561219706292,-4.807045983064));
#37884=CARTESIAN_POINT('',(0.6,-1.71261709084344,-4.69754645534783));
#37885=CARTESIAN_POINT('Origin',(0.6,0.,0.));
#37886=CARTESIAN_POINT('',(7.4,-1.71261709084344,-4.69754645534783));
#37887=CARTESIAN_POINT('',(3.95,-1.71261709084344,-4.69754645534783));
#37888=CARTESIAN_POINT('',(7.4,-2.34499282827481,-4.41599463715025));
#37889=CARTESIAN_POINT('Origin',(7.4,0.,0.));
#37890=CARTESIAN_POINT('',(0.6,-2.34499282827481,-4.41599463715025));
#37891=CARTESIAN_POINT('',(3.95,-2.34499282827481,-4.41599463715025));
#37892=CARTESIAN_POINT('',(0.6,-2.65186712461056,-4.23882067955342));
#37893=CARTESIAN_POINT('Origin',(0.6,0.,0.));
#37894=CARTESIAN_POINT('',(7.4,-2.65186712461056,-4.23882067955342));
#37895=CARTESIAN_POINT('',(3.95,-2.65186712461056,-4.23882067955342));
#37896=CARTESIAN_POINT('',(7.4,-3.21188602036705,-3.83194313529973));
#37897=CARTESIAN_POINT('Origin',(7.4,0.,0.));
#37898=CARTESIAN_POINT('',(0.6,-3.21188602036705,-3.83194313529973));
#37899=CARTESIAN_POINT('',(3.95,-3.21188602036705,-3.83194313529973));
#37900=CARTESIAN_POINT('',(0.6,-3.47521783996191,-3.59483809994421));
#37901=CARTESIAN_POINT('Origin',(0.6,0.,0.));
#37902=CARTESIAN_POINT('',(7.4,-3.47521783996191,-3.59483809994421));
#37903=CARTESIAN_POINT('',(3.95,-3.47521783996191,-3.59483809994421));
#37904=CARTESIAN_POINT('',(7.4,-3.93840438103015,-3.08041733073337));
#37905=CARTESIAN_POINT('Origin',(7.4,0.,0.));
#37906=CARTESIAN_POINT('',(0.6,-3.93840438103015,-3.08041733073337));
#37907=CARTESIAN_POINT('',(3.95,-3.93840438103015,-3.08041733073337));
#37908=CARTESIAN_POINT('',(0.6,-4.14668485976156,-2.79374384542038));
#37909=CARTESIAN_POINT('Origin',(0.6,0.,0.));
#37910=CARTESIAN_POINT('',(7.4,-4.14668485976156,-2.79374384542038));
#37911=CARTESIAN_POINT('',(3.95,-4.14668485976156,-2.79374384542038));
#37912=CARTESIAN_POINT('',(7.4,-4.49279557168126,-2.19426250733163));
#37913=CARTESIAN_POINT('Origin',(7.4,0.,0.));
#37914=CARTESIAN_POINT('',(0.6,-4.49279557168126,-2.19426250733163));
#37915=CARTESIAN_POINT('',(3.95,-4.49279557168126,-2.19426250733163));
#37916=CARTESIAN_POINT('',(0.6,-4.63692185318803,-1.87054957898135));
#37917=CARTESIAN_POINT('Origin',(0.6,0.,0.));
#37918=CARTESIAN_POINT('',(7.4,-4.63692185318803,-1.87054957898135));
#37919=CARTESIAN_POINT('',(3.95,-4.63692185318803,-1.87054957898135));
#37920=CARTESIAN_POINT('',(7.4,-4.85083003702482,-1.21220788311979));
#37921=CARTESIAN_POINT('Origin',(7.4,0.,0.));
#37922=CARTESIAN_POINT('',(0.6,-4.85083003702482,-1.21220788311979));
#37923=CARTESIAN_POINT('',(3.95,-4.85083003702482,-1.21220788311979));
#37924=CARTESIAN_POINT('',(0.6,-4.92450311121048,-0.865603320048097));
#37925=CARTESIAN_POINT('Origin',(0.6,0.,0.));
#37926=CARTESIAN_POINT('',(7.4,-4.92450311121048,-0.865603320048097));
#37927=CARTESIAN_POINT('',(3.95,-4.92450311121048,-0.865603320048097));
#37928=CARTESIAN_POINT('',(7.4,-4.99685995288536,-0.177173957596823));
#37929=CARTESIAN_POINT('Origin',(7.4,0.,0.));
#37930=CARTESIAN_POINT('',(0.6,-4.99685995288536,-0.177173957596823));
#37931=CARTESIAN_POINT('',(3.95,-4.99685995288536,-0.177173957596823));
#37932=CARTESIAN_POINT('',(0.6,-5.,-6.12323399573677E-16));
#37933=CARTESIAN_POINT('Origin',(0.6,0.,0.));
#37934=CARTESIAN_POINT('',(0.5,-5.,-6.12323399573677E-16));
#37935=CARTESIAN_POINT('',(3.95,-5.,-6.12323399573677E-16));
#37936=CARTESIAN_POINT('Origin',(0.5,0.,0.));
#37937=CARTESIAN_POINT('',(0.6,-4.99685995288536,0.177173957596825));
#37938=CARTESIAN_POINT('Origin',(0.6,0.,0.));
#37939=CARTESIAN_POINT('',(7.4,-4.99685995288536,0.177173957596825));
#37940=CARTESIAN_POINT('',(3.95,-4.99685995288536,0.177173957596825));
#37941=CARTESIAN_POINT('',(7.4,-4.92450311121048,0.865603320048101));
#37942=CARTESIAN_POINT('Origin',(7.4,0.,0.));
#37943=CARTESIAN_POINT('',(0.6,-4.92450311121048,0.865603320048101));
#37944=CARTESIAN_POINT('',(3.95,-4.92450311121048,0.865603320048101));
#37945=CARTESIAN_POINT('',(0.6,-4.85083003702482,1.21220788311979));
#37946=CARTESIAN_POINT('Origin',(0.6,0.,0.));
#37947=CARTESIAN_POINT('',(7.4,-4.85083003702482,1.21220788311979));
#37948=CARTESIAN_POINT('',(3.95,-4.85083003702482,1.21220788311979));
#37949=CARTESIAN_POINT('',(7.4,-4.63692185318803,1.87054957898135));
#37950=CARTESIAN_POINT('Origin',(7.4,0.,0.));
#37951=CARTESIAN_POINT('',(0.6,-4.63692185318803,1.87054957898135));
#37952=CARTESIAN_POINT('',(3.95,-4.63692185318803,1.87054957898135));
#37953=CARTESIAN_POINT('',(0.6,-4.49279557168125,2.19426250733163));
#37954=CARTESIAN_POINT('Origin',(0.6,0.,0.));
#37955=CARTESIAN_POINT('',(7.4,-4.49279557168125,2.19426250733164));
#37956=CARTESIAN_POINT('',(3.95,-4.49279557168125,2.19426250733164));
#37957=CARTESIAN_POINT('',(7.4,-4.14668485976156,2.79374384542038));
#37958=CARTESIAN_POINT('Origin',(7.4,0.,0.));
#37959=CARTESIAN_POINT('',(0.6,-4.14668485976156,2.79374384542038));
#37960=CARTESIAN_POINT('',(3.95,-4.14668485976156,2.79374384542038));
#37961=CARTESIAN_POINT('',(0.6,-3.93840438103015,3.08041733073337));
#37962=CARTESIAN_POINT('Origin',(0.6,0.,0.));
#37963=CARTESIAN_POINT('',(7.4,-3.93840438103015,3.08041733073337));
#37964=CARTESIAN_POINT('',(3.95,-3.93840438103015,3.08041733073337));
#37965=CARTESIAN_POINT('',(7.4,-3.47521783996191,3.59483809994421));
#37966=CARTESIAN_POINT('Origin',(7.4,0.,0.));
#37967=CARTESIAN_POINT('',(0.6,-3.47521783996191,3.59483809994421));
#37968=CARTESIAN_POINT('',(3.95,-3.47521783996191,3.59483809994421));
#37969=CARTESIAN_POINT('',(0.6,-3.21188602036704,3.83194313529973));
#37970=CARTESIAN_POINT('Origin',(0.6,0.,0.));
#37971=CARTESIAN_POINT('',(7.4,-3.21188602036704,3.83194313529973));
#37972=CARTESIAN_POINT('',(3.95,-3.21188602036704,3.83194313529973));
#37973=CARTESIAN_POINT('',(7.4,-2.65186712461055,4.23882067955342));
#37974=CARTESIAN_POINT('Origin',(7.4,0.,0.));
#37975=CARTESIAN_POINT('',(0.6,-2.65186712461055,4.23882067955342));
#37976=CARTESIAN_POINT('',(3.95,-2.65186712461055,4.23882067955342));
#37977=CARTESIAN_POINT('',(0.6,-2.3449928282748,4.41599463715025));
#37978=CARTESIAN_POINT('Origin',(0.6,0.,0.));
#37979=CARTESIAN_POINT('',(7.4,-2.3449928282748,4.41599463715025));
#37980=CARTESIAN_POINT('',(3.95,-2.3449928282748,4.41599463715025));
#37981=CARTESIAN_POINT('',(7.4,-1.71261709084343,4.69754645534783));
#37982=CARTESIAN_POINT('Origin',(7.4,0.,0.));
#37983=CARTESIAN_POINT('',(0.6,-1.71261709084343,4.69754645534783));
#37984=CARTESIAN_POINT('',(3.95,-1.71261709084343,4.69754645534783));
#37985=CARTESIAN_POINT('',(0.6,-1.37561219706291,4.807045983064));
#37986=CARTESIAN_POINT('Origin',(0.6,0.,0.));
#37987=CARTESIAN_POINT('',(7.4,-1.37561219706291,4.807045983064));
#37988=CARTESIAN_POINT('',(3.95,-1.37561219706291,4.807045983064));
#37989=CARTESIAN_POINT('',(7.4,-0.698517472157877,4.95096690971473));
#37990=CARTESIAN_POINT('Origin',(7.4,0.,0.));
#37991=CARTESIAN_POINT('',(0.6,-0.698517472157877,4.95096690971473));
#37992=CARTESIAN_POINT('',(3.95,-0.698517472157877,4.95096690971473));
#37993=CARTESIAN_POINT('',(0.6,-0.346110711919694,4.98800635275201));
#37994=CARTESIAN_POINT('Origin',(0.6,0.,0.));
#37995=CARTESIAN_POINT('',(7.4,-0.346110711919694,4.98800635275201));
#37996=CARTESIAN_POINT('',(3.95,-0.346110711919694,4.98800635275201));
#37997=CARTESIAN_POINT('',(7.4,0.346110711919697,4.98800635275201));
#37998=CARTESIAN_POINT('Origin',(7.4,0.,0.));
#37999=CARTESIAN_POINT('',(0.6,0.346110711919695,4.98800635275201));
#38000=CARTESIAN_POINT('',(3.95,0.346110711919697,4.98800635275201));
#38001=CARTESIAN_POINT('',(0.6,0.698517472157879,4.95096690971472));
#38002=CARTESIAN_POINT('Origin',(0.6,0.,0.));
#38003=CARTESIAN_POINT('',(7.4,0.698517472157878,4.95096690971472));
#38004=CARTESIAN_POINT('',(3.95,0.698517472157878,4.95096690971472));
#38005=CARTESIAN_POINT('',(7.4,1.37561219706292,4.807045983064));
#38006=CARTESIAN_POINT('Origin',(7.4,0.,0.));
#38007=CARTESIAN_POINT('',(0.6,1.37561219706292,4.807045983064));
#38008=CARTESIAN_POINT('',(3.95,1.37561219706292,4.807045983064));
#38009=CARTESIAN_POINT('',(0.6,1.71261709084344,4.69754645534783));
#38010=CARTESIAN_POINT('Origin',(0.6,0.,0.));
#38011=CARTESIAN_POINT('',(7.4,1.71261709084344,4.69754645534783));
#38012=CARTESIAN_POINT('',(3.95,1.71261709084344,4.69754645534783));
#38013=CARTESIAN_POINT('',(7.4,2.3449928282748,4.41599463715025));
#38014=CARTESIAN_POINT('Origin',(7.4,0.,0.));
#38015=CARTESIAN_POINT('',(0.6,2.3449928282748,4.41599463715025));
#38016=CARTESIAN_POINT('',(3.95,2.3449928282748,4.41599463715025));
#38017=CARTESIAN_POINT('',(0.6,2.65186712461056,4.23882067955342));
#38018=CARTESIAN_POINT('Origin',(0.6,0.,0.));
#38019=CARTESIAN_POINT('',(7.4,2.65186712461056,4.23882067955342));
#38020=CARTESIAN_POINT('',(3.95,2.65186712461056,4.23882067955342));
#38021=CARTESIAN_POINT('',(7.4,3.21188602036705,3.83194313529973));
#38022=CARTESIAN_POINT('Origin',(7.4,0.,0.));
#38023=CARTESIAN_POINT('',(0.6,3.21188602036705,3.83194313529973));
#38024=CARTESIAN_POINT('',(3.95,3.21188602036705,3.83194313529973));
#38025=CARTESIAN_POINT('',(0.6,3.47521783996191,3.59483809994421));
#38026=CARTESIAN_POINT('Origin',(0.6,0.,0.));
#38027=CARTESIAN_POINT('',(7.4,3.47521783996191,3.59483809994421));
#38028=CARTESIAN_POINT('',(3.95,3.47521783996191,3.59483809994421));
#38029=CARTESIAN_POINT('',(7.4,3.93840438103015,3.08041733073337));
#38030=CARTESIAN_POINT('Origin',(7.4,0.,0.));
#38031=CARTESIAN_POINT('',(0.6,3.93840438103015,3.08041733073337));
#38032=CARTESIAN_POINT('',(3.95,3.93840438103015,3.08041733073337));
#38033=CARTESIAN_POINT('',(0.6,4.14668485976156,2.79374384542038));
#38034=CARTESIAN_POINT('Origin',(0.6,0.,0.));
#38035=CARTESIAN_POINT('',(7.4,4.14668485976156,2.79374384542038));
#38036=CARTESIAN_POINT('',(3.95,4.14668485976156,2.79374384542038));
#38037=CARTESIAN_POINT('',(7.4,4.49279557168126,2.19426250733163));
#38038=CARTESIAN_POINT('Origin',(7.4,0.,0.));
#38039=CARTESIAN_POINT('',(0.6,4.49279557168126,2.19426250733163));
#38040=CARTESIAN_POINT('',(3.95,4.49279557168126,2.19426250733163));
#38041=CARTESIAN_POINT('',(0.6,4.63692185318803,1.87054957898135));
#38042=CARTESIAN_POINT('Origin',(0.6,0.,0.));
#38043=CARTESIAN_POINT('',(7.4,4.63692185318803,1.87054957898135));
#38044=CARTESIAN_POINT('',(3.95,4.63692185318803,1.87054957898135));
#38045=CARTESIAN_POINT('',(7.4,4.85083003702482,1.21220788311979));
#38046=CARTESIAN_POINT('Origin',(7.4,0.,0.));
#38047=CARTESIAN_POINT('',(0.6,4.85083003702482,1.21220788311979));
#38048=CARTESIAN_POINT('',(3.95,4.85083003702482,1.21220788311979));
#38049=CARTESIAN_POINT('',(0.6,4.92450311121048,0.865603320048098));
#38050=CARTESIAN_POINT('Origin',(0.6,0.,0.));
#38051=CARTESIAN_POINT('',(7.4,4.92450311121048,0.865603320048098));
#38052=CARTESIAN_POINT('',(3.95,4.92450311121048,0.865603320048098));
#38053=CARTESIAN_POINT('',(7.4,4.99685995288536,0.177173957596825));
#38054=CARTESIAN_POINT('Origin',(7.4,0.,0.));
#38055=CARTESIAN_POINT('',(0.6,4.99685995288536,0.177173957596825));
#38056=CARTESIAN_POINT('',(3.95,4.99685995288536,0.177173957596825));
#38057=CARTESIAN_POINT('',(0.6,4.99685995288536,-0.177173957596824));
#38058=CARTESIAN_POINT('Origin',(0.6,0.,0.));
#38059=CARTESIAN_POINT('',(7.4,4.99685995288536,-0.177173957596824));
#38060=CARTESIAN_POINT('',(3.95,4.99685995288536,-0.177173957596824));
#38061=CARTESIAN_POINT('Origin',(7.4,0.,0.));
#38062=CARTESIAN_POINT('Origin',(0.6,4.70492030578719,-1.84847231956321));
#38063=CARTESIAN_POINT('',(7.6,4.38501819668448,-1.95233588676384));
#38064=CARTESIAN_POINT('Ctrl Pts',(7.6,4.38501819668448,-1.95233588676384));
#38065=CARTESIAN_POINT('Ctrl Pts',(7.5035787985868,4.50839957946168,-1.91227728703366));
#38066=CARTESIAN_POINT('Ctrl Pts',(7.4,4.63692185318803,-1.87054957898135));
#38067=CARTESIAN_POINT('',(0.6,4.38501819668448,-1.95233588676384));
#38068=CARTESIAN_POINT('',(0.6,4.38501819668448,-1.95233588676384));
#38069=CARTESIAN_POINT('',(0.6,4.70492030578719,-1.84847231956321));
#38070=CARTESIAN_POINT('Origin',(0.6,4.49921137888981,-2.00317796714832));
#38071=CARTESIAN_POINT('',(0.6,4.38501819668448,-1.95233588676384));
#38072=CARTESIAN_POINT('Origin',(0.6,4.38501819668448,-1.95233588676384));
#38073=CARTESIAN_POINT('Ctrl Pts',(7.4,4.49279557168125,-2.19426250733164));
#38074=CARTESIAN_POINT('Ctrl Pts',(7.50357879858675,4.43780711505025,-2.07083055806237));
#38075=CARTESIAN_POINT('Ctrl Pts',(7.6,4.38501819668448,-1.95233588676385));
#38076=CARTESIAN_POINT('Origin',(0.6,4.21778750335929,-2.78628670034263));
#38077=CARTESIAN_POINT('',(7.6,3.88328157299975,-2.82136921100387));
#38078=CARTESIAN_POINT('Ctrl Pts',(7.6,3.88328157299975,-2.82136921100387));
#38079=CARTESIAN_POINT('Ctrl Pts',(7.50357879858666,4.01229542774037,-2.80783841969766));
#38080=CARTESIAN_POINT('Ctrl Pts',(7.4,4.14668485976156,-2.79374384542038));
#38081=CARTESIAN_POINT('',(0.6,3.88328157299975,-2.82136921100387));
#38082=CARTESIAN_POINT('',(0.6,3.88328157299975,-2.82136921100387));
#38083=CARTESIAN_POINT('',(0.6,4.21778750335929,-2.78628670034263));
#38084=CARTESIAN_POINT('Origin',(0.6,3.98440869729662,-2.89484236754043));
#38085=CARTESIAN_POINT('',(0.6,3.88328157299975,-2.82136921100387));
#38086=CARTESIAN_POINT('Origin',(0.6,3.88328157299975,-2.82136921100387));
#38087=CARTESIAN_POINT('Ctrl Pts',(7.4,3.93840438103015,-3.08041733073338));
#38088=CARTESIAN_POINT('Ctrl Pts',(7.50357879858664,3.91028049938202,-2.94824992270828));
#38089=CARTESIAN_POINT('Ctrl Pts',(7.6,3.88328157299975,-2.82136921100387));
#38090=CARTESIAN_POINT('Origin',(0.6,3.54631714784465,-3.6023269822301));
#38091=CARTESIAN_POINT('',(7.6,3.21182691052252,-3.56709516229149));
#38092=CARTESIAN_POINT('Ctrl Pts',(7.6,3.21182691052252,-3.56709516229149));
#38093=CARTESIAN_POINT('Ctrl Pts',(7.50357879858679,3.34083471269687,-3.58068353991731));
#38094=CARTESIAN_POINT('Ctrl Pts',(7.4,3.47521783996191,-3.59483809994421));
#38095=CARTESIAN_POINT('',(0.6,3.21182691052252,-3.56709516229149));
#38096=CARTESIAN_POINT('',(0.6,3.21182691052252,-3.56709516229149));
#38097=CARTESIAN_POINT('',(0.6,3.54631714784465,-3.6023269822301));
#38098=CARTESIAN_POINT('Origin',(0.6,3.29546823631738,-3.65998826547617));
#38099=CARTESIAN_POINT('',(0.6,3.21182691052252,-3.56709516229149));
#38100=CARTESIAN_POINT('Origin',(0.6,3.21182691052252,-3.56709516229149));
#38101=CARTESIAN_POINT('Ctrl Pts',(7.4,3.21188602036704,-3.83194313529974));
#38102=CARTESIAN_POINT('Ctrl Pts',(7.50357879858676,3.2118558622831,-3.6968166184588));
#38103=CARTESIAN_POINT('Ctrl Pts',(7.6,3.21182691052252,-3.56709516229149));
#38104=CARTESIAN_POINT('Origin',(0.6,2.71985571585149,-4.26092828911142));
#38105=CARTESIAN_POINT('',(7.6,2.4,-4.15692193816531));
#38106=CARTESIAN_POINT('Ctrl Pts',(7.6,2.4,-4.15692193816531));
#38107=CARTESIAN_POINT('Ctrl Pts',(7.5035787985868,2.52336348960512,-4.19703560741661));
#38108=CARTESIAN_POINT('Ctrl Pts',(7.4,2.65186712461055,-4.23882067955342));
#38109=CARTESIAN_POINT('',(0.6,2.4,-4.15692193816531));
#38110=CARTESIAN_POINT('',(0.6,2.4,-4.15692193816531));
#38111=CARTESIAN_POINT('',(0.6,2.71985571585149,-4.26092828911142));
#38112=CARTESIAN_POINT('Origin',(0.6,2.4625,-4.26517511363836));
#38113=CARTESIAN_POINT('',(0.6,2.4,-4.15692193816531));
#38114=CARTESIAN_POINT('Origin',(0.6,2.4,-4.15692193816531));
#38115=CARTESIAN_POINT('Ctrl Pts',(7.4,2.3449928282748,-4.41599463715025));
#38116=CARTESIAN_POINT('Ctrl Pts',(7.50357879858669,2.37305771180804,-4.28381468868864));
#38117=CARTESIAN_POINT('Ctrl Pts',(7.6,2.4,-4.15692193816531));
#38118=CARTESIAN_POINT('Origin',(0.6,1.77452353775989,-4.73330658355616));
#38119=CARTESIAN_POINT('',(7.6,1.48328157299975,-4.56507127821674));
#38120=CARTESIAN_POINT('Ctrl Pts',(7.6,1.48328157299975,-4.56507127821674));
#38121=CARTESIAN_POINT('Ctrl Pts',(7.50357879858666,1.59560917357637,-4.62995707926061));
#38122=CARTESIAN_POINT('Ctrl Pts',(7.4,1.71261709084344,-4.69754645534783));
#38123=CARTESIAN_POINT('',(0.6,1.48328157299975,-4.56507127821674));
#38124=CARTESIAN_POINT('',(0.6,1.48328157299975,-4.56507127821674));
#38125=CARTESIAN_POINT('',(0.6,1.77452353775989,-4.73330658355616));
#38126=CARTESIAN_POINT('Origin',(0.6,1.52190869729661,-4.68395334275363));
#38127=CARTESIAN_POINT('',(0.6,1.48328157299975,-4.56507127821674));
#38128=CARTESIAN_POINT('Origin',(0.6,1.48328157299975,-4.56507127821674));
#38129=CARTESIAN_POINT('Ctrl Pts',(7.4,1.37561219706291,-4.807045983064));
#38130=CARTESIAN_POINT('Ctrl Pts',(7.50357879858666,1.43054555213267,-4.68358950099919));
#38131=CARTESIAN_POINT('Ctrl Pts',(7.6,1.48328157299975,-4.56507127821674));
#38132=CARTESIAN_POINT('Origin',(0.6,0.751636165959509,-4.99881666737456));
#38133=CARTESIAN_POINT('',(7.6,0.501736623684734,-4.77370509776771));
#38134=CARTESIAN_POINT('Ctrl Pts',(7.6,0.501736623684735,-4.77370509776771));
#38135=CARTESIAN_POINT('Ctrl Pts',(7.50357879858666,0.59811908007984,-4.86052720974185));
#38136=CARTESIAN_POINT('Ctrl Pts',(7.4,0.698517472157876,-4.95096690971473));
#38137=CARTESIAN_POINT('',(0.6,0.501736623684734,-4.77370509776771));
#38138=CARTESIAN_POINT('',(0.6,0.501736623684734,-4.77370509776771));
#38139=CARTESIAN_POINT('',(0.6,0.751636165959509,-4.99881666737456));
#38140=CARTESIAN_POINT('Origin',(0.6,0.514802681593191,-4.89802033468875));
#38141=CARTESIAN_POINT('',(0.6,0.501736623684734,-4.77370509776771));
#38142=CARTESIAN_POINT('Origin',(0.6,0.501736623684734,-4.77370509776771));
#38143=CARTESIAN_POINT('Ctrl Pts',(7.4,0.346110711919692,-4.98800635275201));
#38144=CARTESIAN_POINT('Ctrl Pts',(7.50357879858676,0.425511687310016,-4.87866897776003));
#38145=CARTESIAN_POINT('Ctrl Pts',(7.6,0.501736623684734,-4.77370509776771));
#38146=CARTESIAN_POINT('Origin',(0.6,-0.304101313043792,-5.045854475845));
#38147=CARTESIAN_POINT('',(7.6,-0.50173662368474,-4.77370509776771));
#38148=CARTESIAN_POINT('Ctrl Pts',(7.6,-0.50173662368474,-4.77370509776771));
#38149=CARTESIAN_POINT('Ctrl Pts',(7.50357879858676,-0.425511687310022,
-4.87866897776003));
#38150=CARTESIAN_POINT('Ctrl Pts',(7.4,-0.346110711919699,-4.98800635275201));
#38151=CARTESIAN_POINT('',(0.6,-0.50173662368474,-4.77370509776771));
#38152=CARTESIAN_POINT('',(0.6,-0.50173662368474,-4.77370509776771));
#38153=CARTESIAN_POINT('',(0.6,-0.304101313043792,-5.045854475845));
#38154=CARTESIAN_POINT('Origin',(0.6,-0.514802681593197,-4.89802033468875));
#38155=CARTESIAN_POINT('',(0.6,-0.50173662368474,-4.77370509776771));
#38156=CARTESIAN_POINT('Origin',(0.6,-0.50173662368474,-4.77370509776771));
#38157=CARTESIAN_POINT('Ctrl Pts',(7.4,-0.698517472157881,-4.95096690971472));
#38158=CARTESIAN_POINT('Ctrl Pts',(7.50357879858675,-0.598119080079759,
-4.86052720974177));
#38159=CARTESIAN_POINT('Ctrl Pts',(7.6,-0.501736623684741,-4.77370509776771));
#38160=CARTESIAN_POINT('Origin',(0.6,-1.34654810542708,-4.87236423102489));
#38161=CARTESIAN_POINT('',(7.6,-1.48328157299975,-4.56507127821674));
#38162=CARTESIAN_POINT('Ctrl Pts',(7.6,-1.48328157299975,-4.56507127821674));
#38163=CARTESIAN_POINT('Ctrl Pts',(7.50357879858675,-1.43054555213272,-4.68358950099908));
#38164=CARTESIAN_POINT('Ctrl Pts',(7.4,-1.37561219706292,-4.807045983064));
#38165=CARTESIAN_POINT('',(0.6,-1.48328157299975,-4.56507127821674));
#38166=CARTESIAN_POINT('',(0.6,-1.48328157299975,-4.56507127821674));
#38167=CARTESIAN_POINT('',(0.6,-1.34654810542708,-4.87236423102489));
#38168=CARTESIAN_POINT('Origin',(0.6,-1.52190869729662,-4.68395334275363));
#38169=CARTESIAN_POINT('',(0.6,-1.48328157299975,-4.56507127821674));
#38170=CARTESIAN_POINT('Origin',(0.6,-1.48328157299975,-4.56507127821674));
#38171=CARTESIAN_POINT('Ctrl Pts',(7.4,-1.71261709084344,-4.69754645534783));
#38172=CARTESIAN_POINT('Ctrl Pts',(7.50357879858678,-1.59560917357623,-4.62995707926053));
#38173=CARTESIAN_POINT('Ctrl Pts',(7.6,-1.48328157299975,-4.56507127821674));
#38174=CARTESIAN_POINT('Origin',(0.6,-2.3301442841485,-4.48592828911141));
#38175=CARTESIAN_POINT('',(7.6,-2.4,-4.1569219381653));
#38176=CARTESIAN_POINT('Ctrl Pts',(7.6,-2.4,-4.15692193816531));
#38177=CARTESIAN_POINT('Ctrl Pts',(7.50357879858655,-2.37305771180801,-4.28381468868881));
#38178=CARTESIAN_POINT('Ctrl Pts',(7.4,-2.34499282827481,-4.41599463715025));
#38179=CARTESIAN_POINT('',(0.6,-2.4,-4.1569219381653));
#38180=CARTESIAN_POINT('',(0.6,-2.4,-4.1569219381653));
#38181=CARTESIAN_POINT('',(0.6,-2.3301442841485,-4.48592828911141));
#38182=CARTESIAN_POINT('Origin',(0.6,-2.4625,-4.26517511363836));
#38183=CARTESIAN_POINT('',(0.6,-2.4,-4.1569219381653));
#38184=CARTESIAN_POINT('Origin',(0.6,-2.4,-4.1569219381653));
#38185=CARTESIAN_POINT('Ctrl Pts',(7.4,-2.65186712461056,-4.23882067955342));
#38186=CARTESIAN_POINT('Ctrl Pts',(7.5035787985868,-2.52336348960513,-4.19703560741661));
#38187=CARTESIAN_POINT('Ctrl Pts',(7.6,-2.4,-4.1569219381653));
#38188=CARTESIAN_POINT('Origin',(0.6,-3.21190197637982,-3.90343575509158));
#38189=CARTESIAN_POINT('',(7.6,-3.21182691052252,-3.56709516229149));
#38190=CARTESIAN_POINT('Ctrl Pts',(7.6,-3.21182691052252,-3.56709516229149));
#38191=CARTESIAN_POINT('Ctrl Pts',(7.5035787985866,-3.2118558622831,-3.69681661845901));
#38192=CARTESIAN_POINT('Ctrl Pts',(7.4,-3.21188602036705,-3.83194313529973));
#38193=CARTESIAN_POINT('',(0.6,-3.21182691052252,-3.56709516229149));
#38194=CARTESIAN_POINT('',(0.6,-3.21182691052252,-3.56709516229149));
#38195=CARTESIAN_POINT('',(0.6,-3.21190197637982,-3.90343575509158));
#38196=CARTESIAN_POINT('Origin',(0.6,-3.29546823631738,-3.65998826547617));
#38197=CARTESIAN_POINT('',(0.6,-3.21182691052252,-3.56709516229149));
#38198=CARTESIAN_POINT('Origin',(0.6,-3.21182691052252,-3.56709516229149));
#38199=CARTESIAN_POINT('Ctrl Pts',(7.4,-3.47521783996191,-3.59483809994421));
#38200=CARTESIAN_POINT('Ctrl Pts',(7.5035787985868,-3.34083471269686,-3.58068353991731));
#38201=CARTESIAN_POINT('Ctrl Pts',(7.6,-3.21182691052252,-3.56709516229149));
#38202=CARTESIAN_POINT('Origin',(0.6,-3.95328413982768,-3.15034434781135));
#38203=CARTESIAN_POINT('',(7.6,-3.88328157299975,-2.82136921100387));
#38204=CARTESIAN_POINT('Ctrl Pts',(7.6,-3.88328157299975,-2.82136921100387));
#38205=CARTESIAN_POINT('Ctrl Pts',(7.50357879858668,-3.91028049938201,-2.94824992270822));
#38206=CARTESIAN_POINT('Ctrl Pts',(7.4,-3.93840438103015,-3.08041733073337));
#38207=CARTESIAN_POINT('',(0.6,-3.88328157299975,-2.82136921100387));
#38208=CARTESIAN_POINT('',(0.6,-3.88328157299975,-2.82136921100387));
#38209=CARTESIAN_POINT('',(0.6,-3.95328413982768,-3.15034434781135));
#38210=CARTESIAN_POINT('Origin',(0.6,-3.98440869729662,-2.89484236754043));
#38211=CARTESIAN_POINT('',(0.6,-3.88328157299975,-2.82136921100387));
#38212=CARTESIAN_POINT('Origin',(0.6,-3.88328157299975,-2.82136921100387));
#38213=CARTESIAN_POINT('Ctrl Pts',(7.4,-4.14668485976156,-2.79374384542038));
#38214=CARTESIAN_POINT('Ctrl Pts',(7.50357879858676,-4.01229542774023,-2.80783841969767));
#38215=CARTESIAN_POINT('Ctrl Pts',(7.6,-3.88328157299975,-2.82136921100387));
#38216=CARTESIAN_POINT('Origin',(0.6,-4.52188881640308,-2.25956777550237));
#38217=CARTESIAN_POINT('',(7.6,-4.38501819668449,-1.95233588676384));
#38218=CARTESIAN_POINT('Ctrl Pts',(7.6,-4.38501819668449,-1.95233588676384));
#38219=CARTESIAN_POINT('Ctrl Pts',(7.50357879858659,-4.43780711505034,-2.07083055806256));
#38220=CARTESIAN_POINT('Ctrl Pts',(7.4,-4.49279557168126,-2.19426250733163));
#38221=CARTESIAN_POINT('',(0.6,-4.38501819668449,-1.95233588676384));
#38222=CARTESIAN_POINT('',(0.6,-4.38501819668449,-1.95233588676384));
#38223=CARTESIAN_POINT('',(0.6,-4.52188881640308,-2.25956777550237));
#38224=CARTESIAN_POINT('Origin',(0.6,-4.49921137888981,-2.00317796714831));
#38225=CARTESIAN_POINT('',(0.6,-4.38501819668449,-1.95233588676384));
#38226=CARTESIAN_POINT('Origin',(0.6,-4.38501819668449,-1.95233588676384));
#38227=CARTESIAN_POINT('Ctrl Pts',(7.4,-4.63692185318803,-1.87054957898135));
#38228=CARTESIAN_POINT('Ctrl Pts',(7.50357879858679,-4.5083995794617,-1.91227728703365));
#38229=CARTESIAN_POINT('Ctrl Pts',(7.6,-4.38501819668449,-1.95233588676384));
#38230=CARTESIAN_POINT('Origin',(0.6,-4.89286525327172,-1.27003724879479));
#38231=CARTESIAN_POINT('',(7.6,-4.69510848352227,-0.997976115925243));
#38232=CARTESIAN_POINT('Ctrl Pts',(7.6,-4.69510848352227,-0.997976115925244));
#38233=CARTESIAN_POINT('Ctrl Pts',(7.50357879858667,-4.77138026482971,-1.10290596108185));
#38234=CARTESIAN_POINT('Ctrl Pts',(7.4,-4.85083003702482,-1.21220788311979));
#38235=CARTESIAN_POINT('',(0.6,-4.69510848352227,-0.997976115925243));
#38236=CARTESIAN_POINT('',(0.6,-4.69510848352227,-0.997976115925243));
#38237=CARTESIAN_POINT('',(0.6,-4.89286525327172,-1.27003724879479));
#38238=CARTESIAN_POINT('Origin',(0.6,-4.81737693361399,-1.02396507727746));
#38239=CARTESIAN_POINT('',(0.6,-4.69510848352227,-0.997976115925243));
#38240=CARTESIAN_POINT('Origin',(0.6,-4.69510848352227,-0.997976115925243));
#38241=CARTESIAN_POINT('Ctrl Pts',(7.4,-4.92450311121048,-0.865603320048097));
#38242=CARTESIAN_POINT('Ctrl Pts',(7.50357879858677,-4.80746503585935,-0.933140460801746));
#38243=CARTESIAN_POINT('Ctrl Pts',(7.6,-4.69510848352227,-0.997976115925243));
#38244=CARTESIAN_POINT('Origin',(0.6,-5.05,-0.224999999999999));
#38245=CARTESIAN_POINT('',(7.6,-4.8,5.87830463590729E-16));
#38246=CARTESIAN_POINT('Ctrl Pts',(7.6,-4.8,-2.83461197776636E-16));
#38247=CARTESIAN_POINT('Ctrl Pts',(7.50357879858684,-4.89642120141316,-0.0867790812718465));
#38248=CARTESIAN_POINT('Ctrl Pts',(7.4,-4.99685995288536,-0.177173957596824));
#38249=CARTESIAN_POINT('',(0.6,-4.8,5.87830463590729E-16));
#38250=CARTESIAN_POINT('',(0.6,-4.8,5.87830463590729E-16));
#38251=CARTESIAN_POINT('',(0.6,-5.05,-0.224999999999999));
#38252=CARTESIAN_POINT('Origin',(0.6,-4.925,6.03138548580071E-16));
#38253=CARTESIAN_POINT('',(0.6,-4.8,5.87830463590729E-16));
#38254=CARTESIAN_POINT('Origin',(0.6,-4.8,5.87830463590729E-16));
#38255=CARTESIAN_POINT('Ctrl Pts',(7.4,-4.99685995288536,0.177173957596825));
#38256=CARTESIAN_POINT('Ctrl Pts',(7.50357879858667,-4.89642120141333,0.0867790812719992));
#38257=CARTESIAN_POINT('Ctrl Pts',(7.6,-4.8,1.41730598888318E-15));
#38258=CARTESIAN_POINT('Origin',(0.6,-4.98642551413971,0.82987082846458));
#38259=CARTESIAN_POINT('',(7.6,-4.69510848352227,0.997976115925247));
#38260=CARTESIAN_POINT('Ctrl Pts',(7.6,-4.69510848352227,0.997976115925246));
#38261=CARTESIAN_POINT('Ctrl Pts',(7.50357879858674,-4.80746503585938,0.933140460801728));
#38262=CARTESIAN_POINT('Ctrl Pts',(7.4,-4.92450311121048,0.8656033200481));
#38263=CARTESIAN_POINT('',(0.6,-4.69510848352227,0.997976115925247));
#38264=CARTESIAN_POINT('',(0.6,-4.69510848352227,0.997976115925247));
#38265=CARTESIAN_POINT('',(0.6,-4.98642551413971,0.82987082846458));
#38266=CARTESIAN_POINT('Origin',(0.6,-4.81737693361399,1.02396507727747));
#38267=CARTESIAN_POINT('',(0.6,-4.69510848352227,0.997976115925247));
#38268=CARTESIAN_POINT('Origin',(0.6,-4.69510848352227,0.997976115925247));
#38269=CARTESIAN_POINT('Ctrl Pts',(7.4,-4.85083003702482,1.21220788311979));
#38270=CARTESIAN_POINT('Ctrl Pts',(7.50357879858672,-4.77138026482967,1.1029059610818));
#38271=CARTESIAN_POINT('Ctrl Pts',(7.6,-4.69510848352227,0.997976115925247));
#38272=CARTESIAN_POINT('Origin',(0.6,-4.70492030578719,1.84847231956321));
#38273=CARTESIAN_POINT('',(7.6,-4.38501819668448,1.95233588676384));
#38274=CARTESIAN_POINT('Ctrl Pts',(7.6,-4.38501819668448,1.95233588676384));
#38275=CARTESIAN_POINT('Ctrl Pts',(7.50357879858671,-4.50839957946179,1.91227728703362));
#38276=CARTESIAN_POINT('Ctrl Pts',(7.4,-4.63692185318803,1.87054957898135));
#38277=CARTESIAN_POINT('',(0.6,-4.38501819668448,1.95233588676384));
#38278=CARTESIAN_POINT('',(0.6,-4.38501819668448,1.95233588676384));
#38279=CARTESIAN_POINT('',(0.6,-4.70492030578719,1.84847231956321));
#38280=CARTESIAN_POINT('Origin',(0.6,-4.49921137888981,2.00317796714832));
#38281=CARTESIAN_POINT('',(0.6,-4.38501819668448,1.95233588676384));
#38282=CARTESIAN_POINT('Origin',(0.6,-4.38501819668448,1.95233588676384));
#38283=CARTESIAN_POINT('Ctrl Pts',(7.4,-4.49279557168125,2.19426250733164));
#38284=CARTESIAN_POINT('Ctrl Pts',(7.50357879858679,-4.43780711505023,2.07083055806232));
#38285=CARTESIAN_POINT('Ctrl Pts',(7.6,-4.38501819668448,1.95233588676384));
#38286=CARTESIAN_POINT('Origin',(0.6,-4.21778750335929,2.78628670034263));
#38287=CARTESIAN_POINT('',(7.6,-3.88328157299975,2.82136921100387));
#38288=CARTESIAN_POINT('Ctrl Pts',(7.6,-3.88328157299975,2.82136921100387));
#38289=CARTESIAN_POINT('Ctrl Pts',(7.50357879858675,-4.01229542774025,2.80783841969767));
#38290=CARTESIAN_POINT('Ctrl Pts',(7.4,-4.14668485976156,2.79374384542038));
#38291=CARTESIAN_POINT('',(0.6,-3.88328157299975,2.82136921100387));
#38292=CARTESIAN_POINT('',(0.6,-3.88328157299975,2.82136921100387));
#38293=CARTESIAN_POINT('',(0.6,-4.21778750335929,2.78628670034263));
#38294=CARTESIAN_POINT('Origin',(0.6,-3.98440869729662,2.89484236754043));
#38295=CARTESIAN_POINT('',(0.6,-3.88328157299975,2.82136921100387));
#38296=CARTESIAN_POINT('Origin',(0.6,-3.88328157299975,2.82136921100387));
#38297=CARTESIAN_POINT('Ctrl Pts',(7.4,-3.93840438103015,3.08041733073337));
#38298=CARTESIAN_POINT('Ctrl Pts',(7.50357879858669,-3.910280499382,2.94824992270821));
#38299=CARTESIAN_POINT('Ctrl Pts',(7.6,-3.88328157299975,2.82136921100387));
#38300=CARTESIAN_POINT('Origin',(0.6,-3.54631714784465,3.6023269822301));
#38301=CARTESIAN_POINT('',(7.6,-3.21182691052252,3.56709516229149));
#38302=CARTESIAN_POINT('Ctrl Pts',(7.6,-3.21182691052252,3.56709516229149));
#38303=CARTESIAN_POINT('Ctrl Pts',(7.50357879858679,-3.34083471269687,3.58068353991731));
#38304=CARTESIAN_POINT('Ctrl Pts',(7.4,-3.47521783996191,3.59483809994421));
#38305=CARTESIAN_POINT('',(0.6,-3.21182691052252,3.56709516229149));
#38306=CARTESIAN_POINT('',(0.6,-3.21182691052252,3.56709516229149));
#38307=CARTESIAN_POINT('',(0.6,-3.54631714784465,3.6023269822301));
#38308=CARTESIAN_POINT('Origin',(0.6,-3.29546823631738,3.65998826547617));
#38309=CARTESIAN_POINT('',(0.6,-3.21182691052252,3.56709516229149));
#38310=CARTESIAN_POINT('Origin',(0.6,-3.21182691052252,3.56709516229149));
#38311=CARTESIAN_POINT('Ctrl Pts',(7.4,-3.21188602036704,3.83194313529973));
#38312=CARTESIAN_POINT('Ctrl Pts',(7.50357879858653,-3.2118558622831,3.69681661845911));
#38313=CARTESIAN_POINT('Ctrl Pts',(7.6,-3.21182691052252,3.5670951622915));
#38314=CARTESIAN_POINT('Origin',(0.6,-2.7198557158515,4.26092828911142));
#38315=CARTESIAN_POINT('',(7.6,-2.4,4.15692193816531));
#38316=CARTESIAN_POINT('Ctrl Pts',(7.6,-2.4,4.15692193816531));
#38317=CARTESIAN_POINT('Ctrl Pts',(7.50357879858686,-2.52336348960505,4.19703560741659));
#38318=CARTESIAN_POINT('Ctrl Pts',(7.4,-2.65186712461055,4.23882067955342));
#38319=CARTESIAN_POINT('',(0.6,-2.4,4.15692193816531));
#38320=CARTESIAN_POINT('',(0.6,-2.4,4.15692193816531));
#38321=CARTESIAN_POINT('',(0.6,-2.7198557158515,4.26092828911142));
#38322=CARTESIAN_POINT('Origin',(0.6,-2.4625,4.26517511363836));
#38323=CARTESIAN_POINT('',(0.6,-2.4,4.15692193816531));
#38324=CARTESIAN_POINT('Origin',(0.6,-2.4,4.15692193816531));
#38325=CARTESIAN_POINT('Ctrl Pts',(7.4,-2.3449928282748,4.41599463715025));
#38326=CARTESIAN_POINT('Ctrl Pts',(7.50357879858658,-2.37305771180802,4.28381468868878));
#38327=CARTESIAN_POINT('Ctrl Pts',(7.6,-2.4,4.15692193816531));
#38328=CARTESIAN_POINT('Origin',(0.6,-1.77452353775989,4.73330658355616));
#38329=CARTESIAN_POINT('',(7.6,-1.48328157299975,4.56507127821674));
#38330=CARTESIAN_POINT('Ctrl Pts',(7.6,-1.48328157299975,4.56507127821674));
#38331=CARTESIAN_POINT('Ctrl Pts',(7.50357879858684,-1.59560917357616,4.62995707926049));
#38332=CARTESIAN_POINT('Ctrl Pts',(7.4,-1.71261709084344,4.69754645534783));
#38333=CARTESIAN_POINT('',(0.6,-1.48328157299975,4.56507127821674));
#38334=CARTESIAN_POINT('',(0.6,-1.48328157299975,4.56507127821674));
#38335=CARTESIAN_POINT('',(0.6,-1.77452353775989,4.73330658355616));
#38336=CARTESIAN_POINT('Origin',(0.6,-1.52190869729662,4.68395334275363));
#38337=CARTESIAN_POINT('',(0.6,-1.48328157299975,4.56507127821674));
#38338=CARTESIAN_POINT('Origin',(0.6,-1.48328157299975,4.56507127821674));
#38339=CARTESIAN_POINT('Ctrl Pts',(7.4,-1.37561219706291,4.807045983064));
#38340=CARTESIAN_POINT('Ctrl Pts',(7.50357879858665,-1.43054555213267,4.6835895009992));
#38341=CARTESIAN_POINT('Ctrl Pts',(7.6,-1.48328157299975,4.56507127821674));
#38342=CARTESIAN_POINT('Origin',(0.6,-0.751636165959511,4.99881666737456));
#38343=CARTESIAN_POINT('',(7.6,-0.501736623684736,4.77370509776771));
#38344=CARTESIAN_POINT('Ctrl Pts',(7.6,-0.501736623684736,4.77370509776771));
#38345=CARTESIAN_POINT('Ctrl Pts',(7.5035787985868,-0.598119080079706,4.86052720974173));
#38346=CARTESIAN_POINT('Ctrl Pts',(7.4,-0.698517472157876,4.95096690971472));
#38347=CARTESIAN_POINT('',(0.6,-0.501736623684736,4.77370509776771));
#38348=CARTESIAN_POINT('',(0.6,-0.501736623684736,4.77370509776771));
#38349=CARTESIAN_POINT('',(0.6,-0.751636165959511,4.99881666737456));
#38350=CARTESIAN_POINT('Origin',(0.6,-0.514802681593193,4.89802033468875));
#38351=CARTESIAN_POINT('',(0.6,-0.501736623684736,4.77370509776771));
#38352=CARTESIAN_POINT('Origin',(0.6,-0.501736623684736,4.77370509776771));
#38353=CARTESIAN_POINT('Ctrl Pts',(7.4,-0.346110711919695,4.98800635275201));
#38354=CARTESIAN_POINT('Ctrl Pts',(7.50357879858677,-0.425511687310028,
4.87866897776002));
#38355=CARTESIAN_POINT('Ctrl Pts',(7.6,-0.501736623684736,4.77370509776771));
#38356=CARTESIAN_POINT('Origin',(0.6,0.30410131304379,5.045854475845));
#38357=CARTESIAN_POINT('',(7.6,0.501736623684738,4.77370509776771));
#38358=CARTESIAN_POINT('Ctrl Pts',(7.6,0.501736623684738,4.77370509776771));
#38359=CARTESIAN_POINT('Ctrl Pts',(7.50357879858681,0.425511687310058,4.87866897775998));
#38360=CARTESIAN_POINT('Ctrl Pts',(7.4,0.346110711919696,4.98800635275201));
#38361=CARTESIAN_POINT('',(0.6,0.501736623684738,4.77370509776771));
#38362=CARTESIAN_POINT('',(0.6,0.501736623684738,4.77370509776771));
#38363=CARTESIAN_POINT('',(0.6,0.30410131304379,5.045854475845));
#38364=CARTESIAN_POINT('Origin',(0.6,0.514802681593194,4.89802033468875));
#38365=CARTESIAN_POINT('',(0.6,0.501736623684738,4.77370509776771));
#38366=CARTESIAN_POINT('Origin',(0.6,0.501736623684738,4.77370509776771));
#38367=CARTESIAN_POINT('Ctrl Pts',(7.4,0.698517472157879,4.95096690971472));
#38368=CARTESIAN_POINT('Ctrl Pts',(7.50357879858674,0.598119080079767,4.86052720974178));
#38369=CARTESIAN_POINT('Ctrl Pts',(7.6,0.501736623684738,4.77370509776771));
#38370=CARTESIAN_POINT('Origin',(0.6,1.34654810542708,4.87236423102489));
#38371=CARTESIAN_POINT('',(7.6,1.48328157299975,4.56507127821674));
#38372=CARTESIAN_POINT('Ctrl Pts',(7.6,1.48328157299975,4.56507127821674));
#38373=CARTESIAN_POINT('Ctrl Pts',(7.50357879858677,1.43054555213273,4.68358950099906));
#38374=CARTESIAN_POINT('Ctrl Pts',(7.4,1.37561219706292,4.807045983064));
#38375=CARTESIAN_POINT('',(0.6,1.48328157299975,4.56507127821674));
#38376=CARTESIAN_POINT('',(0.6,1.48328157299975,4.56507127821674));
#38377=CARTESIAN_POINT('',(0.6,1.34654810542708,4.87236423102489));
#38378=CARTESIAN_POINT('Origin',(0.6,1.52190869729662,4.68395334275363));
#38379=CARTESIAN_POINT('',(0.6,1.48328157299975,4.56507127821674));
#38380=CARTESIAN_POINT('Origin',(0.6,1.48328157299975,4.56507127821674));
#38381=CARTESIAN_POINT('Ctrl Pts',(7.4,1.71261709084344,4.69754645534783));
#38382=CARTESIAN_POINT('Ctrl Pts',(7.50357879858672,1.59560917357629,4.62995707926056));
#38383=CARTESIAN_POINT('Ctrl Pts',(7.6,1.48328157299975,4.56507127821674));
#38384=CARTESIAN_POINT('Origin',(0.6,2.3301442841485,4.48592828911142));
#38385=CARTESIAN_POINT('',(7.6,2.4,4.15692193816531));
#38386=CARTESIAN_POINT('Ctrl Pts',(7.6,2.4,4.15692193816531));
#38387=CARTESIAN_POINT('Ctrl Pts',(7.50357879858657,2.37305771180801,4.28381468868879));
#38388=CARTESIAN_POINT('Ctrl Pts',(7.4,2.3449928282748,4.41599463715025));
#38389=CARTESIAN_POINT('',(0.6,2.4,4.15692193816531));
#38390=CARTESIAN_POINT('',(0.6,2.4,4.15692193816531));
#38391=CARTESIAN_POINT('',(0.6,2.3301442841485,4.48592828911142));
#38392=CARTESIAN_POINT('Origin',(0.6,2.4625,4.26517511363836));
#38393=CARTESIAN_POINT('',(0.6,2.4,4.15692193816531));
#38394=CARTESIAN_POINT('Origin',(0.6,2.4,4.15692193816531));
#38395=CARTESIAN_POINT('Ctrl Pts',(7.4,2.65186712461056,4.23882067955342));
#38396=CARTESIAN_POINT('Ctrl Pts',(7.50357879858673,2.52336348960521,4.19703560741664));
#38397=CARTESIAN_POINT('Ctrl Pts',(7.6,2.4,4.15692193816531));
#38398=CARTESIAN_POINT('Origin',(0.6,3.21190197637982,3.90343575509158));
#38399=CARTESIAN_POINT('',(7.6,3.21182691052252,3.56709516229149));
#38400=CARTESIAN_POINT('Ctrl Pts',(7.6,3.21182691052252,3.56709516229149));
#38401=CARTESIAN_POINT('Ctrl Pts',(7.5035787985867,3.2118558622831,3.69681661845887));
#38402=CARTESIAN_POINT('Ctrl Pts',(7.4,3.21188602036705,3.83194313529973));
#38403=CARTESIAN_POINT('',(0.6,3.21182691052252,3.56709516229149));
#38404=CARTESIAN_POINT('',(0.6,3.21182691052252,3.56709516229149));
#38405=CARTESIAN_POINT('',(0.6,3.21190197637982,3.90343575509158));
#38406=CARTESIAN_POINT('Origin',(0.6,3.29546823631738,3.65998826547617));
#38407=CARTESIAN_POINT('',(0.6,3.21182691052252,3.56709516229149));
#38408=CARTESIAN_POINT('Origin',(0.6,3.21182691052252,3.56709516229149));
#38409=CARTESIAN_POINT('Ctrl Pts',(7.4,3.47521783996191,3.59483809994421));
#38410=CARTESIAN_POINT('Ctrl Pts',(7.50357879858682,3.34083471269684,3.58068353991731));
#38411=CARTESIAN_POINT('Ctrl Pts',(7.6,3.21182691052252,3.56709516229149));
#38412=CARTESIAN_POINT('Origin',(0.6,3.95328413982768,3.15034434781135));
#38413=CARTESIAN_POINT('',(7.6,3.88328157299975,2.82136921100387));
#38414=CARTESIAN_POINT('Ctrl Pts',(7.6,3.88328157299975,2.82136921100387));
#38415=CARTESIAN_POINT('Ctrl Pts',(7.50357879858661,3.91028049938203,2.94824992270832));
#38416=CARTESIAN_POINT('Ctrl Pts',(7.4,3.93840438103015,3.08041733073337));
#38417=CARTESIAN_POINT('',(0.6,3.88328157299975,2.82136921100387));
#38418=CARTESIAN_POINT('',(0.6,3.88328157299975,2.82136921100387));
#38419=CARTESIAN_POINT('',(0.6,3.95328413982768,3.15034434781135));
#38420=CARTESIAN_POINT('Origin',(0.6,3.98440869729662,2.89484236754043));
#38421=CARTESIAN_POINT('',(0.6,3.88328157299975,2.82136921100387));
#38422=CARTESIAN_POINT('Origin',(0.6,3.88328157299975,2.82136921100387));
#38423=CARTESIAN_POINT('Ctrl Pts',(7.4,4.14668485976156,2.79374384542038));
#38424=CARTESIAN_POINT('Ctrl Pts',(7.50357879858679,4.01229542774018,2.80783841969768));
#38425=CARTESIAN_POINT('Ctrl Pts',(7.6,3.88328157299975,2.82136921100387));
#38426=CARTESIAN_POINT('Origin',(0.6,4.52188881640308,2.25956777550238));
#38427=CARTESIAN_POINT('',(7.6,4.38501819668448,1.95233588676384));
#38428=CARTESIAN_POINT('Ctrl Pts',(7.6,4.38501819668449,1.95233588676384));
#38429=CARTESIAN_POINT('Ctrl Pts',(7.50357879858667,4.4378071150503,2.07083055806246));
#38430=CARTESIAN_POINT('Ctrl Pts',(7.4,4.49279557168126,2.19426250733163));
#38431=CARTESIAN_POINT('',(0.6,4.38501819668448,1.95233588676384));
#38432=CARTESIAN_POINT('',(0.6,4.38501819668448,1.95233588676384));
#38433=CARTESIAN_POINT('',(0.6,4.52188881640308,2.25956777550238));
#38434=CARTESIAN_POINT('Origin',(0.6,4.49921137888981,2.00317796714832));
#38435=CARTESIAN_POINT('',(0.6,4.38501819668448,1.95233588676384));
#38436=CARTESIAN_POINT('Origin',(0.6,4.38501819668448,1.95233588676384));
#38437=CARTESIAN_POINT('Ctrl Pts',(7.4,4.63692185318803,1.87054957898135));
#38438=CARTESIAN_POINT('Ctrl Pts',(7.50357879858679,4.5083995794617,1.91227728703365));
#38439=CARTESIAN_POINT('Ctrl Pts',(7.6,4.38501819668448,1.95233588676384));
#38440=CARTESIAN_POINT('Origin',(0.6,4.89286525327172,1.27003724879479));
#38441=CARTESIAN_POINT('',(7.6,4.69510848352227,0.997976115925245));
#38442=CARTESIAN_POINT('Ctrl Pts',(7.6,4.69510848352227,0.997976115925245));
#38443=CARTESIAN_POINT('Ctrl Pts',(7.50357879858677,4.77138026482964,1.10290596108175));
#38444=CARTESIAN_POINT('Ctrl Pts',(7.4,4.85083003702482,1.21220788311979));
#38445=CARTESIAN_POINT('',(0.6,4.69510848352227,0.997976115925245));
#38446=CARTESIAN_POINT('',(0.6,4.69510848352227,0.997976115925245));
#38447=CARTESIAN_POINT('',(0.6,4.89286525327172,1.27003724879479));
#38448=CARTESIAN_POINT('Origin',(0.6,4.81737693361399,1.02396507727746));
#38449=CARTESIAN_POINT('',(0.6,4.69510848352227,0.997976115925245));
#38450=CARTESIAN_POINT('Origin',(0.6,4.69510848352227,0.997976115925245));
#38451=CARTESIAN_POINT('Ctrl Pts',(7.4,4.92450311121048,0.865603320048098));
#38452=CARTESIAN_POINT('Ctrl Pts',(7.50357879858674,4.80746503585938,0.933140460801728));
#38453=CARTESIAN_POINT('Ctrl Pts',(7.6,4.69510848352227,0.997976115925244));
#38454=CARTESIAN_POINT('Origin',(0.6,5.05,0.225));
#38455=CARTESIAN_POINT('',(7.6,4.8,0.));
#38456=CARTESIAN_POINT('Ctrl Pts',(7.6,4.8,5.66922395553271E-16));
#38457=CARTESIAN_POINT('Ctrl Pts',(7.50357879858671,4.89642120141329,0.0867790812719613));
#38458=CARTESIAN_POINT('Ctrl Pts',(7.4,4.99685995288536,0.177173957596824));
#38459=CARTESIAN_POINT('',(0.6,4.8,0.));
#38460=CARTESIAN_POINT('',(0.6,4.8,0.));
#38461=CARTESIAN_POINT('',(0.6,5.05,0.225));
#38462=CARTESIAN_POINT('Origin',(0.6,4.925,0.));
#38463=CARTESIAN_POINT('',(0.6,4.8,0.));
#38464=CARTESIAN_POINT('Origin',(0.6,4.8,0.));
#38465=CARTESIAN_POINT('Ctrl Pts',(7.4,4.99685995288536,-0.177173957596825));
#38466=CARTESIAN_POINT('Ctrl Pts',(7.5035787985867,4.8964212014133,-0.0867790812719661));
#38467=CARTESIAN_POINT('Ctrl Pts',(7.6,4.8,-5.66922395553271E-16));
#38468=CARTESIAN_POINT('Origin',(-12.,2.1,0.));
#38469=CARTESIAN_POINT('',(-12.,-2.1,-2.57175827820944E-16));
#38470=CARTESIAN_POINT('Origin',(-12.,0.,0.));
#38471=CARTESIAN_POINT('Origin',(-11.8,0.,0.));
#38472=CARTESIAN_POINT('',(-11.8,-2.3,-2.81668763803891E-16));
#38473=CARTESIAN_POINT('Origin',(-5.8,0.,0.));
#38474=CARTESIAN_POINT('Origin',(0.,0.,0.));
#38475=CARTESIAN_POINT('Origin',(0.,4.5,0.));
#38476=CARTESIAN_POINT('',(2.08166817117217E-16,-4.5,-5.51091059616309E-16));
#38477=CARTESIAN_POINT('Origin',(0.,0.,0.));
#38478=CARTESIAN_POINT('Origin',(0.25,0.,0.));
#38479=CARTESIAN_POINT('',(0.25,-4.75,-5.81707229594993E-16));
#38480=CARTESIAN_POINT('Origin',(7.7,0.,0.));
#38481=CARTESIAN_POINT('',(8.,-4.4,-5.38844591624835E-16));
#38482=CARTESIAN_POINT('Origin',(8.,0.,0.));
#38483=CARTESIAN_POINT('',(7.7,-4.7,-5.75583995599256E-16));
#38484=CARTESIAN_POINT('Origin',(8.,0.,0.));
#38513=UNCERTAINTY_MEASURE_WITH_UNIT(LENGTH_MEASURE(0.01),#38529,
'DISTANCE_ACCURACY_VALUE',
'Maximum model space distance between geometric entities at asserted c
onnectivities');
#38514=UNCERTAINTY_MEASURE_WITH_UNIT(LENGTH_MEASURE(0.01),#38529,
'DISTANCE_ACCURACY_VALUE',
'Maximum model space distance between geometric entities at asserted c
onnectivities');
#38527=(
GEOMETRIC_REPRESENTATION_CONTEXT(3)
GLOBAL_UNCERTAINTY_ASSIGNED_CONTEXT((#38513))
GLOBAL_UNIT_ASSIGNED_CONTEXT((#38529,#38531,#38532))
REPRESENTATION_CONTEXT('','3D')
);
#38528=(
GEOMETRIC_REPRESENTATION_CONTEXT(3)
GLOBAL_UNCERTAINTY_ASSIGNED_CONTEXT((#38514))
GLOBAL_UNIT_ASSIGNED_CONTEXT((#38529,#38531,#38532))
REPRESENTATION_CONTEXT('','3D')
);
#38529=(
LENGTH_UNIT()
NAMED_UNIT(*)
SI_UNIT(.MILLI.,.METRE.)
);
#38531=(
NAMED_UNIT(*)
PLANE_ANGLE_UNIT()
SI_UNIT($,.RADIAN.)
);
#38532=(
NAMED_UNIT(*)
SI_UNIT($,.STERADIAN.)
SOLID_ANGLE_UNIT()
);
#38545=SHAPE_DEFINITION_REPRESENTATION(#38558,#38587);
#38558=PRODUCT_DEFINITION_SHAPE('',$,#38601);
#38587=SHAPE_REPRESENTATION('',(#18808),#38527);
#38588=PRODUCT_DEFINITION_CONTEXT('part definition',#38629,'design');
#38601=PRODUCT_DEFINITION('2026-10-20-13-39-12-626',
'12_Dovetail_Lock_Thumb_Screw_M5',#38614,#38588);
#38614=PRODUCT_DEFINITION_FORMATION('',$,#38643);
#38629=APPLICATION_CONTEXT(
'Core Data for Automotive Mechanical Design Process');
#38630=PRODUCT_CONTEXT('part definition',#38629,'mechanical');
#38643=PRODUCT('2026-10-20-13-39-12-626',
'12_Dovetail_Lock_Thumb_Screw_M5',$,(#38630));
#38707=COLOUR_RGB('Black',0.12,0.14,0.17);
#38708=FILL_AREA_STYLE_COLOUR('',#38707);
#38709=FILL_AREA_STYLE('',(#38708));
#38710=SURFACE_STYLE_FILL_AREA(#38709);
#38711=SURFACE_SIDE_STYLE('',(#38710));
#38712=SURFACE_STYLE_USAGE(.BOTH.,#38711);
#38713=PRESENTATION_STYLE_ASSIGNMENT((#38712));
ENDSEC;
END-ISO-10303-21;
